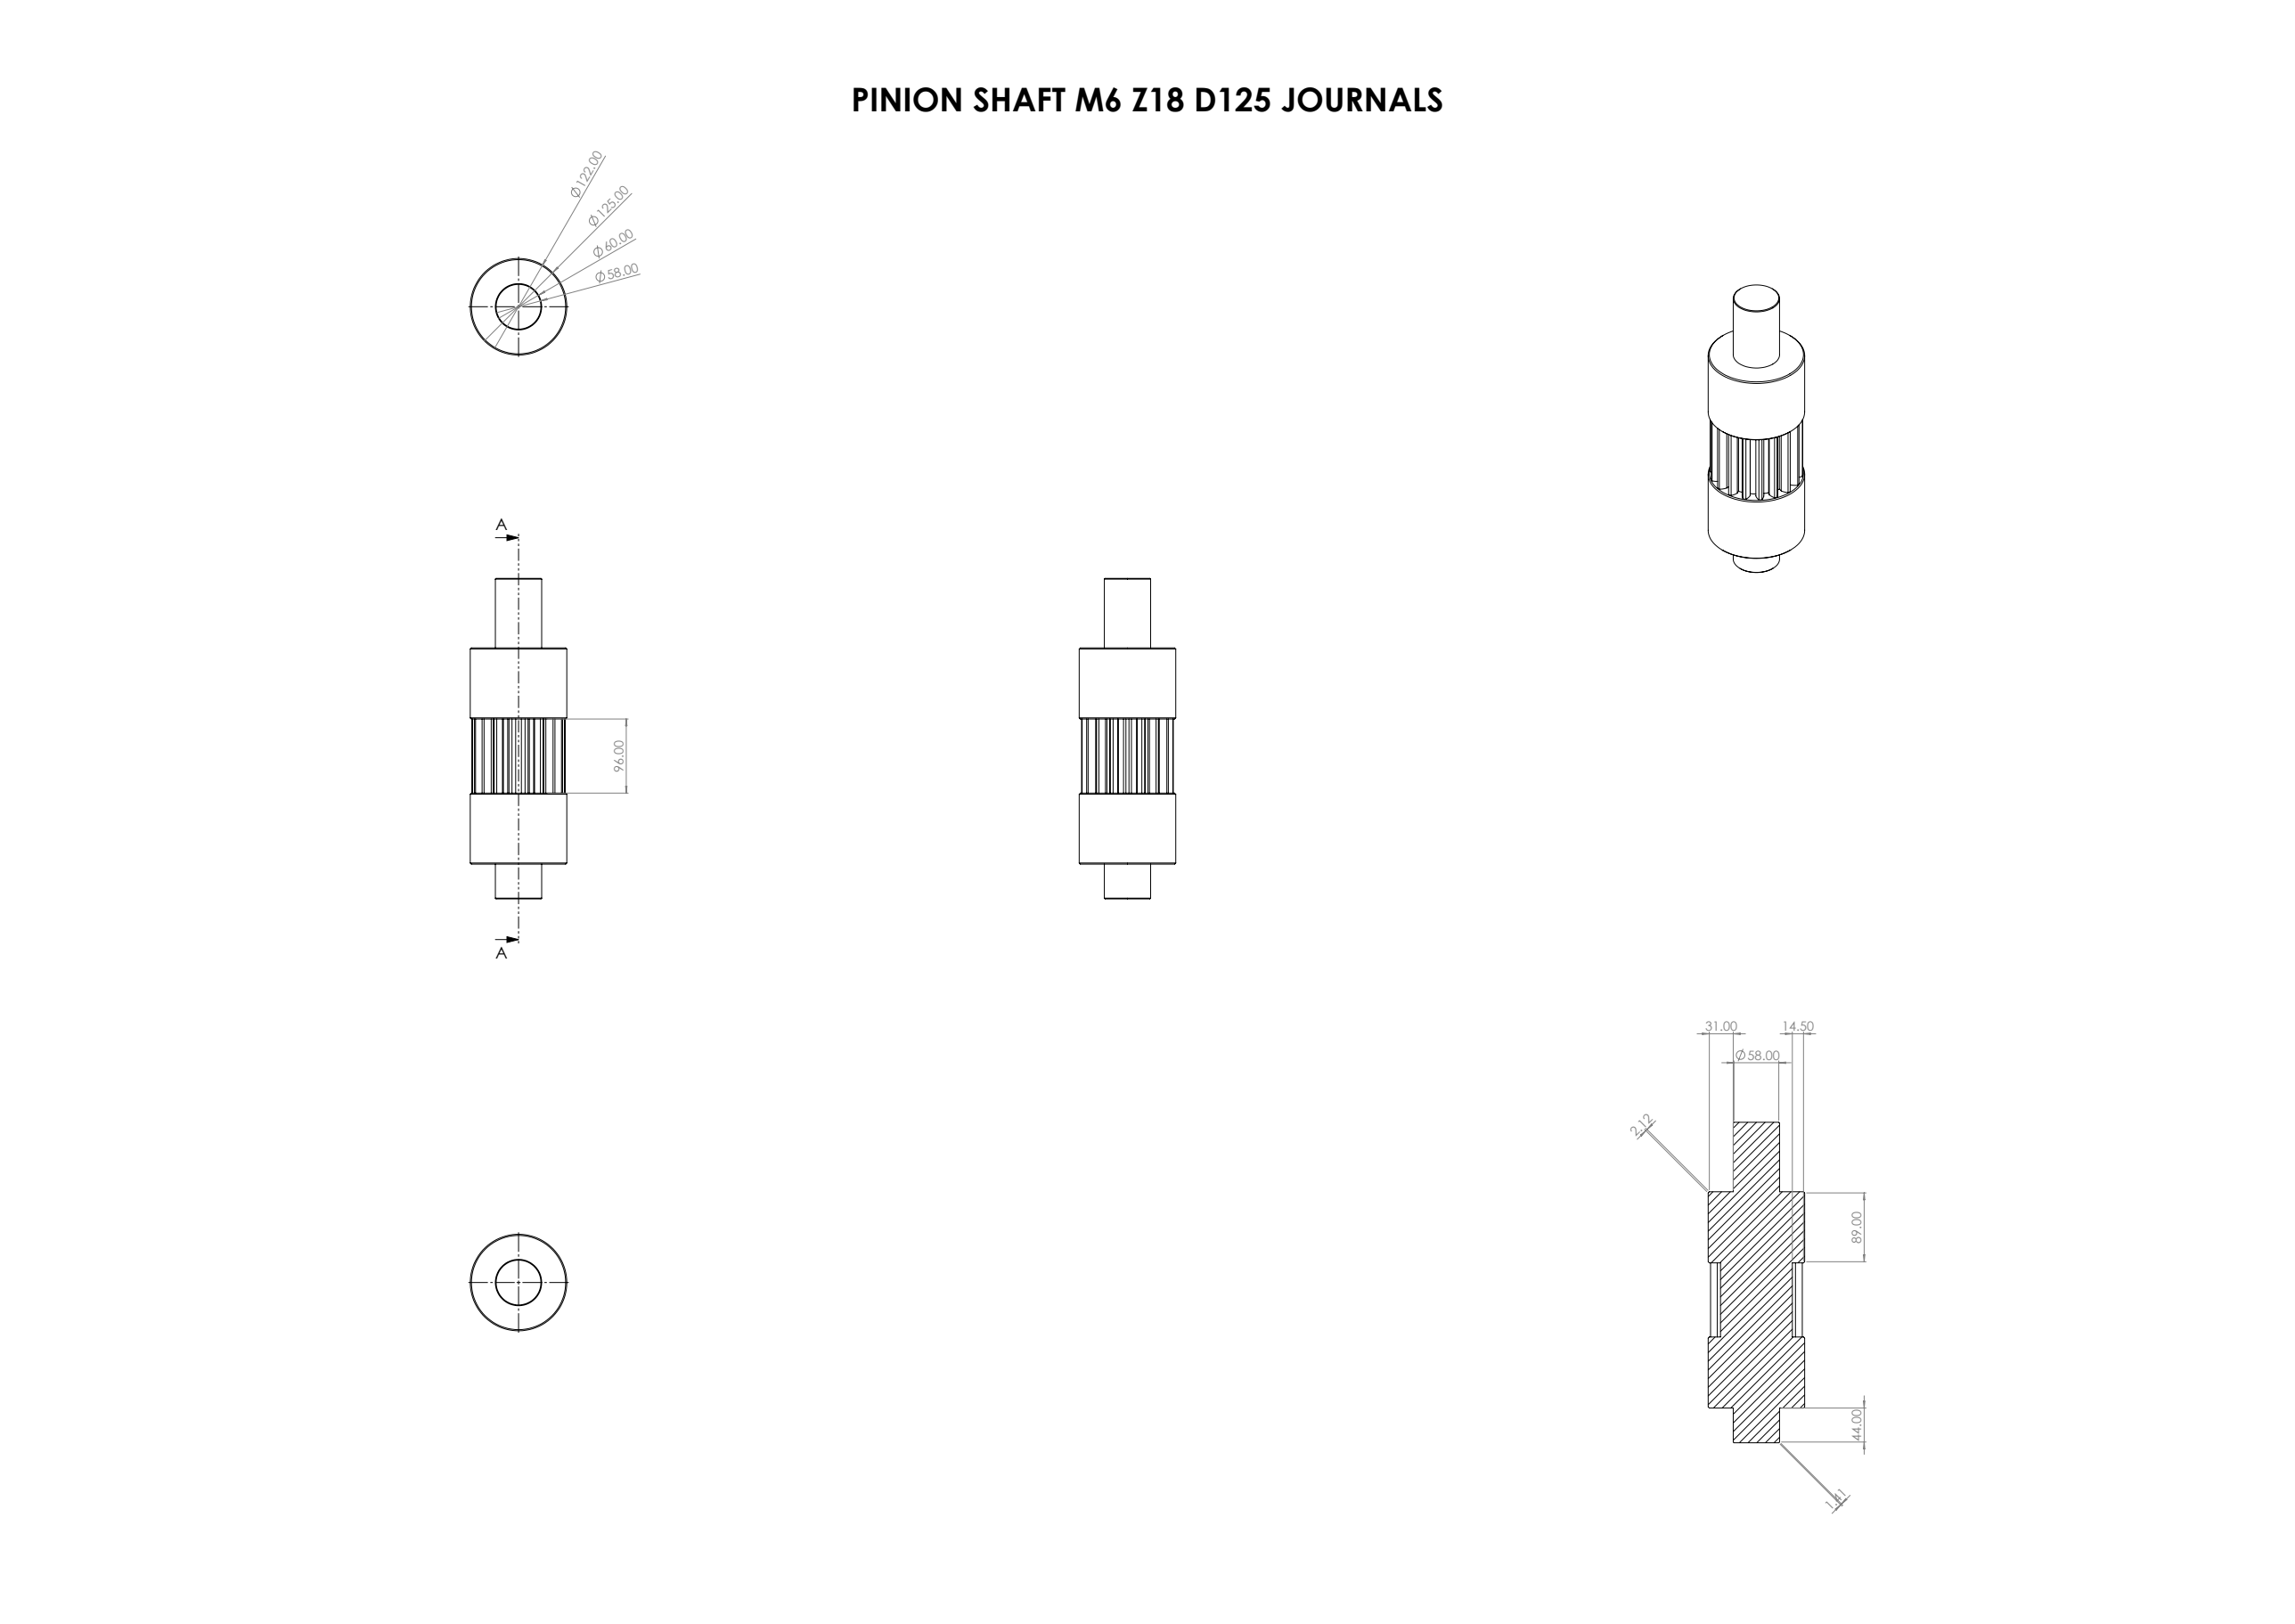
ISO-10303-21;
HEADER;
/* Generated by software containing ST-Developer
 * from STEP Tools, Inc. (www.steptools.com) 
 */

FILE_DESCRIPTION(
/* description */ (''),
/* implementation_level */ '2;1');

FILE_NAME(
/* name */ '03_Pinion_Shaft_m6_z18_D125_Journals.step',
/* time_stamp */ '2026-10-19T23:58:09-07:00',
/* author */ (''),
/* organization */ (''),
/* preprocessor_version */ 'ST-DEVELOPER v20.2',
/* originating_system */ 'Autodesk Translation Framework v15.15.0.0',
/* authorisation */ '');

FILE_SCHEMA (('AP203_CONFIGURATION_CONTROLLED_3D_DESIGN_OF_MECHANICAL_PARTS_AND_ASSEMBLIES_MIM_LF { 1 0 10303 203 3 1 4 }',
'AUTOMOTIVE_DESIGN { 1 0 10303 214 3 1 1 }','INTEGRATED_CNC_SCHEMA','MODEL_BASED_INTEGRATED_MANUFACTURING_SCHEMA',
'PROCESS_PLANNING_SCHEMA','AP242_MANAGED_MODEL_BASED_3D_ENGINEERING_MIM_LF { 1 0 10303 442 3 1 4 }'));
ENDSEC;

DATA;
#10=MECHANICAL_DESIGN_GEOMETRIC_PRESENTATION_REPRESENTATION('',(#407),#70757);
#377=SHAPE_REPRESENTATION_RELATIONSHIP('SRR','None',#70818,#392);
#392=ADVANCED_BREP_SHAPE_REPRESENTATION('',(#467),#70742);
#407=STYLED_ITEM('',(#71047),#467);
#467=MANIFOLD_SOLID_BREP('Pinion shaft',#26872);
#482=(
BOUNDED_SURFACE()
B_SPLINE_SURFACE(5,1,((#37442,#37443),(#37444,#37445),(#37446,#37447),(#37448,
#37449),(#37450,#37451),(#37452,#37453),(#37454,#37455),(#37456,#37457),
(#37458,#37459),(#37460,#37461),(#37462,#37463),(#37464,#37465),(#37466,
#37467),(#37468,#37469),(#37470,#37471),(#37472,#37473),(#37474,#37475),
(#37476,#37477),(#37478,#37479),(#37480,#37481),(#37482,#37483),(#37484,
#37485),(#37486,#37487),(#37488,#37489),(#37490,#37491),(#37492,#37493),
(#37494,#37495),(#37496,#37497),(#37498,#37499),(#37500,#37501),(#37502,
#37503),(#37504,#37505),(#37506,#37507),(#37508,#37509),(#37510,#37511)),
 .UNSPECIFIED.,.F.,.F.,.F.)
B_SPLINE_SURFACE_WITH_KNOTS((6,1,1,1,1,1,1,1,1,1,1,1,1,1,1,1,1,1,1,1,1,
1,1,1,1,1,1,1,1,1,6),(2,2),(-1.,-0.966666666666667,-0.933333333333333,-0.9,
-0.866666666666667,-0.833333333333333,-0.8,-0.766666666666667,-0.733333333333333,
-0.7,-0.666666666666667,-0.633333333333333,-0.6,-0.566666666666667,-0.533333333333333,
-0.5,-0.466666666666667,-0.433333333333333,-0.4,-0.366666666666667,-0.333333333333333,
-0.3,-0.266666666666667,-0.233333333333333,-0.2,-0.166666666666667,-0.133333333333333,
-0.1,-0.0666666666666667,-0.0333333333333333,0.),(-5.,5.),.UNSPECIFIED.)
GEOMETRIC_REPRESENTATION_ITEM()
RATIONAL_B_SPLINE_SURFACE(((1.,1.),(1.,1.),(1.,1.),(1.,1.),(1.,1.),(1.,
1.),(1.,1.),(1.,1.),(1.,1.),(1.,1.),(1.,1.),(1.,1.),(1.,1.),(1.,1.),(1.,
1.),(1.,1.),(1.,1.),(1.,1.),(1.,1.),(1.,1.),(1.,1.),(1.,1.),(1.,1.),(1.,
1.),(1.,1.),(1.,1.),(1.,1.),(1.,1.),(1.,1.),(1.,1.),(1.,1.),(1.,1.),(1.,
1.),(1.,1.),(1.,1.)))
REPRESENTATION_ITEM('')
SURFACE()
);
#483=(
BOUNDED_SURFACE()
B_SPLINE_SURFACE(5,1,((#37523,#37524),(#37525,#37526),(#37527,#37528),(#37529,
#37530),(#37531,#37532),(#37533,#37534),(#37535,#37536),(#37537,#37538),
(#37539,#37540),(#37541,#37542),(#37543,#37544),(#37545,#37546),(#37547,
#37548),(#37549,#37550),(#37551,#37552),(#37553,#37554),(#37555,#37556),
(#37557,#37558),(#37559,#37560),(#37561,#37562),(#37563,#37564),(#37565,
#37566),(#37567,#37568),(#37569,#37570),(#37571,#37572),(#37573,#37574),
(#37575,#37576),(#37577,#37578),(#37579,#37580),(#37581,#37582),(#37583,
#37584),(#37585,#37586),(#37587,#37588),(#37589,#37590),(#37591,#37592)),
 .UNSPECIFIED.,.F.,.F.,.F.)
B_SPLINE_SURFACE_WITH_KNOTS((6,1,1,1,1,1,1,1,1,1,1,1,1,1,1,1,1,1,1,1,1,
1,1,1,1,1,1,1,1,1,6),(2,2),(0.,0.0333333333333333,0.0666666666666667,0.1,
0.133333333333333,0.166666666666667,0.2,0.233333333333333,0.266666666666667,
0.3,0.333333333333333,0.366666666666667,0.4,0.433333333333333,0.466666666666667,
0.5,0.533333333333333,0.566666666666667,0.6,0.633333333333333,0.666666666666667,
0.7,0.733333333333333,0.766666666666667,0.8,0.833333333333333,0.866666666666667,
0.9,0.933333333333333,0.966666666666667,1.),(-5.,5.),.UNSPECIFIED.)
GEOMETRIC_REPRESENTATION_ITEM()
RATIONAL_B_SPLINE_SURFACE(((1.,1.),(1.,1.),(1.,1.),(1.,1.),(1.,1.),(1.,
1.),(1.,1.),(1.,1.),(1.,1.),(1.,1.),(1.,1.),(1.,1.),(1.,1.),(1.,1.),(1.,
1.),(1.,1.),(1.,1.),(1.,1.),(1.,1.),(1.,1.),(1.,1.),(1.,1.),(1.,1.),(1.,
1.),(1.,1.),(1.,1.),(1.,1.),(1.,1.),(1.,1.),(1.,1.),(1.,1.),(1.,1.),(1.,
1.),(1.,1.),(1.,1.)))
REPRESENTATION_ITEM('')
SURFACE()
);
#484=(
BOUNDED_SURFACE()
B_SPLINE_SURFACE(5,1,((#37601,#37602),(#37603,#37604),(#37605,#37606),(#37607,
#37608),(#37609,#37610),(#37611,#37612),(#37613,#37614),(#37615,#37616),
(#37617,#37618),(#37619,#37620),(#37621,#37622),(#37623,#37624),(#37625,
#37626),(#37627,#37628),(#37629,#37630),(#37631,#37632),(#37633,#37634),
(#37635,#37636),(#37637,#37638),(#37639,#37640),(#37641,#37642),(#37643,
#37644),(#37645,#37646),(#37647,#37648),(#37649,#37650),(#37651,#37652),
(#37653,#37654),(#37655,#37656),(#37657,#37658),(#37659,#37660),(#37661,
#37662),(#37663,#37664),(#37665,#37666),(#37667,#37668),(#37669,#37670)),
 .UNSPECIFIED.,.F.,.F.,.F.)
B_SPLINE_SURFACE_WITH_KNOTS((6,1,1,1,1,1,1,1,1,1,1,1,1,1,1,1,1,1,1,1,1,
1,1,1,1,1,1,1,1,1,6),(2,2),(-1.,-0.966666666666667,-0.933333333333333,-0.9,
-0.866666666666667,-0.833333333333333,-0.8,-0.766666666666667,-0.733333333333333,
-0.7,-0.666666666666667,-0.633333333333333,-0.6,-0.566666666666667,-0.533333333333333,
-0.5,-0.466666666666667,-0.433333333333333,-0.4,-0.366666666666667,-0.333333333333333,
-0.3,-0.266666666666667,-0.233333333333333,-0.2,-0.166666666666667,-0.133333333333333,
-0.1,-0.0666666666666667,-0.0333333333333333,0.),(-5.,5.),.UNSPECIFIED.)
GEOMETRIC_REPRESENTATION_ITEM()
RATIONAL_B_SPLINE_SURFACE(((1.,1.),(1.,1.),(1.,1.),(1.,1.),(1.,1.),(1.,
1.),(1.,1.),(1.,1.),(1.,1.),(1.,1.),(1.,1.),(1.,1.),(1.,1.),(1.,1.),(1.,
1.),(1.,1.),(1.,1.),(1.,1.),(1.,1.),(1.,1.),(1.,1.),(1.,1.),(1.,1.),(1.,
1.),(1.,1.),(1.,1.),(1.,1.),(1.,1.),(1.,1.),(1.,1.),(1.,1.),(1.,1.),(1.,
1.),(1.,1.),(1.,1.)))
REPRESENTATION_ITEM('')
SURFACE()
);
#485=(
BOUNDED_SURFACE()
B_SPLINE_SURFACE(5,1,((#37682,#37683),(#37684,#37685),(#37686,#37687),(#37688,
#37689),(#37690,#37691),(#37692,#37693),(#37694,#37695),(#37696,#37697),
(#37698,#37699),(#37700,#37701),(#37702,#37703),(#37704,#37705),(#37706,
#37707),(#37708,#37709),(#37710,#37711),(#37712,#37713),(#37714,#37715),
(#37716,#37717),(#37718,#37719),(#37720,#37721),(#37722,#37723),(#37724,
#37725),(#37726,#37727),(#37728,#37729),(#37730,#37731),(#37732,#37733),
(#37734,#37735),(#37736,#37737),(#37738,#37739),(#37740,#37741),(#37742,
#37743),(#37744,#37745),(#37746,#37747),(#37748,#37749),(#37750,#37751)),
 .UNSPECIFIED.,.F.,.F.,.F.)
B_SPLINE_SURFACE_WITH_KNOTS((6,1,1,1,1,1,1,1,1,1,1,1,1,1,1,1,1,1,1,1,1,
1,1,1,1,1,1,1,1,1,6),(2,2),(0.,0.0333333333333333,0.0666666666666667,0.1,
0.133333333333333,0.166666666666667,0.2,0.233333333333333,0.266666666666667,
0.3,0.333333333333333,0.366666666666667,0.4,0.433333333333333,0.466666666666667,
0.5,0.533333333333333,0.566666666666667,0.6,0.633333333333333,0.666666666666667,
0.7,0.733333333333333,0.766666666666667,0.8,0.833333333333333,0.866666666666667,
0.9,0.933333333333333,0.966666666666667,1.),(-5.,5.),.UNSPECIFIED.)
GEOMETRIC_REPRESENTATION_ITEM()
RATIONAL_B_SPLINE_SURFACE(((1.,1.),(1.,1.),(1.,1.),(1.,1.),(1.,1.),(1.,
1.),(1.,1.),(1.,1.),(1.,1.),(1.,1.),(1.,1.),(1.,1.),(1.,1.),(1.,1.),(1.,
1.),(1.,1.),(1.,1.),(1.,1.),(1.,1.),(1.,1.),(1.,1.),(1.,1.),(1.,1.),(1.,
1.),(1.,1.),(1.,1.),(1.,1.),(1.,1.),(1.,1.),(1.,1.),(1.,1.),(1.,1.),(1.,
1.),(1.,1.),(1.,1.)))
REPRESENTATION_ITEM('')
SURFACE()
);
#486=(
BOUNDED_SURFACE()
B_SPLINE_SURFACE(5,1,((#37760,#37761),(#37762,#37763),(#37764,#37765),(#37766,
#37767),(#37768,#37769),(#37770,#37771),(#37772,#37773),(#37774,#37775),
(#37776,#37777),(#37778,#37779),(#37780,#37781),(#37782,#37783),(#37784,
#37785),(#37786,#37787),(#37788,#37789),(#37790,#37791),(#37792,#37793),
(#37794,#37795),(#37796,#37797),(#37798,#37799),(#37800,#37801),(#37802,
#37803),(#37804,#37805),(#37806,#37807),(#37808,#37809),(#37810,#37811),
(#37812,#37813),(#37814,#37815),(#37816,#37817),(#37818,#37819),(#37820,
#37821),(#37822,#37823),(#37824,#37825),(#37826,#37827),(#37828,#37829)),
 .UNSPECIFIED.,.F.,.F.,.F.)
B_SPLINE_SURFACE_WITH_KNOTS((6,1,1,1,1,1,1,1,1,1,1,1,1,1,1,1,1,1,1,1,1,
1,1,1,1,1,1,1,1,1,6),(2,2),(-1.,-0.966666666666667,-0.933333333333333,-0.9,
-0.866666666666667,-0.833333333333333,-0.8,-0.766666666666667,-0.733333333333333,
-0.7,-0.666666666666667,-0.633333333333333,-0.6,-0.566666666666667,-0.533333333333333,
-0.5,-0.466666666666667,-0.433333333333333,-0.4,-0.366666666666667,-0.333333333333333,
-0.3,-0.266666666666667,-0.233333333333333,-0.2,-0.166666666666667,-0.133333333333333,
-0.1,-0.0666666666666667,-0.0333333333333333,0.),(-5.,5.),.UNSPECIFIED.)
GEOMETRIC_REPRESENTATION_ITEM()
RATIONAL_B_SPLINE_SURFACE(((1.,1.),(1.,1.),(1.,1.),(1.,1.),(1.,1.),(1.,
1.),(1.,1.),(1.,1.),(1.,1.),(1.,1.),(1.,1.),(1.,1.),(1.,1.),(1.,1.),(1.,
1.),(1.,1.),(1.,1.),(1.,1.),(1.,1.),(1.,1.),(1.,1.),(1.,1.),(1.,1.),(1.,
1.),(1.,1.),(1.,1.),(1.,1.),(1.,1.),(1.,1.),(1.,1.),(1.,1.),(1.,1.),(1.,
1.),(1.,1.),(1.,1.)))
REPRESENTATION_ITEM('')
SURFACE()
);
#487=(
BOUNDED_SURFACE()
B_SPLINE_SURFACE(5,1,((#37841,#37842),(#37843,#37844),(#37845,#37846),(#37847,
#37848),(#37849,#37850),(#37851,#37852),(#37853,#37854),(#37855,#37856),
(#37857,#37858),(#37859,#37860),(#37861,#37862),(#37863,#37864),(#37865,
#37866),(#37867,#37868),(#37869,#37870),(#37871,#37872),(#37873,#37874),
(#37875,#37876),(#37877,#37878),(#37879,#37880),(#37881,#37882),(#37883,
#37884),(#37885,#37886),(#37887,#37888),(#37889,#37890),(#37891,#37892),
(#37893,#37894),(#37895,#37896),(#37897,#37898),(#37899,#37900),(#37901,
#37902),(#37903,#37904),(#37905,#37906),(#37907,#37908),(#37909,#37910)),
 .UNSPECIFIED.,.F.,.F.,.F.)
B_SPLINE_SURFACE_WITH_KNOTS((6,1,1,1,1,1,1,1,1,1,1,1,1,1,1,1,1,1,1,1,1,
1,1,1,1,1,1,1,1,1,6),(2,2),(0.,0.0333333333333333,0.0666666666666667,0.1,
0.133333333333333,0.166666666666667,0.2,0.233333333333333,0.266666666666667,
0.3,0.333333333333333,0.366666666666667,0.4,0.433333333333333,0.466666666666667,
0.5,0.533333333333333,0.566666666666667,0.6,0.633333333333333,0.666666666666667,
0.7,0.733333333333333,0.766666666666667,0.8,0.833333333333333,0.866666666666667,
0.9,0.933333333333333,0.966666666666667,1.),(-5.,5.),.UNSPECIFIED.)
GEOMETRIC_REPRESENTATION_ITEM()
RATIONAL_B_SPLINE_SURFACE(((1.,1.),(1.,1.),(1.,1.),(1.,1.),(1.,1.),(1.,
1.),(1.,1.),(1.,1.),(1.,1.),(1.,1.),(1.,1.),(1.,1.),(1.,1.),(1.,1.),(1.,
1.),(1.,1.),(1.,1.),(1.,1.),(1.,1.),(1.,1.),(1.,1.),(1.,1.),(1.,1.),(1.,
1.),(1.,1.),(1.,1.),(1.,1.),(1.,1.),(1.,1.),(1.,1.),(1.,1.),(1.,1.),(1.,
1.),(1.,1.),(1.,1.)))
REPRESENTATION_ITEM('')
SURFACE()
);
#488=(
BOUNDED_SURFACE()
B_SPLINE_SURFACE(5,1,((#37919,#37920),(#37921,#37922),(#37923,#37924),(#37925,
#37926),(#37927,#37928),(#37929,#37930),(#37931,#37932),(#37933,#37934),
(#37935,#37936),(#37937,#37938),(#37939,#37940),(#37941,#37942),(#37943,
#37944),(#37945,#37946),(#37947,#37948),(#37949,#37950),(#37951,#37952),
(#37953,#37954),(#37955,#37956),(#37957,#37958),(#37959,#37960),(#37961,
#37962),(#37963,#37964),(#37965,#37966),(#37967,#37968),(#37969,#37970),
(#37971,#37972),(#37973,#37974),(#37975,#37976),(#37977,#37978),(#37979,
#37980),(#37981,#37982),(#37983,#37984),(#37985,#37986),(#37987,#37988)),
 .UNSPECIFIED.,.F.,.F.,.F.)
B_SPLINE_SURFACE_WITH_KNOTS((6,1,1,1,1,1,1,1,1,1,1,1,1,1,1,1,1,1,1,1,1,
1,1,1,1,1,1,1,1,1,6),(2,2),(-1.,-0.966666666666667,-0.933333333333333,-0.9,
-0.866666666666667,-0.833333333333333,-0.8,-0.766666666666667,-0.733333333333333,
-0.7,-0.666666666666667,-0.633333333333333,-0.6,-0.566666666666667,-0.533333333333333,
-0.5,-0.466666666666667,-0.433333333333333,-0.4,-0.366666666666667,-0.333333333333333,
-0.3,-0.266666666666667,-0.233333333333333,-0.2,-0.166666666666667,-0.133333333333333,
-0.1,-0.0666666666666667,-0.0333333333333333,0.),(-5.,5.),.UNSPECIFIED.)
GEOMETRIC_REPRESENTATION_ITEM()
RATIONAL_B_SPLINE_SURFACE(((1.,1.),(1.,1.),(1.,1.),(1.,1.),(1.,1.),(1.,
1.),(1.,1.),(1.,1.),(1.,1.),(1.,1.),(1.,1.),(1.,1.),(1.,1.),(1.,1.),(1.,
1.),(1.,1.),(1.,1.),(1.,1.),(1.,1.),(1.,1.),(1.,1.),(1.,1.),(1.,1.),(1.,
1.),(1.,1.),(1.,1.),(1.,1.),(1.,1.),(1.,1.),(1.,1.),(1.,1.),(1.,1.),(1.,
1.),(1.,1.),(1.,1.)))
REPRESENTATION_ITEM('')
SURFACE()
);
#489=(
BOUNDED_SURFACE()
B_SPLINE_SURFACE(5,1,((#38000,#38001),(#38002,#38003),(#38004,#38005),(#38006,
#38007),(#38008,#38009),(#38010,#38011),(#38012,#38013),(#38014,#38015),
(#38016,#38017),(#38018,#38019),(#38020,#38021),(#38022,#38023),(#38024,
#38025),(#38026,#38027),(#38028,#38029),(#38030,#38031),(#38032,#38033),
(#38034,#38035),(#38036,#38037),(#38038,#38039),(#38040,#38041),(#38042,
#38043),(#38044,#38045),(#38046,#38047),(#38048,#38049),(#38050,#38051),
(#38052,#38053),(#38054,#38055),(#38056,#38057),(#38058,#38059),(#38060,
#38061),(#38062,#38063),(#38064,#38065),(#38066,#38067),(#38068,#38069)),
 .UNSPECIFIED.,.F.,.F.,.F.)
B_SPLINE_SURFACE_WITH_KNOTS((6,1,1,1,1,1,1,1,1,1,1,1,1,1,1,1,1,1,1,1,1,
1,1,1,1,1,1,1,1,1,6),(2,2),(0.,0.0333333333333333,0.0666666666666667,0.1,
0.133333333333333,0.166666666666667,0.2,0.233333333333333,0.266666666666667,
0.3,0.333333333333333,0.366666666666667,0.4,0.433333333333333,0.466666666666667,
0.5,0.533333333333333,0.566666666666667,0.6,0.633333333333333,0.666666666666667,
0.7,0.733333333333333,0.766666666666667,0.8,0.833333333333333,0.866666666666667,
0.9,0.933333333333333,0.966666666666667,1.),(-5.,5.),.UNSPECIFIED.)
GEOMETRIC_REPRESENTATION_ITEM()
RATIONAL_B_SPLINE_SURFACE(((1.,1.),(1.,1.),(1.,1.),(1.,1.),(1.,1.),(1.,
1.),(1.,1.),(1.,1.),(1.,1.),(1.,1.),(1.,1.),(1.,1.),(1.,1.),(1.,1.),(1.,
1.),(1.,1.),(1.,1.),(1.,1.),(1.,1.),(1.,1.),(1.,1.),(1.,1.),(1.,1.),(1.,
1.),(1.,1.),(1.,1.),(1.,1.),(1.,1.),(1.,1.),(1.,1.),(1.,1.),(1.,1.),(1.,
1.),(1.,1.),(1.,1.)))
REPRESENTATION_ITEM('')
SURFACE()
);
#490=(
BOUNDED_SURFACE()
B_SPLINE_SURFACE(5,1,((#38078,#38079),(#38080,#38081),(#38082,#38083),(#38084,
#38085),(#38086,#38087),(#38088,#38089),(#38090,#38091),(#38092,#38093),
(#38094,#38095),(#38096,#38097),(#38098,#38099),(#38100,#38101),(#38102,
#38103),(#38104,#38105),(#38106,#38107),(#38108,#38109),(#38110,#38111),
(#38112,#38113),(#38114,#38115),(#38116,#38117),(#38118,#38119),(#38120,
#38121),(#38122,#38123),(#38124,#38125),(#38126,#38127),(#38128,#38129),
(#38130,#38131),(#38132,#38133),(#38134,#38135),(#38136,#38137),(#38138,
#38139),(#38140,#38141),(#38142,#38143),(#38144,#38145),(#38146,#38147)),
 .UNSPECIFIED.,.F.,.F.,.F.)
B_SPLINE_SURFACE_WITH_KNOTS((6,1,1,1,1,1,1,1,1,1,1,1,1,1,1,1,1,1,1,1,1,
1,1,1,1,1,1,1,1,1,6),(2,2),(-1.,-0.966666666666667,-0.933333333333333,-0.9,
-0.866666666666667,-0.833333333333333,-0.8,-0.766666666666667,-0.733333333333333,
-0.7,-0.666666666666667,-0.633333333333333,-0.6,-0.566666666666667,-0.533333333333333,
-0.5,-0.466666666666667,-0.433333333333333,-0.4,-0.366666666666667,-0.333333333333333,
-0.3,-0.266666666666667,-0.233333333333333,-0.2,-0.166666666666667,-0.133333333333333,
-0.1,-0.0666666666666667,-0.0333333333333333,0.),(-5.,5.),.UNSPECIFIED.)
GEOMETRIC_REPRESENTATION_ITEM()
RATIONAL_B_SPLINE_SURFACE(((1.,1.),(1.,1.),(1.,1.),(1.,1.),(1.,1.),(1.,
1.),(1.,1.),(1.,1.),(1.,1.),(1.,1.),(1.,1.),(1.,1.),(1.,1.),(1.,1.),(1.,
1.),(1.,1.),(1.,1.),(1.,1.),(1.,1.),(1.,1.),(1.,1.),(1.,1.),(1.,1.),(1.,
1.),(1.,1.),(1.,1.),(1.,1.),(1.,1.),(1.,1.),(1.,1.),(1.,1.),(1.,1.),(1.,
1.),(1.,1.),(1.,1.)))
REPRESENTATION_ITEM('')
SURFACE()
);
#491=(
BOUNDED_SURFACE()
B_SPLINE_SURFACE(5,1,((#38159,#38160),(#38161,#38162),(#38163,#38164),(#38165,
#38166),(#38167,#38168),(#38169,#38170),(#38171,#38172),(#38173,#38174),
(#38175,#38176),(#38177,#38178),(#38179,#38180),(#38181,#38182),(#38183,
#38184),(#38185,#38186),(#38187,#38188),(#38189,#38190),(#38191,#38192),
(#38193,#38194),(#38195,#38196),(#38197,#38198),(#38199,#38200),(#38201,
#38202),(#38203,#38204),(#38205,#38206),(#38207,#38208),(#38209,#38210),
(#38211,#38212),(#38213,#38214),(#38215,#38216),(#38217,#38218),(#38219,
#38220),(#38221,#38222),(#38223,#38224),(#38225,#38226),(#38227,#38228)),
 .UNSPECIFIED.,.F.,.F.,.F.)
B_SPLINE_SURFACE_WITH_KNOTS((6,1,1,1,1,1,1,1,1,1,1,1,1,1,1,1,1,1,1,1,1,
1,1,1,1,1,1,1,1,1,6),(2,2),(0.,0.0333333333333333,0.0666666666666667,0.1,
0.133333333333333,0.166666666666667,0.2,0.233333333333333,0.266666666666667,
0.3,0.333333333333333,0.366666666666667,0.4,0.433333333333333,0.466666666666667,
0.5,0.533333333333333,0.566666666666667,0.6,0.633333333333333,0.666666666666667,
0.7,0.733333333333333,0.766666666666667,0.8,0.833333333333333,0.866666666666667,
0.9,0.933333333333333,0.966666666666667,1.),(-5.,5.),.UNSPECIFIED.)
GEOMETRIC_REPRESENTATION_ITEM()
RATIONAL_B_SPLINE_SURFACE(((1.,1.),(1.,1.),(1.,1.),(1.,1.),(1.,1.),(1.,
1.),(1.,1.),(1.,1.),(1.,1.),(1.,1.),(1.,1.),(1.,1.),(1.,1.),(1.,1.),(1.,
1.),(1.,1.),(1.,1.),(1.,1.),(1.,1.),(1.,1.),(1.,1.),(1.,1.),(1.,1.),(1.,
1.),(1.,1.),(1.,1.),(1.,1.),(1.,1.),(1.,1.),(1.,1.),(1.,1.),(1.,1.),(1.,
1.),(1.,1.),(1.,1.)))
REPRESENTATION_ITEM('')
SURFACE()
);
#492=(
BOUNDED_SURFACE()
B_SPLINE_SURFACE(5,1,((#38237,#38238),(#38239,#38240),(#38241,#38242),(#38243,
#38244),(#38245,#38246),(#38247,#38248),(#38249,#38250),(#38251,#38252),
(#38253,#38254),(#38255,#38256),(#38257,#38258),(#38259,#38260),(#38261,
#38262),(#38263,#38264),(#38265,#38266),(#38267,#38268),(#38269,#38270),
(#38271,#38272),(#38273,#38274),(#38275,#38276),(#38277,#38278),(#38279,
#38280),(#38281,#38282),(#38283,#38284),(#38285,#38286),(#38287,#38288),
(#38289,#38290),(#38291,#38292),(#38293,#38294),(#38295,#38296),(#38297,
#38298),(#38299,#38300),(#38301,#38302),(#38303,#38304),(#38305,#38306)),
 .UNSPECIFIED.,.F.,.F.,.F.)
B_SPLINE_SURFACE_WITH_KNOTS((6,1,1,1,1,1,1,1,1,1,1,1,1,1,1,1,1,1,1,1,1,
1,1,1,1,1,1,1,1,1,6),(2,2),(-1.,-0.966666666666667,-0.933333333333333,-0.9,
-0.866666666666667,-0.833333333333333,-0.8,-0.766666666666667,-0.733333333333333,
-0.7,-0.666666666666667,-0.633333333333333,-0.6,-0.566666666666667,-0.533333333333333,
-0.5,-0.466666666666667,-0.433333333333333,-0.4,-0.366666666666667,-0.333333333333333,
-0.3,-0.266666666666667,-0.233333333333333,-0.2,-0.166666666666667,-0.133333333333333,
-0.1,-0.0666666666666667,-0.0333333333333333,0.),(-5.,5.),.UNSPECIFIED.)
GEOMETRIC_REPRESENTATION_ITEM()
RATIONAL_B_SPLINE_SURFACE(((1.,1.),(1.,1.),(1.,1.),(1.,1.),(1.,1.),(1.,
1.),(1.,1.),(1.,1.),(1.,1.),(1.,1.),(1.,1.),(1.,1.),(1.,1.),(1.,1.),(1.,
1.),(1.,1.),(1.,1.),(1.,1.),(1.,1.),(1.,1.),(1.,1.),(1.,1.),(1.,1.),(1.,
1.),(1.,1.),(1.,1.),(1.,1.),(1.,1.),(1.,1.),(1.,1.),(1.,1.),(1.,1.),(1.,
1.),(1.,1.),(1.,1.)))
REPRESENTATION_ITEM('')
SURFACE()
);
#493=(
BOUNDED_SURFACE()
B_SPLINE_SURFACE(5,1,((#38318,#38319),(#38320,#38321),(#38322,#38323),(#38324,
#38325),(#38326,#38327),(#38328,#38329),(#38330,#38331),(#38332,#38333),
(#38334,#38335),(#38336,#38337),(#38338,#38339),(#38340,#38341),(#38342,
#38343),(#38344,#38345),(#38346,#38347),(#38348,#38349),(#38350,#38351),
(#38352,#38353),(#38354,#38355),(#38356,#38357),(#38358,#38359),(#38360,
#38361),(#38362,#38363),(#38364,#38365),(#38366,#38367),(#38368,#38369),
(#38370,#38371),(#38372,#38373),(#38374,#38375),(#38376,#38377),(#38378,
#38379),(#38380,#38381),(#38382,#38383),(#38384,#38385),(#38386,#38387)),
 .UNSPECIFIED.,.F.,.F.,.F.)
B_SPLINE_SURFACE_WITH_KNOTS((6,1,1,1,1,1,1,1,1,1,1,1,1,1,1,1,1,1,1,1,1,
1,1,1,1,1,1,1,1,1,6),(2,2),(0.,0.0333333333333333,0.0666666666666667,0.1,
0.133333333333333,0.166666666666667,0.2,0.233333333333333,0.266666666666667,
0.3,0.333333333333333,0.366666666666667,0.4,0.433333333333333,0.466666666666667,
0.5,0.533333333333333,0.566666666666667,0.6,0.633333333333333,0.666666666666667,
0.7,0.733333333333333,0.766666666666667,0.8,0.833333333333333,0.866666666666667,
0.9,0.933333333333333,0.966666666666667,1.),(-5.,5.),.UNSPECIFIED.)
GEOMETRIC_REPRESENTATION_ITEM()
RATIONAL_B_SPLINE_SURFACE(((1.,1.),(1.,1.),(1.,1.),(1.,1.),(1.,1.),(1.,
1.),(1.,1.),(1.,1.),(1.,1.),(1.,1.),(1.,1.),(1.,1.),(1.,1.),(1.,1.),(1.,
1.),(1.,1.),(1.,1.),(1.,1.),(1.,1.),(1.,1.),(1.,1.),(1.,1.),(1.,1.),(1.,
1.),(1.,1.),(1.,1.),(1.,1.),(1.,1.),(1.,1.),(1.,1.),(1.,1.),(1.,1.),(1.,
1.),(1.,1.),(1.,1.)))
REPRESENTATION_ITEM('')
SURFACE()
);
#494=(
BOUNDED_SURFACE()
B_SPLINE_SURFACE(5,1,((#38396,#38397),(#38398,#38399),(#38400,#38401),(#38402,
#38403),(#38404,#38405),(#38406,#38407),(#38408,#38409),(#38410,#38411),
(#38412,#38413),(#38414,#38415),(#38416,#38417),(#38418,#38419),(#38420,
#38421),(#38422,#38423),(#38424,#38425),(#38426,#38427),(#38428,#38429),
(#38430,#38431),(#38432,#38433),(#38434,#38435),(#38436,#38437),(#38438,
#38439),(#38440,#38441),(#38442,#38443),(#38444,#38445),(#38446,#38447),
(#38448,#38449),(#38450,#38451),(#38452,#38453),(#38454,#38455),(#38456,
#38457),(#38458,#38459),(#38460,#38461),(#38462,#38463),(#38464,#38465)),
 .UNSPECIFIED.,.F.,.F.,.F.)
B_SPLINE_SURFACE_WITH_KNOTS((6,1,1,1,1,1,1,1,1,1,1,1,1,1,1,1,1,1,1,1,1,
1,1,1,1,1,1,1,1,1,6),(2,2),(-1.,-0.966666666666667,-0.933333333333333,-0.9,
-0.866666666666667,-0.833333333333333,-0.8,-0.766666666666667,-0.733333333333333,
-0.7,-0.666666666666667,-0.633333333333333,-0.6,-0.566666666666667,-0.533333333333333,
-0.5,-0.466666666666667,-0.433333333333333,-0.4,-0.366666666666667,-0.333333333333333,
-0.3,-0.266666666666667,-0.233333333333333,-0.2,-0.166666666666667,-0.133333333333333,
-0.1,-0.0666666666666667,-0.0333333333333333,0.),(-5.,5.),.UNSPECIFIED.)
GEOMETRIC_REPRESENTATION_ITEM()
RATIONAL_B_SPLINE_SURFACE(((1.,1.),(1.,1.),(1.,1.),(1.,1.),(1.,1.),(1.,
1.),(1.,1.),(1.,1.),(1.,1.),(1.,1.),(1.,1.),(1.,1.),(1.,1.),(1.,1.),(1.,
1.),(1.,1.),(1.,1.),(1.,1.),(1.,1.),(1.,1.),(1.,1.),(1.,1.),(1.,1.),(1.,
1.),(1.,1.),(1.,1.),(1.,1.),(1.,1.),(1.,1.),(1.,1.),(1.,1.),(1.,1.),(1.,
1.),(1.,1.),(1.,1.)))
REPRESENTATION_ITEM('')
SURFACE()
);
#495=(
BOUNDED_SURFACE()
B_SPLINE_SURFACE(5,1,((#38477,#38478),(#38479,#38480),(#38481,#38482),(#38483,
#38484),(#38485,#38486),(#38487,#38488),(#38489,#38490),(#38491,#38492),
(#38493,#38494),(#38495,#38496),(#38497,#38498),(#38499,#38500),(#38501,
#38502),(#38503,#38504),(#38505,#38506),(#38507,#38508),(#38509,#38510),
(#38511,#38512),(#38513,#38514),(#38515,#38516),(#38517,#38518),(#38519,
#38520),(#38521,#38522),(#38523,#38524),(#38525,#38526),(#38527,#38528),
(#38529,#38530),(#38531,#38532),(#38533,#38534),(#38535,#38536),(#38537,
#38538),(#38539,#38540),(#38541,#38542),(#38543,#38544),(#38545,#38546)),
 .UNSPECIFIED.,.F.,.F.,.F.)
B_SPLINE_SURFACE_WITH_KNOTS((6,1,1,1,1,1,1,1,1,1,1,1,1,1,1,1,1,1,1,1,1,
1,1,1,1,1,1,1,1,1,6),(2,2),(0.,0.0333333333333333,0.0666666666666667,0.1,
0.133333333333333,0.166666666666667,0.2,0.233333333333333,0.266666666666667,
0.3,0.333333333333333,0.366666666666667,0.4,0.433333333333333,0.466666666666667,
0.5,0.533333333333333,0.566666666666667,0.6,0.633333333333333,0.666666666666667,
0.7,0.733333333333333,0.766666666666667,0.8,0.833333333333333,0.866666666666667,
0.9,0.933333333333333,0.966666666666667,1.),(-5.,5.),.UNSPECIFIED.)
GEOMETRIC_REPRESENTATION_ITEM()
RATIONAL_B_SPLINE_SURFACE(((1.,1.),(1.,1.),(1.,1.),(1.,1.),(1.,1.),(1.,
1.),(1.,1.),(1.,1.),(1.,1.),(1.,1.),(1.,1.),(1.,1.),(1.,1.),(1.,1.),(1.,
1.),(1.,1.),(1.,1.),(1.,1.),(1.,1.),(1.,1.),(1.,1.),(1.,1.),(1.,1.),(1.,
1.),(1.,1.),(1.,1.),(1.,1.),(1.,1.),(1.,1.),(1.,1.),(1.,1.),(1.,1.),(1.,
1.),(1.,1.),(1.,1.)))
REPRESENTATION_ITEM('')
SURFACE()
);
#496=(
BOUNDED_SURFACE()
B_SPLINE_SURFACE(5,1,((#38555,#38556),(#38557,#38558),(#38559,#38560),(#38561,
#38562),(#38563,#38564),(#38565,#38566),(#38567,#38568),(#38569,#38570),
(#38571,#38572),(#38573,#38574),(#38575,#38576),(#38577,#38578),(#38579,
#38580),(#38581,#38582),(#38583,#38584),(#38585,#38586),(#38587,#38588),
(#38589,#38590),(#38591,#38592),(#38593,#38594),(#38595,#38596),(#38597,
#38598),(#38599,#38600),(#38601,#38602),(#38603,#38604),(#38605,#38606),
(#38607,#38608),(#38609,#38610),(#38611,#38612),(#38613,#38614),(#38615,
#38616),(#38617,#38618),(#38619,#38620),(#38621,#38622),(#38623,#38624)),
 .UNSPECIFIED.,.F.,.F.,.F.)
B_SPLINE_SURFACE_WITH_KNOTS((6,1,1,1,1,1,1,1,1,1,1,1,1,1,1,1,1,1,1,1,1,
1,1,1,1,1,1,1,1,1,6),(2,2),(-1.,-0.966666666666667,-0.933333333333333,-0.9,
-0.866666666666667,-0.833333333333333,-0.8,-0.766666666666667,-0.733333333333333,
-0.7,-0.666666666666667,-0.633333333333333,-0.6,-0.566666666666667,-0.533333333333333,
-0.5,-0.466666666666667,-0.433333333333333,-0.4,-0.366666666666667,-0.333333333333333,
-0.3,-0.266666666666667,-0.233333333333333,-0.2,-0.166666666666667,-0.133333333333333,
-0.1,-0.0666666666666667,-0.0333333333333333,0.),(-5.,5.),.UNSPECIFIED.)
GEOMETRIC_REPRESENTATION_ITEM()
RATIONAL_B_SPLINE_SURFACE(((1.,1.),(1.,1.),(1.,1.),(1.,1.),(1.,1.),(1.,
1.),(1.,1.),(1.,1.),(1.,1.),(1.,1.),(1.,1.),(1.,1.),(1.,1.),(1.,1.),(1.,
1.),(1.,1.),(1.,1.),(1.,1.),(1.,1.),(1.,1.),(1.,1.),(1.,1.),(1.,1.),(1.,
1.),(1.,1.),(1.,1.),(1.,1.),(1.,1.),(1.,1.),(1.,1.),(1.,1.),(1.,1.),(1.,
1.),(1.,1.),(1.,1.)))
REPRESENTATION_ITEM('')
SURFACE()
);
#497=(
BOUNDED_SURFACE()
B_SPLINE_SURFACE(5,1,((#38636,#38637),(#38638,#38639),(#38640,#38641),(#38642,
#38643),(#38644,#38645),(#38646,#38647),(#38648,#38649),(#38650,#38651),
(#38652,#38653),(#38654,#38655),(#38656,#38657),(#38658,#38659),(#38660,
#38661),(#38662,#38663),(#38664,#38665),(#38666,#38667),(#38668,#38669),
(#38670,#38671),(#38672,#38673),(#38674,#38675),(#38676,#38677),(#38678,
#38679),(#38680,#38681),(#38682,#38683),(#38684,#38685),(#38686,#38687),
(#38688,#38689),(#38690,#38691),(#38692,#38693),(#38694,#38695),(#38696,
#38697),(#38698,#38699),(#38700,#38701),(#38702,#38703),(#38704,#38705)),
 .UNSPECIFIED.,.F.,.F.,.F.)
B_SPLINE_SURFACE_WITH_KNOTS((6,1,1,1,1,1,1,1,1,1,1,1,1,1,1,1,1,1,1,1,1,
1,1,1,1,1,1,1,1,1,6),(2,2),(0.,0.0333333333333333,0.0666666666666667,0.1,
0.133333333333333,0.166666666666667,0.2,0.233333333333333,0.266666666666667,
0.3,0.333333333333333,0.366666666666667,0.4,0.433333333333333,0.466666666666667,
0.5,0.533333333333333,0.566666666666667,0.6,0.633333333333333,0.666666666666667,
0.7,0.733333333333333,0.766666666666667,0.8,0.833333333333333,0.866666666666667,
0.9,0.933333333333333,0.966666666666667,1.),(-5.,5.),.UNSPECIFIED.)
GEOMETRIC_REPRESENTATION_ITEM()
RATIONAL_B_SPLINE_SURFACE(((1.,1.),(1.,1.),(1.,1.),(1.,1.),(1.,1.),(1.,
1.),(1.,1.),(1.,1.),(1.,1.),(1.,1.),(1.,1.),(1.,1.),(1.,1.),(1.,1.),(1.,
1.),(1.,1.),(1.,1.),(1.,1.),(1.,1.),(1.,1.),(1.,1.),(1.,1.),(1.,1.),(1.,
1.),(1.,1.),(1.,1.),(1.,1.),(1.,1.),(1.,1.),(1.,1.),(1.,1.),(1.,1.),(1.,
1.),(1.,1.),(1.,1.)))
REPRESENTATION_ITEM('')
SURFACE()
);
#498=(
BOUNDED_SURFACE()
B_SPLINE_SURFACE(5,1,((#38714,#38715),(#38716,#38717),(#38718,#38719),(#38720,
#38721),(#38722,#38723),(#38724,#38725),(#38726,#38727),(#38728,#38729),
(#38730,#38731),(#38732,#38733),(#38734,#38735),(#38736,#38737),(#38738,
#38739),(#38740,#38741),(#38742,#38743),(#38744,#38745),(#38746,#38747),
(#38748,#38749),(#38750,#38751),(#38752,#38753),(#38754,#38755),(#38756,
#38757),(#38758,#38759),(#38760,#38761),(#38762,#38763),(#38764,#38765),
(#38766,#38767),(#38768,#38769),(#38770,#38771),(#38772,#38773),(#38774,
#38775),(#38776,#38777),(#38778,#38779),(#38780,#38781),(#38782,#38783)),
 .UNSPECIFIED.,.F.,.F.,.F.)
B_SPLINE_SURFACE_WITH_KNOTS((6,1,1,1,1,1,1,1,1,1,1,1,1,1,1,1,1,1,1,1,1,
1,1,1,1,1,1,1,1,1,6),(2,2),(-1.,-0.966666666666667,-0.933333333333333,-0.9,
-0.866666666666667,-0.833333333333333,-0.8,-0.766666666666667,-0.733333333333333,
-0.7,-0.666666666666667,-0.633333333333333,-0.6,-0.566666666666667,-0.533333333333333,
-0.5,-0.466666666666667,-0.433333333333333,-0.4,-0.366666666666667,-0.333333333333333,
-0.3,-0.266666666666667,-0.233333333333333,-0.2,-0.166666666666667,-0.133333333333333,
-0.1,-0.0666666666666667,-0.0333333333333333,0.),(-5.,5.),.UNSPECIFIED.)
GEOMETRIC_REPRESENTATION_ITEM()
RATIONAL_B_SPLINE_SURFACE(((1.,1.),(1.,1.),(1.,1.),(1.,1.),(1.,1.),(1.,
1.),(1.,1.),(1.,1.),(1.,1.),(1.,1.),(1.,1.),(1.,1.),(1.,1.),(1.,1.),(1.,
1.),(1.,1.),(1.,1.),(1.,1.),(1.,1.),(1.,1.),(1.,1.),(1.,1.),(1.,1.),(1.,
1.),(1.,1.),(1.,1.),(1.,1.),(1.,1.),(1.,1.),(1.,1.),(1.,1.),(1.,1.),(1.,
1.),(1.,1.),(1.,1.)))
REPRESENTATION_ITEM('')
SURFACE()
);
#499=(
BOUNDED_SURFACE()
B_SPLINE_SURFACE(5,1,((#38795,#38796),(#38797,#38798),(#38799,#38800),(#38801,
#38802),(#38803,#38804),(#38805,#38806),(#38807,#38808),(#38809,#38810),
(#38811,#38812),(#38813,#38814),(#38815,#38816),(#38817,#38818),(#38819,
#38820),(#38821,#38822),(#38823,#38824),(#38825,#38826),(#38827,#38828),
(#38829,#38830),(#38831,#38832),(#38833,#38834),(#38835,#38836),(#38837,
#38838),(#38839,#38840),(#38841,#38842),(#38843,#38844),(#38845,#38846),
(#38847,#38848),(#38849,#38850),(#38851,#38852),(#38853,#38854),(#38855,
#38856),(#38857,#38858),(#38859,#38860),(#38861,#38862),(#38863,#38864)),
 .UNSPECIFIED.,.F.,.F.,.F.)
B_SPLINE_SURFACE_WITH_KNOTS((6,1,1,1,1,1,1,1,1,1,1,1,1,1,1,1,1,1,1,1,1,
1,1,1,1,1,1,1,1,1,6),(2,2),(0.,0.0333333333333333,0.0666666666666667,0.1,
0.133333333333333,0.166666666666667,0.2,0.233333333333333,0.266666666666667,
0.3,0.333333333333333,0.366666666666667,0.4,0.433333333333333,0.466666666666667,
0.5,0.533333333333333,0.566666666666667,0.6,0.633333333333333,0.666666666666667,
0.7,0.733333333333333,0.766666666666667,0.8,0.833333333333333,0.866666666666667,
0.9,0.933333333333333,0.966666666666667,1.),(-5.,5.),.UNSPECIFIED.)
GEOMETRIC_REPRESENTATION_ITEM()
RATIONAL_B_SPLINE_SURFACE(((1.,1.),(1.,1.),(1.,1.),(1.,1.),(1.,1.),(1.,
1.),(1.,1.),(1.,1.),(1.,1.),(1.,1.),(1.,1.),(1.,1.),(1.,1.),(1.,1.),(1.,
1.),(1.,1.),(1.,1.),(1.,1.),(1.,1.),(1.,1.),(1.,1.),(1.,1.),(1.,1.),(1.,
1.),(1.,1.),(1.,1.),(1.,1.),(1.,1.),(1.,1.),(1.,1.),(1.,1.),(1.,1.),(1.,
1.),(1.,1.),(1.,1.)))
REPRESENTATION_ITEM('')
SURFACE()
);
#500=(
BOUNDED_SURFACE()
B_SPLINE_SURFACE(5,1,((#38873,#38874),(#38875,#38876),(#38877,#38878),(#38879,
#38880),(#38881,#38882),(#38883,#38884),(#38885,#38886),(#38887,#38888),
(#38889,#38890),(#38891,#38892),(#38893,#38894),(#38895,#38896),(#38897,
#38898),(#38899,#38900),(#38901,#38902),(#38903,#38904),(#38905,#38906),
(#38907,#38908),(#38909,#38910),(#38911,#38912),(#38913,#38914),(#38915,
#38916),(#38917,#38918),(#38919,#38920),(#38921,#38922),(#38923,#38924),
(#38925,#38926),(#38927,#38928),(#38929,#38930),(#38931,#38932),(#38933,
#38934),(#38935,#38936),(#38937,#38938),(#38939,#38940),(#38941,#38942)),
 .UNSPECIFIED.,.F.,.F.,.F.)
B_SPLINE_SURFACE_WITH_KNOTS((6,1,1,1,1,1,1,1,1,1,1,1,1,1,1,1,1,1,1,1,1,
1,1,1,1,1,1,1,1,1,6),(2,2),(-1.,-0.966666666666667,-0.933333333333333,-0.9,
-0.866666666666667,-0.833333333333333,-0.8,-0.766666666666667,-0.733333333333333,
-0.7,-0.666666666666667,-0.633333333333333,-0.6,-0.566666666666667,-0.533333333333333,
-0.5,-0.466666666666667,-0.433333333333333,-0.4,-0.366666666666667,-0.333333333333333,
-0.3,-0.266666666666667,-0.233333333333333,-0.2,-0.166666666666667,-0.133333333333333,
-0.1,-0.0666666666666667,-0.0333333333333333,0.),(-5.,5.),.UNSPECIFIED.)
GEOMETRIC_REPRESENTATION_ITEM()
RATIONAL_B_SPLINE_SURFACE(((1.,1.),(1.,1.),(1.,1.),(1.,1.),(1.,1.),(1.,
1.),(1.,1.),(1.,1.),(1.,1.),(1.,1.),(1.,1.),(1.,1.),(1.,1.),(1.,1.),(1.,
1.),(1.,1.),(1.,1.),(1.,1.),(1.,1.),(1.,1.),(1.,1.),(1.,1.),(1.,1.),(1.,
1.),(1.,1.),(1.,1.),(1.,1.),(1.,1.),(1.,1.),(1.,1.),(1.,1.),(1.,1.),(1.,
1.),(1.,1.),(1.,1.)))
REPRESENTATION_ITEM('')
SURFACE()
);
#501=(
BOUNDED_SURFACE()
B_SPLINE_SURFACE(5,1,((#38954,#38955),(#38956,#38957),(#38958,#38959),(#38960,
#38961),(#38962,#38963),(#38964,#38965),(#38966,#38967),(#38968,#38969),
(#38970,#38971),(#38972,#38973),(#38974,#38975),(#38976,#38977),(#38978,
#38979),(#38980,#38981),(#38982,#38983),(#38984,#38985),(#38986,#38987),
(#38988,#38989),(#38990,#38991),(#38992,#38993),(#38994,#38995),(#38996,
#38997),(#38998,#38999),(#39000,#39001),(#39002,#39003),(#39004,#39005),
(#39006,#39007),(#39008,#39009),(#39010,#39011),(#39012,#39013),(#39014,
#39015),(#39016,#39017),(#39018,#39019),(#39020,#39021),(#39022,#39023)),
 .UNSPECIFIED.,.F.,.F.,.F.)
B_SPLINE_SURFACE_WITH_KNOTS((6,1,1,1,1,1,1,1,1,1,1,1,1,1,1,1,1,1,1,1,1,
1,1,1,1,1,1,1,1,1,6),(2,2),(0.,0.0333333333333333,0.0666666666666667,0.1,
0.133333333333333,0.166666666666667,0.2,0.233333333333333,0.266666666666667,
0.3,0.333333333333333,0.366666666666667,0.4,0.433333333333333,0.466666666666667,
0.5,0.533333333333333,0.566666666666667,0.6,0.633333333333333,0.666666666666667,
0.7,0.733333333333333,0.766666666666667,0.8,0.833333333333333,0.866666666666667,
0.9,0.933333333333333,0.966666666666667,1.),(-5.,5.),.UNSPECIFIED.)
GEOMETRIC_REPRESENTATION_ITEM()
RATIONAL_B_SPLINE_SURFACE(((1.,1.),(1.,1.),(1.,1.),(1.,1.),(1.,1.),(1.,
1.),(1.,1.),(1.,1.),(1.,1.),(1.,1.),(1.,1.),(1.,1.),(1.,1.),(1.,1.),(1.,
1.),(1.,1.),(1.,1.),(1.,1.),(1.,1.),(1.,1.),(1.,1.),(1.,1.),(1.,1.),(1.,
1.),(1.,1.),(1.,1.),(1.,1.),(1.,1.),(1.,1.),(1.,1.),(1.,1.),(1.,1.),(1.,
1.),(1.,1.),(1.,1.)))
REPRESENTATION_ITEM('')
SURFACE()
);
#502=(
BOUNDED_SURFACE()
B_SPLINE_SURFACE(5,1,((#39032,#39033),(#39034,#39035),(#39036,#39037),(#39038,
#39039),(#39040,#39041),(#39042,#39043),(#39044,#39045),(#39046,#39047),
(#39048,#39049),(#39050,#39051),(#39052,#39053),(#39054,#39055),(#39056,
#39057),(#39058,#39059),(#39060,#39061),(#39062,#39063),(#39064,#39065),
(#39066,#39067),(#39068,#39069),(#39070,#39071),(#39072,#39073),(#39074,
#39075),(#39076,#39077),(#39078,#39079),(#39080,#39081),(#39082,#39083),
(#39084,#39085),(#39086,#39087),(#39088,#39089),(#39090,#39091),(#39092,
#39093),(#39094,#39095),(#39096,#39097),(#39098,#39099),(#39100,#39101)),
 .UNSPECIFIED.,.F.,.F.,.F.)
B_SPLINE_SURFACE_WITH_KNOTS((6,1,1,1,1,1,1,1,1,1,1,1,1,1,1,1,1,1,1,1,1,
1,1,1,1,1,1,1,1,1,6),(2,2),(-1.,-0.966666666666667,-0.933333333333333,-0.9,
-0.866666666666667,-0.833333333333333,-0.8,-0.766666666666667,-0.733333333333333,
-0.7,-0.666666666666667,-0.633333333333333,-0.6,-0.566666666666667,-0.533333333333333,
-0.5,-0.466666666666667,-0.433333333333333,-0.4,-0.366666666666667,-0.333333333333333,
-0.3,-0.266666666666667,-0.233333333333333,-0.2,-0.166666666666667,-0.133333333333333,
-0.1,-0.0666666666666667,-0.0333333333333333,0.),(-5.,5.),.UNSPECIFIED.)
GEOMETRIC_REPRESENTATION_ITEM()
RATIONAL_B_SPLINE_SURFACE(((1.,1.),(1.,1.),(1.,1.),(1.,1.),(1.,1.),(1.,
1.),(1.,1.),(1.,1.),(1.,1.),(1.,1.),(1.,1.),(1.,1.),(1.,1.),(1.,1.),(1.,
1.),(1.,1.),(1.,1.),(1.,1.),(1.,1.),(1.,1.),(1.,1.),(1.,1.),(1.,1.),(1.,
1.),(1.,1.),(1.,1.),(1.,1.),(1.,1.),(1.,1.),(1.,1.),(1.,1.),(1.,1.),(1.,
1.),(1.,1.),(1.,1.)))
REPRESENTATION_ITEM('')
SURFACE()
);
#503=(
BOUNDED_SURFACE()
B_SPLINE_SURFACE(5,1,((#39113,#39114),(#39115,#39116),(#39117,#39118),(#39119,
#39120),(#39121,#39122),(#39123,#39124),(#39125,#39126),(#39127,#39128),
(#39129,#39130),(#39131,#39132),(#39133,#39134),(#39135,#39136),(#39137,
#39138),(#39139,#39140),(#39141,#39142),(#39143,#39144),(#39145,#39146),
(#39147,#39148),(#39149,#39150),(#39151,#39152),(#39153,#39154),(#39155,
#39156),(#39157,#39158),(#39159,#39160),(#39161,#39162),(#39163,#39164),
(#39165,#39166),(#39167,#39168),(#39169,#39170),(#39171,#39172),(#39173,
#39174),(#39175,#39176),(#39177,#39178),(#39179,#39180),(#39181,#39182)),
 .UNSPECIFIED.,.F.,.F.,.F.)
B_SPLINE_SURFACE_WITH_KNOTS((6,1,1,1,1,1,1,1,1,1,1,1,1,1,1,1,1,1,1,1,1,
1,1,1,1,1,1,1,1,1,6),(2,2),(0.,0.0333333333333333,0.0666666666666667,0.1,
0.133333333333333,0.166666666666667,0.2,0.233333333333333,0.266666666666667,
0.3,0.333333333333333,0.366666666666667,0.4,0.433333333333333,0.466666666666667,
0.5,0.533333333333333,0.566666666666667,0.6,0.633333333333333,0.666666666666667,
0.7,0.733333333333333,0.766666666666667,0.8,0.833333333333333,0.866666666666667,
0.9,0.933333333333333,0.966666666666667,1.),(-5.,5.),.UNSPECIFIED.)
GEOMETRIC_REPRESENTATION_ITEM()
RATIONAL_B_SPLINE_SURFACE(((1.,1.),(1.,1.),(1.,1.),(1.,1.),(1.,1.),(1.,
1.),(1.,1.),(1.,1.),(1.,1.),(1.,1.),(1.,1.),(1.,1.),(1.,1.),(1.,1.),(1.,
1.),(1.,1.),(1.,1.),(1.,1.),(1.,1.),(1.,1.),(1.,1.),(1.,1.),(1.,1.),(1.,
1.),(1.,1.),(1.,1.),(1.,1.),(1.,1.),(1.,1.),(1.,1.),(1.,1.),(1.,1.),(1.,
1.),(1.,1.),(1.,1.)))
REPRESENTATION_ITEM('')
SURFACE()
);
#504=(
BOUNDED_SURFACE()
B_SPLINE_SURFACE(5,1,((#39191,#39192),(#39193,#39194),(#39195,#39196),(#39197,
#39198),(#39199,#39200),(#39201,#39202),(#39203,#39204),(#39205,#39206),
(#39207,#39208),(#39209,#39210),(#39211,#39212),(#39213,#39214),(#39215,
#39216),(#39217,#39218),(#39219,#39220),(#39221,#39222),(#39223,#39224),
(#39225,#39226),(#39227,#39228),(#39229,#39230),(#39231,#39232),(#39233,
#39234),(#39235,#39236),(#39237,#39238),(#39239,#39240),(#39241,#39242),
(#39243,#39244),(#39245,#39246),(#39247,#39248),(#39249,#39250),(#39251,
#39252),(#39253,#39254),(#39255,#39256),(#39257,#39258),(#39259,#39260)),
 .UNSPECIFIED.,.F.,.F.,.F.)
B_SPLINE_SURFACE_WITH_KNOTS((6,1,1,1,1,1,1,1,1,1,1,1,1,1,1,1,1,1,1,1,1,
1,1,1,1,1,1,1,1,1,6),(2,2),(-1.,-0.966666666666667,-0.933333333333333,-0.9,
-0.866666666666667,-0.833333333333333,-0.8,-0.766666666666667,-0.733333333333333,
-0.7,-0.666666666666667,-0.633333333333333,-0.6,-0.566666666666667,-0.533333333333333,
-0.5,-0.466666666666667,-0.433333333333333,-0.4,-0.366666666666667,-0.333333333333333,
-0.3,-0.266666666666667,-0.233333333333333,-0.2,-0.166666666666667,-0.133333333333333,
-0.1,-0.0666666666666667,-0.0333333333333333,0.),(-5.,5.),.UNSPECIFIED.)
GEOMETRIC_REPRESENTATION_ITEM()
RATIONAL_B_SPLINE_SURFACE(((1.,1.),(1.,1.),(1.,1.),(1.,1.),(1.,1.),(1.,
1.),(1.,1.),(1.,1.),(1.,1.),(1.,1.),(1.,1.),(1.,1.),(1.,1.),(1.,1.),(1.,
1.),(1.,1.),(1.,1.),(1.,1.),(1.,1.),(1.,1.),(1.,1.),(1.,1.),(1.,1.),(1.,
1.),(1.,1.),(1.,1.),(1.,1.),(1.,1.),(1.,1.),(1.,1.),(1.,1.),(1.,1.),(1.,
1.),(1.,1.),(1.,1.)))
REPRESENTATION_ITEM('')
SURFACE()
);
#505=(
BOUNDED_SURFACE()
B_SPLINE_SURFACE(5,1,((#39272,#39273),(#39274,#39275),(#39276,#39277),(#39278,
#39279),(#39280,#39281),(#39282,#39283),(#39284,#39285),(#39286,#39287),
(#39288,#39289),(#39290,#39291),(#39292,#39293),(#39294,#39295),(#39296,
#39297),(#39298,#39299),(#39300,#39301),(#39302,#39303),(#39304,#39305),
(#39306,#39307),(#39308,#39309),(#39310,#39311),(#39312,#39313),(#39314,
#39315),(#39316,#39317),(#39318,#39319),(#39320,#39321),(#39322,#39323),
(#39324,#39325),(#39326,#39327),(#39328,#39329),(#39330,#39331),(#39332,
#39333),(#39334,#39335),(#39336,#39337),(#39338,#39339),(#39340,#39341)),
 .UNSPECIFIED.,.F.,.F.,.F.)
B_SPLINE_SURFACE_WITH_KNOTS((6,1,1,1,1,1,1,1,1,1,1,1,1,1,1,1,1,1,1,1,1,
1,1,1,1,1,1,1,1,1,6),(2,2),(0.,0.0333333333333333,0.0666666666666667,0.1,
0.133333333333333,0.166666666666667,0.2,0.233333333333333,0.266666666666667,
0.3,0.333333333333333,0.366666666666667,0.4,0.433333333333333,0.466666666666667,
0.5,0.533333333333333,0.566666666666667,0.6,0.633333333333333,0.666666666666667,
0.7,0.733333333333333,0.766666666666667,0.8,0.833333333333333,0.866666666666667,
0.9,0.933333333333333,0.966666666666667,1.),(-5.,5.),.UNSPECIFIED.)
GEOMETRIC_REPRESENTATION_ITEM()
RATIONAL_B_SPLINE_SURFACE(((1.,1.),(1.,1.),(1.,1.),(1.,1.),(1.,1.),(1.,
1.),(1.,1.),(1.,1.),(1.,1.),(1.,1.),(1.,1.),(1.,1.),(1.,1.),(1.,1.),(1.,
1.),(1.,1.),(1.,1.),(1.,1.),(1.,1.),(1.,1.),(1.,1.),(1.,1.),(1.,1.),(1.,
1.),(1.,1.),(1.,1.),(1.,1.),(1.,1.),(1.,1.),(1.,1.),(1.,1.),(1.,1.),(1.,
1.),(1.,1.),(1.,1.)))
REPRESENTATION_ITEM('')
SURFACE()
);
#506=(
BOUNDED_SURFACE()
B_SPLINE_SURFACE(5,1,((#39350,#39351),(#39352,#39353),(#39354,#39355),(#39356,
#39357),(#39358,#39359),(#39360,#39361),(#39362,#39363),(#39364,#39365),
(#39366,#39367),(#39368,#39369),(#39370,#39371),(#39372,#39373),(#39374,
#39375),(#39376,#39377),(#39378,#39379),(#39380,#39381),(#39382,#39383),
(#39384,#39385),(#39386,#39387),(#39388,#39389),(#39390,#39391),(#39392,
#39393),(#39394,#39395),(#39396,#39397),(#39398,#39399),(#39400,#39401),
(#39402,#39403),(#39404,#39405),(#39406,#39407),(#39408,#39409),(#39410,
#39411),(#39412,#39413),(#39414,#39415),(#39416,#39417),(#39418,#39419)),
 .UNSPECIFIED.,.F.,.F.,.F.)
B_SPLINE_SURFACE_WITH_KNOTS((6,1,1,1,1,1,1,1,1,1,1,1,1,1,1,1,1,1,1,1,1,
1,1,1,1,1,1,1,1,1,6),(2,2),(-1.,-0.966666666666667,-0.933333333333333,-0.9,
-0.866666666666667,-0.833333333333333,-0.8,-0.766666666666667,-0.733333333333333,
-0.7,-0.666666666666667,-0.633333333333333,-0.6,-0.566666666666667,-0.533333333333333,
-0.5,-0.466666666666667,-0.433333333333333,-0.4,-0.366666666666667,-0.333333333333333,
-0.3,-0.266666666666667,-0.233333333333333,-0.2,-0.166666666666667,-0.133333333333333,
-0.1,-0.0666666666666667,-0.0333333333333333,0.),(-5.,5.),.UNSPECIFIED.)
GEOMETRIC_REPRESENTATION_ITEM()
RATIONAL_B_SPLINE_SURFACE(((1.,1.),(1.,1.),(1.,1.),(1.,1.),(1.,1.),(1.,
1.),(1.,1.),(1.,1.),(1.,1.),(1.,1.),(1.,1.),(1.,1.),(1.,1.),(1.,1.),(1.,
1.),(1.,1.),(1.,1.),(1.,1.),(1.,1.),(1.,1.),(1.,1.),(1.,1.),(1.,1.),(1.,
1.),(1.,1.),(1.,1.),(1.,1.),(1.,1.),(1.,1.),(1.,1.),(1.,1.),(1.,1.),(1.,
1.),(1.,1.),(1.,1.)))
REPRESENTATION_ITEM('')
SURFACE()
);
#507=(
BOUNDED_SURFACE()
B_SPLINE_SURFACE(5,1,((#39431,#39432),(#39433,#39434),(#39435,#39436),(#39437,
#39438),(#39439,#39440),(#39441,#39442),(#39443,#39444),(#39445,#39446),
(#39447,#39448),(#39449,#39450),(#39451,#39452),(#39453,#39454),(#39455,
#39456),(#39457,#39458),(#39459,#39460),(#39461,#39462),(#39463,#39464),
(#39465,#39466),(#39467,#39468),(#39469,#39470),(#39471,#39472),(#39473,
#39474),(#39475,#39476),(#39477,#39478),(#39479,#39480),(#39481,#39482),
(#39483,#39484),(#39485,#39486),(#39487,#39488),(#39489,#39490),(#39491,
#39492),(#39493,#39494),(#39495,#39496),(#39497,#39498),(#39499,#39500)),
 .UNSPECIFIED.,.F.,.F.,.F.)
B_SPLINE_SURFACE_WITH_KNOTS((6,1,1,1,1,1,1,1,1,1,1,1,1,1,1,1,1,1,1,1,1,
1,1,1,1,1,1,1,1,1,6),(2,2),(0.,0.0333333333333333,0.0666666666666667,0.1,
0.133333333333333,0.166666666666667,0.2,0.233333333333333,0.266666666666667,
0.3,0.333333333333333,0.366666666666667,0.4,0.433333333333333,0.466666666666667,
0.5,0.533333333333333,0.566666666666667,0.6,0.633333333333333,0.666666666666667,
0.7,0.733333333333333,0.766666666666667,0.8,0.833333333333333,0.866666666666667,
0.9,0.933333333333333,0.966666666666667,1.),(-5.,5.),.UNSPECIFIED.)
GEOMETRIC_REPRESENTATION_ITEM()
RATIONAL_B_SPLINE_SURFACE(((1.,1.),(1.,1.),(1.,1.),(1.,1.),(1.,1.),(1.,
1.),(1.,1.),(1.,1.),(1.,1.),(1.,1.),(1.,1.),(1.,1.),(1.,1.),(1.,1.),(1.,
1.),(1.,1.),(1.,1.),(1.,1.),(1.,1.),(1.,1.),(1.,1.),(1.,1.),(1.,1.),(1.,
1.),(1.,1.),(1.,1.),(1.,1.),(1.,1.),(1.,1.),(1.,1.),(1.,1.),(1.,1.),(1.,
1.),(1.,1.),(1.,1.)))
REPRESENTATION_ITEM('')
SURFACE()
);
#508=(
BOUNDED_SURFACE()
B_SPLINE_SURFACE(5,1,((#39509,#39510),(#39511,#39512),(#39513,#39514),(#39515,
#39516),(#39517,#39518),(#39519,#39520),(#39521,#39522),(#39523,#39524),
(#39525,#39526),(#39527,#39528),(#39529,#39530),(#39531,#39532),(#39533,
#39534),(#39535,#39536),(#39537,#39538),(#39539,#39540),(#39541,#39542),
(#39543,#39544),(#39545,#39546),(#39547,#39548),(#39549,#39550),(#39551,
#39552),(#39553,#39554),(#39555,#39556),(#39557,#39558),(#39559,#39560),
(#39561,#39562),(#39563,#39564),(#39565,#39566),(#39567,#39568),(#39569,
#39570),(#39571,#39572),(#39573,#39574),(#39575,#39576),(#39577,#39578)),
 .UNSPECIFIED.,.F.,.F.,.F.)
B_SPLINE_SURFACE_WITH_KNOTS((6,1,1,1,1,1,1,1,1,1,1,1,1,1,1,1,1,1,1,1,1,
1,1,1,1,1,1,1,1,1,6),(2,2),(-1.,-0.966666666666667,-0.933333333333333,-0.9,
-0.866666666666667,-0.833333333333333,-0.8,-0.766666666666667,-0.733333333333333,
-0.7,-0.666666666666667,-0.633333333333333,-0.6,-0.566666666666667,-0.533333333333333,
-0.5,-0.466666666666667,-0.433333333333333,-0.4,-0.366666666666667,-0.333333333333333,
-0.3,-0.266666666666667,-0.233333333333333,-0.2,-0.166666666666667,-0.133333333333333,
-0.1,-0.0666666666666667,-0.0333333333333333,0.),(-5.,5.),.UNSPECIFIED.)
GEOMETRIC_REPRESENTATION_ITEM()
RATIONAL_B_SPLINE_SURFACE(((1.,1.),(1.,1.),(1.,1.),(1.,1.),(1.,1.),(1.,
1.),(1.,1.),(1.,1.),(1.,1.),(1.,1.),(1.,1.),(1.,1.),(1.,1.),(1.,1.),(1.,
1.),(1.,1.),(1.,1.),(1.,1.),(1.,1.),(1.,1.),(1.,1.),(1.,1.),(1.,1.),(1.,
1.),(1.,1.),(1.,1.),(1.,1.),(1.,1.),(1.,1.),(1.,1.),(1.,1.),(1.,1.),(1.,
1.),(1.,1.),(1.,1.)))
REPRESENTATION_ITEM('')
SURFACE()
);
#509=(
BOUNDED_SURFACE()
B_SPLINE_SURFACE(5,1,((#39590,#39591),(#39592,#39593),(#39594,#39595),(#39596,
#39597),(#39598,#39599),(#39600,#39601),(#39602,#39603),(#39604,#39605),
(#39606,#39607),(#39608,#39609),(#39610,#39611),(#39612,#39613),(#39614,
#39615),(#39616,#39617),(#39618,#39619),(#39620,#39621),(#39622,#39623),
(#39624,#39625),(#39626,#39627),(#39628,#39629),(#39630,#39631),(#39632,
#39633),(#39634,#39635),(#39636,#39637),(#39638,#39639),(#39640,#39641),
(#39642,#39643),(#39644,#39645),(#39646,#39647),(#39648,#39649),(#39650,
#39651),(#39652,#39653),(#39654,#39655),(#39656,#39657),(#39658,#39659)),
 .UNSPECIFIED.,.F.,.F.,.F.)
B_SPLINE_SURFACE_WITH_KNOTS((6,1,1,1,1,1,1,1,1,1,1,1,1,1,1,1,1,1,1,1,1,
1,1,1,1,1,1,1,1,1,6),(2,2),(0.,0.0333333333333333,0.0666666666666667,0.1,
0.133333333333333,0.166666666666667,0.2,0.233333333333333,0.266666666666667,
0.3,0.333333333333333,0.366666666666667,0.4,0.433333333333333,0.466666666666667,
0.5,0.533333333333333,0.566666666666667,0.6,0.633333333333333,0.666666666666667,
0.7,0.733333333333333,0.766666666666667,0.8,0.833333333333333,0.866666666666667,
0.9,0.933333333333333,0.966666666666667,1.),(-5.,5.),.UNSPECIFIED.)
GEOMETRIC_REPRESENTATION_ITEM()
RATIONAL_B_SPLINE_SURFACE(((1.,1.),(1.,1.),(1.,1.),(1.,1.),(1.,1.),(1.,
1.),(1.,1.),(1.,1.),(1.,1.),(1.,1.),(1.,1.),(1.,1.),(1.,1.),(1.,1.),(1.,
1.),(1.,1.),(1.,1.),(1.,1.),(1.,1.),(1.,1.),(1.,1.),(1.,1.),(1.,1.),(1.,
1.),(1.,1.),(1.,1.),(1.,1.),(1.,1.),(1.,1.),(1.,1.),(1.,1.),(1.,1.),(1.,
1.),(1.,1.),(1.,1.)))
REPRESENTATION_ITEM('')
SURFACE()
);
#510=(
BOUNDED_SURFACE()
B_SPLINE_SURFACE(5,1,((#39668,#39669),(#39670,#39671),(#39672,#39673),(#39674,
#39675),(#39676,#39677),(#39678,#39679),(#39680,#39681),(#39682,#39683),
(#39684,#39685),(#39686,#39687),(#39688,#39689),(#39690,#39691),(#39692,
#39693),(#39694,#39695),(#39696,#39697),(#39698,#39699),(#39700,#39701),
(#39702,#39703),(#39704,#39705),(#39706,#39707),(#39708,#39709),(#39710,
#39711),(#39712,#39713),(#39714,#39715),(#39716,#39717),(#39718,#39719),
(#39720,#39721),(#39722,#39723),(#39724,#39725),(#39726,#39727),(#39728,
#39729),(#39730,#39731),(#39732,#39733),(#39734,#39735),(#39736,#39737)),
 .UNSPECIFIED.,.F.,.F.,.F.)
B_SPLINE_SURFACE_WITH_KNOTS((6,1,1,1,1,1,1,1,1,1,1,1,1,1,1,1,1,1,1,1,1,
1,1,1,1,1,1,1,1,1,6),(2,2),(-1.,-0.966666666666667,-0.933333333333333,-0.9,
-0.866666666666667,-0.833333333333333,-0.8,-0.766666666666667,-0.733333333333333,
-0.7,-0.666666666666667,-0.633333333333333,-0.6,-0.566666666666667,-0.533333333333333,
-0.5,-0.466666666666667,-0.433333333333333,-0.4,-0.366666666666667,-0.333333333333333,
-0.3,-0.266666666666667,-0.233333333333333,-0.2,-0.166666666666667,-0.133333333333333,
-0.1,-0.0666666666666667,-0.0333333333333333,0.),(-5.,5.),.UNSPECIFIED.)
GEOMETRIC_REPRESENTATION_ITEM()
RATIONAL_B_SPLINE_SURFACE(((1.,1.),(1.,1.),(1.,1.),(1.,1.),(1.,1.),(1.,
1.),(1.,1.),(1.,1.),(1.,1.),(1.,1.),(1.,1.),(1.,1.),(1.,1.),(1.,1.),(1.,
1.),(1.,1.),(1.,1.),(1.,1.),(1.,1.),(1.,1.),(1.,1.),(1.,1.),(1.,1.),(1.,
1.),(1.,1.),(1.,1.),(1.,1.),(1.,1.),(1.,1.),(1.,1.),(1.,1.),(1.,1.),(1.,
1.),(1.,1.),(1.,1.)))
REPRESENTATION_ITEM('')
SURFACE()
);
#511=(
BOUNDED_SURFACE()
B_SPLINE_SURFACE(5,1,((#39749,#39750),(#39751,#39752),(#39753,#39754),(#39755,
#39756),(#39757,#39758),(#39759,#39760),(#39761,#39762),(#39763,#39764),
(#39765,#39766),(#39767,#39768),(#39769,#39770),(#39771,#39772),(#39773,
#39774),(#39775,#39776),(#39777,#39778),(#39779,#39780),(#39781,#39782),
(#39783,#39784),(#39785,#39786),(#39787,#39788),(#39789,#39790),(#39791,
#39792),(#39793,#39794),(#39795,#39796),(#39797,#39798),(#39799,#39800),
(#39801,#39802),(#39803,#39804),(#39805,#39806),(#39807,#39808),(#39809,
#39810),(#39811,#39812),(#39813,#39814),(#39815,#39816),(#39817,#39818)),
 .UNSPECIFIED.,.F.,.F.,.F.)
B_SPLINE_SURFACE_WITH_KNOTS((6,1,1,1,1,1,1,1,1,1,1,1,1,1,1,1,1,1,1,1,1,
1,1,1,1,1,1,1,1,1,6),(2,2),(0.,0.0333333333333333,0.0666666666666667,0.1,
0.133333333333333,0.166666666666667,0.2,0.233333333333333,0.266666666666667,
0.3,0.333333333333333,0.366666666666667,0.4,0.433333333333333,0.466666666666667,
0.5,0.533333333333333,0.566666666666667,0.6,0.633333333333333,0.666666666666667,
0.7,0.733333333333333,0.766666666666667,0.8,0.833333333333333,0.866666666666667,
0.9,0.933333333333333,0.966666666666667,1.),(-5.,5.),.UNSPECIFIED.)
GEOMETRIC_REPRESENTATION_ITEM()
RATIONAL_B_SPLINE_SURFACE(((1.,1.),(1.,1.),(1.,1.),(1.,1.),(1.,1.),(1.,
1.),(1.,1.),(1.,1.),(1.,1.),(1.,1.),(1.,1.),(1.,1.),(1.,1.),(1.,1.),(1.,
1.),(1.,1.),(1.,1.),(1.,1.),(1.,1.),(1.,1.),(1.,1.),(1.,1.),(1.,1.),(1.,
1.),(1.,1.),(1.,1.),(1.,1.),(1.,1.),(1.,1.),(1.,1.),(1.,1.),(1.,1.),(1.,
1.),(1.,1.),(1.,1.)))
REPRESENTATION_ITEM('')
SURFACE()
);
#512=(
BOUNDED_SURFACE()
B_SPLINE_SURFACE(5,1,((#39827,#39828),(#39829,#39830),(#39831,#39832),(#39833,
#39834),(#39835,#39836),(#39837,#39838),(#39839,#39840),(#39841,#39842),
(#39843,#39844),(#39845,#39846),(#39847,#39848),(#39849,#39850),(#39851,
#39852),(#39853,#39854),(#39855,#39856),(#39857,#39858),(#39859,#39860),
(#39861,#39862),(#39863,#39864),(#39865,#39866),(#39867,#39868),(#39869,
#39870),(#39871,#39872),(#39873,#39874),(#39875,#39876),(#39877,#39878),
(#39879,#39880),(#39881,#39882),(#39883,#39884),(#39885,#39886),(#39887,
#39888),(#39889,#39890),(#39891,#39892),(#39893,#39894),(#39895,#39896)),
 .UNSPECIFIED.,.F.,.F.,.F.)
B_SPLINE_SURFACE_WITH_KNOTS((6,1,1,1,1,1,1,1,1,1,1,1,1,1,1,1,1,1,1,1,1,
1,1,1,1,1,1,1,1,1,6),(2,2),(-1.,-0.966666666666667,-0.933333333333333,-0.9,
-0.866666666666667,-0.833333333333333,-0.8,-0.766666666666667,-0.733333333333333,
-0.7,-0.666666666666667,-0.633333333333333,-0.6,-0.566666666666667,-0.533333333333333,
-0.5,-0.466666666666667,-0.433333333333333,-0.4,-0.366666666666667,-0.333333333333333,
-0.3,-0.266666666666667,-0.233333333333333,-0.2,-0.166666666666667,-0.133333333333333,
-0.1,-0.0666666666666667,-0.0333333333333333,0.),(-5.,5.),.UNSPECIFIED.)
GEOMETRIC_REPRESENTATION_ITEM()
RATIONAL_B_SPLINE_SURFACE(((1.,1.),(1.,1.),(1.,1.),(1.,1.),(1.,1.),(1.,
1.),(1.,1.),(1.,1.),(1.,1.),(1.,1.),(1.,1.),(1.,1.),(1.,1.),(1.,1.),(1.,
1.),(1.,1.),(1.,1.),(1.,1.),(1.,1.),(1.,1.),(1.,1.),(1.,1.),(1.,1.),(1.,
1.),(1.,1.),(1.,1.),(1.,1.),(1.,1.),(1.,1.),(1.,1.),(1.,1.),(1.,1.),(1.,
1.),(1.,1.),(1.,1.)))
REPRESENTATION_ITEM('')
SURFACE()
);
#513=(
BOUNDED_SURFACE()
B_SPLINE_SURFACE(5,1,((#39908,#39909),(#39910,#39911),(#39912,#39913),(#39914,
#39915),(#39916,#39917),(#39918,#39919),(#39920,#39921),(#39922,#39923),
(#39924,#39925),(#39926,#39927),(#39928,#39929),(#39930,#39931),(#39932,
#39933),(#39934,#39935),(#39936,#39937),(#39938,#39939),(#39940,#39941),
(#39942,#39943),(#39944,#39945),(#39946,#39947),(#39948,#39949),(#39950,
#39951),(#39952,#39953),(#39954,#39955),(#39956,#39957),(#39958,#39959),
(#39960,#39961),(#39962,#39963),(#39964,#39965),(#39966,#39967),(#39968,
#39969),(#39970,#39971),(#39972,#39973),(#39974,#39975),(#39976,#39977)),
 .UNSPECIFIED.,.F.,.F.,.F.)
B_SPLINE_SURFACE_WITH_KNOTS((6,1,1,1,1,1,1,1,1,1,1,1,1,1,1,1,1,1,1,1,1,
1,1,1,1,1,1,1,1,1,6),(2,2),(0.,0.0333333333333333,0.0666666666666667,0.1,
0.133333333333333,0.166666666666667,0.2,0.233333333333333,0.266666666666667,
0.3,0.333333333333333,0.366666666666667,0.4,0.433333333333333,0.466666666666667,
0.5,0.533333333333333,0.566666666666667,0.6,0.633333333333333,0.666666666666667,
0.7,0.733333333333333,0.766666666666667,0.8,0.833333333333333,0.866666666666667,
0.9,0.933333333333333,0.966666666666667,1.),(-5.,5.),.UNSPECIFIED.)
GEOMETRIC_REPRESENTATION_ITEM()
RATIONAL_B_SPLINE_SURFACE(((1.,1.),(1.,1.),(1.,1.),(1.,1.),(1.,1.),(1.,
1.),(1.,1.),(1.,1.),(1.,1.),(1.,1.),(1.,1.),(1.,1.),(1.,1.),(1.,1.),(1.,
1.),(1.,1.),(1.,1.),(1.,1.),(1.,1.),(1.,1.),(1.,1.),(1.,1.),(1.,1.),(1.,
1.),(1.,1.),(1.,1.),(1.,1.),(1.,1.),(1.,1.),(1.,1.),(1.,1.),(1.,1.),(1.,
1.),(1.,1.),(1.,1.)))
REPRESENTATION_ITEM('')
SURFACE()
);
#514=(
BOUNDED_SURFACE()
B_SPLINE_SURFACE(5,1,((#39986,#39987),(#39988,#39989),(#39990,#39991),(#39992,
#39993),(#39994,#39995),(#39996,#39997),(#39998,#39999),(#40000,#40001),
(#40002,#40003),(#40004,#40005),(#40006,#40007),(#40008,#40009),(#40010,
#40011),(#40012,#40013),(#40014,#40015),(#40016,#40017),(#40018,#40019),
(#40020,#40021),(#40022,#40023),(#40024,#40025),(#40026,#40027),(#40028,
#40029),(#40030,#40031),(#40032,#40033),(#40034,#40035),(#40036,#40037),
(#40038,#40039),(#40040,#40041),(#40042,#40043),(#40044,#40045),(#40046,
#40047),(#40048,#40049),(#40050,#40051),(#40052,#40053),(#40054,#40055)),
 .UNSPECIFIED.,.F.,.F.,.F.)
B_SPLINE_SURFACE_WITH_KNOTS((6,1,1,1,1,1,1,1,1,1,1,1,1,1,1,1,1,1,1,1,1,
1,1,1,1,1,1,1,1,1,6),(2,2),(-1.,-0.966666666666667,-0.933333333333333,-0.9,
-0.866666666666667,-0.833333333333333,-0.8,-0.766666666666667,-0.733333333333333,
-0.7,-0.666666666666667,-0.633333333333333,-0.6,-0.566666666666667,-0.533333333333333,
-0.5,-0.466666666666667,-0.433333333333333,-0.4,-0.366666666666667,-0.333333333333333,
-0.3,-0.266666666666667,-0.233333333333333,-0.2,-0.166666666666667,-0.133333333333333,
-0.1,-0.0666666666666667,-0.0333333333333333,0.),(-5.,5.),.UNSPECIFIED.)
GEOMETRIC_REPRESENTATION_ITEM()
RATIONAL_B_SPLINE_SURFACE(((1.,1.),(1.,1.),(1.,1.),(1.,1.),(1.,1.),(1.,
1.),(1.,1.),(1.,1.),(1.,1.),(1.,1.),(1.,1.),(1.,1.),(1.,1.),(1.,1.),(1.,
1.),(1.,1.),(1.,1.),(1.,1.),(1.,1.),(1.,1.),(1.,1.),(1.,1.),(1.,1.),(1.,
1.),(1.,1.),(1.,1.),(1.,1.),(1.,1.),(1.,1.),(1.,1.),(1.,1.),(1.,1.),(1.,
1.),(1.,1.),(1.,1.)))
REPRESENTATION_ITEM('')
SURFACE()
);
#515=(
BOUNDED_SURFACE()
B_SPLINE_SURFACE(5,1,((#40067,#40068),(#40069,#40070),(#40071,#40072),(#40073,
#40074),(#40075,#40076),(#40077,#40078),(#40079,#40080),(#40081,#40082),
(#40083,#40084),(#40085,#40086),(#40087,#40088),(#40089,#40090),(#40091,
#40092),(#40093,#40094),(#40095,#40096),(#40097,#40098),(#40099,#40100),
(#40101,#40102),(#40103,#40104),(#40105,#40106),(#40107,#40108),(#40109,
#40110),(#40111,#40112),(#40113,#40114),(#40115,#40116),(#40117,#40118),
(#40119,#40120),(#40121,#40122),(#40123,#40124),(#40125,#40126),(#40127,
#40128),(#40129,#40130),(#40131,#40132),(#40133,#40134),(#40135,#40136)),
 .UNSPECIFIED.,.F.,.F.,.F.)
B_SPLINE_SURFACE_WITH_KNOTS((6,1,1,1,1,1,1,1,1,1,1,1,1,1,1,1,1,1,1,1,1,
1,1,1,1,1,1,1,1,1,6),(2,2),(0.,0.0333333333333333,0.0666666666666667,0.1,
0.133333333333333,0.166666666666667,0.2,0.233333333333333,0.266666666666667,
0.3,0.333333333333333,0.366666666666667,0.4,0.433333333333333,0.466666666666667,
0.5,0.533333333333333,0.566666666666667,0.6,0.633333333333333,0.666666666666667,
0.7,0.733333333333333,0.766666666666667,0.8,0.833333333333333,0.866666666666667,
0.9,0.933333333333333,0.966666666666667,1.),(-5.,5.),.UNSPECIFIED.)
GEOMETRIC_REPRESENTATION_ITEM()
RATIONAL_B_SPLINE_SURFACE(((1.,1.),(1.,1.),(1.,1.),(1.,1.),(1.,1.),(1.,
1.),(1.,1.),(1.,1.),(1.,1.),(1.,1.),(1.,1.),(1.,1.),(1.,1.),(1.,1.),(1.,
1.),(1.,1.),(1.,1.),(1.,1.),(1.,1.),(1.,1.),(1.,1.),(1.,1.),(1.,1.),(1.,
1.),(1.,1.),(1.,1.),(1.,1.),(1.,1.),(1.,1.),(1.,1.),(1.,1.),(1.,1.),(1.,
1.),(1.,1.),(1.,1.)))
REPRESENTATION_ITEM('')
SURFACE()
);
#516=(
BOUNDED_SURFACE()
B_SPLINE_SURFACE(5,1,((#40145,#40146),(#40147,#40148),(#40149,#40150),(#40151,
#40152),(#40153,#40154),(#40155,#40156),(#40157,#40158),(#40159,#40160),
(#40161,#40162),(#40163,#40164),(#40165,#40166),(#40167,#40168),(#40169,
#40170),(#40171,#40172),(#40173,#40174),(#40175,#40176),(#40177,#40178),
(#40179,#40180),(#40181,#40182),(#40183,#40184),(#40185,#40186),(#40187,
#40188),(#40189,#40190),(#40191,#40192),(#40193,#40194),(#40195,#40196),
(#40197,#40198),(#40199,#40200),(#40201,#40202),(#40203,#40204),(#40205,
#40206),(#40207,#40208),(#40209,#40210),(#40211,#40212),(#40213,#40214)),
 .UNSPECIFIED.,.F.,.F.,.F.)
B_SPLINE_SURFACE_WITH_KNOTS((6,1,1,1,1,1,1,1,1,1,1,1,1,1,1,1,1,1,1,1,1,
1,1,1,1,1,1,1,1,1,6),(2,2),(-1.,-0.966666666666667,-0.933333333333333,-0.9,
-0.866666666666667,-0.833333333333333,-0.8,-0.766666666666667,-0.733333333333333,
-0.7,-0.666666666666667,-0.633333333333333,-0.6,-0.566666666666667,-0.533333333333333,
-0.5,-0.466666666666667,-0.433333333333333,-0.4,-0.366666666666667,-0.333333333333333,
-0.3,-0.266666666666667,-0.233333333333333,-0.2,-0.166666666666667,-0.133333333333333,
-0.1,-0.0666666666666667,-0.0333333333333333,0.),(-5.,5.),.UNSPECIFIED.)
GEOMETRIC_REPRESENTATION_ITEM()
RATIONAL_B_SPLINE_SURFACE(((1.,1.),(1.,1.),(1.,1.),(1.,1.),(1.,1.),(1.,
1.),(1.,1.),(1.,1.),(1.,1.),(1.,1.),(1.,1.),(1.,1.),(1.,1.),(1.,1.),(1.,
1.),(1.,1.),(1.,1.),(1.,1.),(1.,1.),(1.,1.),(1.,1.),(1.,1.),(1.,1.),(1.,
1.),(1.,1.),(1.,1.),(1.,1.),(1.,1.),(1.,1.),(1.,1.),(1.,1.),(1.,1.),(1.,
1.),(1.,1.),(1.,1.)))
REPRESENTATION_ITEM('')
SURFACE()
);
#517=(
BOUNDED_SURFACE()
B_SPLINE_SURFACE(5,1,((#40226,#40227),(#40228,#40229),(#40230,#40231),(#40232,
#40233),(#40234,#40235),(#40236,#40237),(#40238,#40239),(#40240,#40241),
(#40242,#40243),(#40244,#40245),(#40246,#40247),(#40248,#40249),(#40250,
#40251),(#40252,#40253),(#40254,#40255),(#40256,#40257),(#40258,#40259),
(#40260,#40261),(#40262,#40263),(#40264,#40265),(#40266,#40267),(#40268,
#40269),(#40270,#40271),(#40272,#40273),(#40274,#40275),(#40276,#40277),
(#40278,#40279),(#40280,#40281),(#40282,#40283),(#40284,#40285),(#40286,
#40287),(#40288,#40289),(#40290,#40291),(#40292,#40293),(#40294,#40295)),
 .UNSPECIFIED.,.F.,.F.,.F.)
B_SPLINE_SURFACE_WITH_KNOTS((6,1,1,1,1,1,1,1,1,1,1,1,1,1,1,1,1,1,1,1,1,
1,1,1,1,1,1,1,1,1,6),(2,2),(0.,0.0333333333333333,0.0666666666666667,0.1,
0.133333333333333,0.166666666666667,0.2,0.233333333333333,0.266666666666667,
0.3,0.333333333333333,0.366666666666667,0.4,0.433333333333333,0.466666666666667,
0.5,0.533333333333333,0.566666666666667,0.6,0.633333333333333,0.666666666666667,
0.7,0.733333333333333,0.766666666666667,0.8,0.833333333333333,0.866666666666667,
0.9,0.933333333333333,0.966666666666667,1.),(-5.,5.),.UNSPECIFIED.)
GEOMETRIC_REPRESENTATION_ITEM()
RATIONAL_B_SPLINE_SURFACE(((1.,1.),(1.,1.),(1.,1.),(1.,1.),(1.,1.),(1.,
1.),(1.,1.),(1.,1.),(1.,1.),(1.,1.),(1.,1.),(1.,1.),(1.,1.),(1.,1.),(1.,
1.),(1.,1.),(1.,1.),(1.,1.),(1.,1.),(1.,1.),(1.,1.),(1.,1.),(1.,1.),(1.,
1.),(1.,1.),(1.,1.),(1.,1.),(1.,1.),(1.,1.),(1.,1.),(1.,1.),(1.,1.),(1.,
1.),(1.,1.),(1.,1.)))
REPRESENTATION_ITEM('')
SURFACE()
);
#518=CYLINDRICAL_SURFACE('',#27096,6.25);
#519=CYLINDRICAL_SURFACE('',#27139,6.25);
#520=CYLINDRICAL_SURFACE('',#27145,3.);
#521=CYLINDRICAL_SURFACE('',#27154,3.);
#522=CYLINDRICAL_SURFACE('',#27159,4.64999999999896);
#523=CYLINDRICAL_SURFACE('',#27162,4.6500000000015);
#524=CYLINDRICAL_SURFACE('',#27165,4.64999999999968);
#525=CYLINDRICAL_SURFACE('',#27168,4.64999999999928);
#526=CYLINDRICAL_SURFACE('',#27171,4.6500000000004);
#527=CYLINDRICAL_SURFACE('',#27174,4.64999999999845);
#528=CYLINDRICAL_SURFACE('',#27177,4.64999999999964);
#529=CYLINDRICAL_SURFACE('',#27180,4.64999999999968);
#530=CYLINDRICAL_SURFACE('',#27183,4.64999999999896);
#531=CYLINDRICAL_SURFACE('',#27186,4.64999999999943);
#532=CYLINDRICAL_SURFACE('',#27189,4.64999999999985);
#533=CYLINDRICAL_SURFACE('',#27192,4.65000000000067);
#534=CYLINDRICAL_SURFACE('',#27195,4.65000000000029);
#535=CYLINDRICAL_SURFACE('',#27198,4.65000000000076);
#536=CYLINDRICAL_SURFACE('',#27201,4.6499999999995);
#537=CYLINDRICAL_SURFACE('',#27204,4.64999999999985);
#538=CYLINDRICAL_SURFACE('',#27207,4.65000000000067);
#539=CYLINDRICAL_SURFACE('',#27210,4.65000000000016);
#540=CYLINDRICAL_SURFACE('',#27213,6.);
#541=CYLINDRICAL_SURFACE('',#27214,6.);
#542=CYLINDRICAL_SURFACE('',#27215,6.);
#543=CYLINDRICAL_SURFACE('',#27216,6.);
#544=CYLINDRICAL_SURFACE('',#27217,6.);
#545=CYLINDRICAL_SURFACE('',#27218,6.);
#546=CYLINDRICAL_SURFACE('',#27219,6.);
#547=CYLINDRICAL_SURFACE('',#27220,6.);
#548=CYLINDRICAL_SURFACE('',#27221,6.);
#549=CYLINDRICAL_SURFACE('',#27222,6.);
#550=CYLINDRICAL_SURFACE('',#27223,6.);
#551=CYLINDRICAL_SURFACE('',#27224,6.);
#552=CYLINDRICAL_SURFACE('',#27225,6.);
#553=CYLINDRICAL_SURFACE('',#27226,6.);
#554=CYLINDRICAL_SURFACE('',#27227,6.);
#555=CYLINDRICAL_SURFACE('',#27228,6.);
#556=CYLINDRICAL_SURFACE('',#27229,6.);
#557=CYLINDRICAL_SURFACE('',#27230,6.);
#845=FACE_BOUND('',#4061,.T.);
#846=FACE_BOUND('',#4065,.T.);
#847=FACE_BOUND('',#4071,.T.);
#848=FACE_BOUND('',#4075,.T.);
#927=B_SPLINE_CURVE_WITH_KNOTS('',3,(#35359,#35360,#35361,#35362,#35363,
#35364,#35365,#35366),.UNSPECIFIED.,.F.,.F.,(4,2,2,4),(0.,0.132844638508084,
0.516072227163779,0.952446027985499),.UNSPECIFIED.);
#928=B_SPLINE_CURVE_WITH_KNOTS('',3,(#35370,#35371,#35372,#35373,#35374,
#35375,#35376,#35377,#35378,#35379,#35380,#35381,#35382,#35383,#35384,#35385,
#35386,#35387,#35388,#35389,#35390,#35391,#35392,#35393,#35394,#35395,#35396,
#35397,#35398,#35399,#35400,#35401,#35402,#35403,#35404,#35405,#35406,#35407,
#35408,#35409,#35410,#35411,#35412,#35413,#35414,#35415),.UNSPECIFIED.,
 .F.,.F.,(4,3,3,3,3,3,3,3,3,3,3,3,3,3,3,4),(0.0570515547696962,0.149568289595802,
0.223514482269147,0.282749049350133,0.347422910484109,0.403643225845913,
0.449479112897856,0.49960329648389,0.536801063595721,0.570796167721486,
0.605256849208612,0.653238995251095,0.689225604782957,0.723986222716722,
0.763860497206074,0.797185433378544),.UNSPECIFIED.);
#929=B_SPLINE_CURVE_WITH_KNOTS('',3,(#35423,#35424,#35425,#35426,#35427,
#35428,#35429,#35430),.UNSPECIFIED.,.F.,.F.,(4,2,2,4),(0.,0.132844645404084,
0.506252028814034,0.808059701573943),.UNSPECIFIED.);
#930=B_SPLINE_CURVE_WITH_KNOTS('',3,(#35434,#35435,#35436,#35437,#35438,
#35439,#35440,#35441,#35442,#35443,#35444,#35445,#35446,#35447,#35448,#35449,
#35450,#35451,#35452,#35453,#35454,#35455,#35456,#35457,#35458,#35459,#35460,
#35461,#35462,#35463,#35464,#35465,#35466,#35467,#35468,#35469,#35470,#35471,
#35472,#35473,#35474,#35475,#35476,#35477,#35478,#35479),.UNSPECIFIED.,
 .F.,.F.,(4,3,3,3,3,3,3,3,3,3,3,3,3,3,3,4),(0.119257110722831,0.259765467187379,
0.372070105050779,0.462031684316788,0.560254105414672,0.645637837542741,
0.715250379918589,0.791375706431016,0.847869238432041,0.899498775585672,
0.951835401168699,1.02470754148633,1.07936164672455,1.1321537960343,1.19271223244992,
1.24332396243922),.UNSPECIFIED.);
#931=B_SPLINE_CURVE_WITH_KNOTS('',3,(#35487,#35488,#35489,#35490,#35491,
#35492,#35493,#35494),.UNSPECIFIED.,.F.,.F.,(4,2,2,4),(0.,0.132844651236982,
0.50625209941203,0.808059823281027),.UNSPECIFIED.);
#932=B_SPLINE_CURVE_WITH_KNOTS('',3,(#35498,#35499,#35500,#35501,#35502,
#35503,#35504,#35505),.UNSPECIFIED.,.F.,.F.,(4,2,2,4),(0.119257110624965,
0.656228060783636,0.967756326223977,1.24332397370374),.UNSPECIFIED.);
#933=B_SPLINE_CURVE_WITH_KNOTS('',3,(#35513,#35514,#35515,#35516,#35517,
#35518,#35519,#35520),.UNSPECIFIED.,.F.,.F.,(4,2,2,4),(0.,0.13284465519222,
0.506252154763523,0.80805991875116),.UNSPECIFIED.);
#934=B_SPLINE_CURVE_WITH_KNOTS('',3,(#35524,#35525,#35526,#35527,#35528,
#35529,#35530,#35531),.UNSPECIFIED.,.F.,.F.,(4,2,2,4),(0.119257110675847,
0.656228061682481,0.967756327568862,1.2433239759647),.UNSPECIFIED.);
#935=B_SPLINE_CURVE_WITH_KNOTS('',3,(#35539,#35540,#35541,#35542,#35543,
#35544,#35545,#35546),.UNSPECIFIED.,.F.,.F.,(4,2,2,4),(0.,0.132844659512976,
0.506252186151232,0.808059968862547),.UNSPECIFIED.);
#936=B_SPLINE_CURVE_WITH_KNOTS('',3,(#35550,#35551,#35552,#35553,#35554,
#35555,#35556,#35557,#35558,#35559,#35560,#35561,#35562,#35563,#35564,#35565,
#35566,#35567,#35568,#35569,#35570,#35571,#35572,#35573,#35574,#35575,#35576,
#35577,#35578,#35579,#35580,#35581,#35582,#35583,#35584,#35585,#35586,#35587,
#35588,#35589,#35590,#35591,#35592,#35593,#35594,#35595),.UNSPECIFIED.,
 .F.,.F.,(4,3,3,3,3,3,3,3,3,3,3,3,3,3,3,4),(0.119257110749042,0.259765469653336,
0.372070124544791,0.462031702597275,0.560254122921395,0.645637855304144,
0.715250398053293,0.791375721829739,0.847869254348945,0.899498792238198,
0.951835419100633,1.02470755982132,1.07936166536184,1.13215381569044,1.19271225399545,
1.24332398198339),.UNSPECIFIED.);
#937=B_SPLINE_CURVE_WITH_KNOTS('',3,(#35603,#35604,#35605,#35606,#35607,
#35608,#35609,#35610),.UNSPECIFIED.,.F.,.F.,(4,2,2,4),(0.,0.132844660225076,
0.50625220794817,0.808060006746839),.UNSPECIFIED.);
#938=B_SPLINE_CURVE_WITH_KNOTS('',3,(#35614,#35615,#35616,#35617,#35618,
#35619,#35620,#35621,#35622,#35623,#35624,#35625,#35626,#35627,#35628,#35629,
#35630,#35631,#35632,#35633,#35634,#35635,#35636,#35637,#35638,#35639,#35640,
#35641,#35642,#35643,#35644,#35645,#35646,#35647,#35648,#35649,#35650,#35651,
#35652,#35653,#35654,#35655,#35656,#35657,#35658,#35659),.UNSPECIFIED.,
 .F.,.F.,(4,3,3,3,3,3,3,3,3,3,3,3,3,3,3,4),(0.119257110935751,0.259765470643982,
0.372070120535554,0.462031699629386,0.560254116907991,0.645637850869692,
0.715250394186009,0.791375722521945,0.847869255781902,0.899498793924427,
0.951835420553605,1.0247075625656,1.0793616690746,1.1321538192465,1.19271225740627,
1.2433239886016),.UNSPECIFIED.);
#939=B_SPLINE_CURVE_WITH_KNOTS('',3,(#35667,#35668,#35669,#35670,#35671,
#35672,#35673,#35674),.UNSPECIFIED.,.F.,.F.,(4,2,2,4),(0.,0.132844662938583,
0.506252246824074,0.808060074600784),.UNSPECIFIED.);
#940=B_SPLINE_CURVE_WITH_KNOTS('',3,(#35678,#35679,#35680,#35681,#35682,
#35683,#35684,#35685,#35686,#35687,#35688,#35689,#35690,#35691,#35692,#35693,
#35694,#35695,#35696,#35697,#35698,#35699,#35700,#35701,#35702,#35703,#35704,
#35705,#35706,#35707,#35708,#35709,#35710,#35711,#35712,#35713,#35714,#35715,
#35716,#35717,#35718,#35719,#35720,#35721,#35722,#35723),.UNSPECIFIED.,
 .F.,.F.,(4,3,3,3,3,3,3,3,3,3,3,3,3,3,3,4),(0.119257111119166,0.259765471826694,
0.37207011961253,0.462031700004267,0.560254117679798,0.645637852567247,
0.715250396938671,0.791375727041412,0.847869260758659,0.899498799503518,
0.951835426609056,1.02470756915164,1.07936167605858,1.13215382706252,1.19271226527703,
1.24332399677939),.UNSPECIFIED.);
#941=B_SPLINE_CURVE_WITH_KNOTS('',3,(#35731,#35732,#35733,#35734,#35735,
#35736,#35737,#35738),.UNSPECIFIED.,.F.,.F.,(4,2,2,4),(0.,0.132844662332266,
0.506252246901422,0.808060074727922),.UNSPECIFIED.);
#942=B_SPLINE_CURVE_WITH_KNOTS('',3,(#35742,#35743,#35744,#35745,#35746,
#35747,#35748,#35749,#35750,#35751,#35752,#35753,#35754,#35755,#35756,#35757,
#35758,#35759,#35760,#35761,#35762,#35763,#35764,#35765,#35766,#35767,#35768,
#35769,#35770,#35771,#35772,#35773,#35774,#35775,#35776,#35777,#35778,#35779,
#35780,#35781,#35782,#35783,#35784,#35785,#35786,#35787),.UNSPECIFIED.,
 .F.,.F.,(4,3,3,3,3,3,3,3,3,3,3,3,3,3,3,4),(0.119257111366122,0.259765473891839,
0.372070110740388,0.462031694612758,0.560254112754749,0.645637850106888,
0.715250395993883,0.791375732012897,0.847869266957768,0.899498806411333,
0.951835433730862,1.02470757819111,1.0793616865363,1.13215383802383,1.19271227633857,
1.24332401157186),.UNSPECIFIED.);
#943=B_SPLINE_CURVE_WITH_KNOTS('',3,(#35795,#35796,#35797,#35798,#35799,
#35800,#35801,#35802),.UNSPECIFIED.,.F.,.F.,(4,2,2,4),(0.,0.132844673397704,
0.506252379761466,0.808060307624835),.UNSPECIFIED.);
#944=B_SPLINE_CURVE_WITH_KNOTS('',3,(#35806,#35807,#35808,#35809,#35810,
#35811,#35812,#35813,#35814,#35815,#35816,#35817,#35818,#35819,#35820,#35821,
#35822,#35823,#35824,#35825,#35826,#35827,#35828,#35829,#35830,#35831,#35832,
#35833,#35834,#35835,#35836,#35837,#35838,#35839,#35840,#35841,#35842,#35843,
#35844,#35845,#35846,#35847,#35848,#35849,#35850,#35851),.UNSPECIFIED.,
 .F.,.F.,(4,3,3,3,3,3,3,3,3,3,3,3,3,3,3,4),(0.119257111629581,0.25976547574254,
0.372070105266965,0.462031691347436,0.560254108875743,0.645637848332932,
0.715250395621009,0.791375736838517,0.847869272800359,0.899498812911096,
0.951835440390312,1.02470758642605,1.07936169595285,1.13215384794752,1.19271228630097,
1.24332402453326),.UNSPECIFIED.);
#945=B_SPLINE_CURVE_WITH_KNOTS('',3,(#35859,#35860,#35861,#35862,#35863,
#35864,#35865,#35866),.UNSPECIFIED.,.F.,.F.,(4,2,2,4),(0.,0.13284466924466,
0.516072631745704,0.952446861020481),.UNSPECIFIED.);
#946=B_SPLINE_CURVE_WITH_KNOTS('',3,(#35870,#35871,#35872,#35873,#35874,
#35875),.UNSPECIFIED.,.F.,.F.,(4,2,4),(0.0570515528938123,0.427835960222195,
0.797185331883135),.UNSPECIFIED.);
#947=B_SPLINE_CURVE_WITH_KNOTS('',3,(#35883,#35884,#35885,#35886,#35887,
#35888,#35889,#35890),.UNSPECIFIED.,.F.,.F.,(4,2,2,4),(0.,0.132844667776373,
0.50625232484217,0.80806021526576),.UNSPECIFIED.);
#948=B_SPLINE_CURVE_WITH_KNOTS('',3,(#35894,#35895,#35896,#35897,#35898,
#35899,#35900,#35901),.UNSPECIFIED.,.F.,.F.,(4,2,2,4),(0.11925711175789,
0.65622808055564,0.96775635514001,1.2433240286364),.UNSPECIFIED.);
#949=B_SPLINE_CURVE_WITH_KNOTS('',3,(#35909,#35910,#35911,#35912,#35913,
#35914,#35915,#35916),.UNSPECIFIED.,.F.,.F.,(4,2,2,4),(0.,0.132844663472207,
0.506252284758126,0.808060148341119),.UNSPECIFIED.);
#950=B_SPLINE_CURVE_WITH_KNOTS('',3,(#35920,#35921,#35922,#35923,#35924,
#35925,#35926,#35927,#35928,#35929,#35930,#35931,#35932,#35933,#35934,#35935,
#35936,#35937,#35938,#35939,#35940,#35941,#35942,#35943,#35944,#35945,#35946,
#35947,#35948,#35949,#35950,#35951,#35952,#35953,#35954,#35955,#35956,#35957,
#35958,#35959,#35960,#35961,#35962,#35963,#35964,#35965),.UNSPECIFIED.,
 .F.,.F.,(4,3,3,3,3,3,3,3,3,3,3,3,3,3,3,4),(0.119257111880342,0.259765477112128,
0.372070088145812,0.462031678747241,0.560254098178944,0.645637840123405,
0.715250389444509,0.791375737515883,0.847869274543226,0.899498815448392,
0.951835443060419,1.02470759072897,1.07936170148039,1.13215385418117,1.19271229155254,
1.24332403373463),.UNSPECIFIED.);
#951=B_SPLINE_CURVE_WITH_KNOTS('',3,(#35973,#35974,#35975,#35976,#35977,
#35978,#35979,#35980),.UNSPECIFIED.,.F.,.F.,(4,2,2,4),(0.,0.132844658495434,
0.506252224582906,0.808060045014047),.UNSPECIFIED.);
#952=B_SPLINE_CURVE_WITH_KNOTS('',3,(#35984,#35985,#35986,#35987,#35988,
#35989,#35990,#35991,#35992,#35993,#35994,#35995,#35996,#35997,#35998,#35999,
#36000,#36001,#36002,#36003,#36004,#36005,#36006,#36007,#36008,#36009,#36010,
#36011,#36012,#36013,#36014,#36015,#36016,#36017,#36018,#36019,#36020,#36021,
#36022,#36023,#36024,#36025,#36026,#36027,#36028,#36029),.UNSPECIFIED.,
 .F.,.F.,(4,3,3,3,3,3,3,3,3,3,3,3,3,3,3,4),(0.119257111768233,0.259765476607262,
0.372070087318006,0.462031678446782,0.56025410111,0.645637842281308,0.715250391588022,
0.79137573761201,0.847869274220567,0.899498815109955,0.951835442916956,
1.02470758980783,1.07936169997599,1.13215385283319,1.19271229000116,1.24332403048047),
 .UNSPECIFIED.);
#953=B_SPLINE_CURVE_WITH_KNOTS('',3,(#36037,#36038,#36039,#36040,#36041,
#36042,#36043,#36044),.UNSPECIFIED.,.F.,.F.,(4,2,2,4),(0.,0.13284465245657,
0.506252146299661,0.808059910467814),.UNSPECIFIED.);
#954=B_SPLINE_CURVE_WITH_KNOTS('',3,(#36048,#36049,#36050,#36051,#36052,
#36053,#36054,#36055,#36056,#36057,#36058,#36059,#36060,#36061,#36062,#36063,
#36064,#36065,#36066,#36067,#36068,#36069,#36070,#36071,#36072,#36073,#36074,
#36075,#36076,#36077,#36078,#36079,#36080,#36081,#36082,#36083,#36084,#36085,
#36086,#36087,#36088,#36089,#36090,#36091,#36092,#36093),.UNSPECIFIED.,
 .F.,.F.,(4,3,3,3,3,3,3,3,3,3,3,3,3,3,3,4),(0.119257111589422,0.259765475268004,
0.372070087430169,0.462031677585357,0.560254102164649,0.645637842021328,
0.715250390618003,0.791375733532979,0.847869269468616,0.899498810014054,
0.951835437747858,1.02470758356541,1.07936169292858,1.13215384569843,1.19271228256891,
1.24332402101808),.UNSPECIFIED.);
#955=B_SPLINE_CURVE_WITH_KNOTS('',3,(#36101,#36102,#36103,#36104,#36105,
#36106,#36107,#36108),.UNSPECIFIED.,.F.,.F.,(4,2,2,4),(0.,0.132844642748753,
0.506252042985508,0.808059732577867),.UNSPECIFIED.);
#956=B_SPLINE_CURVE_WITH_KNOTS('',3,(#36112,#36113,#36114,#36115,#36116,
#36117,#36118,#36119,#36120,#36121,#36122,#36123,#36124,#36125,#36126,#36127,
#36128,#36129,#36130,#36131,#36132,#36133,#36134,#36135,#36136,#36137,#36138,
#36139,#36140,#36141,#36142,#36143,#36144,#36145,#36146,#36147,#36148,#36149,
#36150,#36151,#36152,#36153,#36154,#36155,#36156,#36157),.UNSPECIFIED.,
 .F.,.F.,(4,3,3,3,3,3,3,3,3,3,3,3,3,3,3,4),(0.11925711158155,0.259765474036443,
0.37207007811818,0.462031669168862,0.560254093454163,0.64563783317498,0.715250381276493,
0.791375725677586,0.847869261370474,0.899498801276523,0.951835428081933,
1.02470757386662,1.07936168320514,1.132153835061,1.19271227143741,1.2433240112207),
 .UNSPECIFIED.);
#957=B_SPLINE_CURVE_WITH_KNOTS('',3,(#36165,#36166,#36167,#36168,#36169,
#36170,#36171,#36172),.UNSPECIFIED.,.F.,.F.,(4,2,2,4),(0.,0.132844640346774,
0.506251998634185,0.808059655501969),.UNSPECIFIED.);
#958=B_SPLINE_CURVE_WITH_KNOTS('',3,(#36176,#36177,#36178,#36179,#36180,
#36181,#36182,#36183,#36184,#36185,#36186,#36187,#36188,#36189,#36190,#36191,
#36192,#36193,#36194,#36195,#36196,#36197,#36198,#36199,#36200,#36201,#36202,
#36203,#36204,#36205,#36206,#36207,#36208,#36209,#36210,#36211,#36212,#36213,
#36214,#36215,#36216,#36217,#36218,#36219,#36220,#36221),.UNSPECIFIED.,
 .F.,.F.,(4,3,3,3,3,3,3,3,3,3,3,3,3,3,3,4),(0.119257111275641,0.259765471844383,
0.372070088547094,0.462031674851804,0.56025409860193,0.645637835754886,
0.715250382069428,0.791375720258739,0.847869254704594,0.899498793847599,
0.951835420477167,1.02470756431427,1.0793616721921,1.13215382332698,1.19271225959965,
1.24332399582558),.UNSPECIFIED.);
#959=B_SPLINE_CURVE_WITH_KNOTS('',3,(#36229,#36230,#36231,#36232,#36233,
#36234,#36235,#36236),.UNSPECIFIED.,.F.,.F.,(4,2,2,4),(0.,0.132844649562065,
0.506252093176766,0.808059817747012),.UNSPECIFIED.);
#960=B_SPLINE_CURVE_WITH_KNOTS('',3,(#36240,#36241,#36242,#36243,#36244,
#36245,#36246,#36247,#36248,#36249,#36250,#36251,#36252,#36253,#36254,#36255,
#36256,#36257,#36258,#36259,#36260,#36261,#36262,#36263,#36264,#36265,#36266,
#36267,#36268,#36269,#36270,#36271,#36272,#36273,#36274,#36275,#36276,#36277,
#36278,#36279,#36280,#36281,#36282,#36283,#36284,#36285),.UNSPECIFIED.,
 .F.,.F.,(4,3,3,3,3,3,3,3,3,3,3,3,3,3,3,4),(0.11925711110465,0.259765470177295,
0.372070093314613,0.462031677669758,0.560254099913928,0.645637835385414,
0.715250380522247,0.791375714853033,0.847869248457131,0.899498786975331,
0.951835413282065,1.024707555883,1.07936166283371,1.13215381358851,1.19271224958777,
1.24332398368582),.UNSPECIFIED.);
#961=B_SPLINE_CURVE_WITH_KNOTS('',3,(#36293,#36294,#36295,#36296,#36297,
#36298,#36299,#36300),.UNSPECIFIED.,.F.,.F.,(4,2,2,4),(0.,0.132844633425521,
0.506251897062758,0.808059476130729),.UNSPECIFIED.);
#962=B_SPLINE_CURVE_WITH_KNOTS('',3,(#36304,#36305,#36306,#36307,#36308,
#36309,#36310,#36311,#36312,#36313,#36314,#36315,#36316,#36317,#36318,#36319,
#36320,#36321,#36322,#36323,#36324,#36325,#36326,#36327,#36328,#36329,#36330,
#36331,#36332,#36333,#36334,#36335,#36336,#36337,#36338,#36339,#36340,#36341,
#36342,#36343,#36344,#36345,#36346,#36347,#36348,#36349),.UNSPECIFIED.,
 .F.,.F.,(4,3,3,3,3,3,3,3,3,3,3,3,3,3,3,4),(0.119257110965343,0.259765469256534,
0.372070096273217,0.462031679137717,0.560254101459727,0.64563783593912,
0.715250380224683,0.791375712237953,0.847869245370068,0.89949878344051,
0.951835409469422,1.02470755142578,1.07936165789306,1.13215380812679,1.19271224425172,
1.24332397729487),.UNSPECIFIED.);
#963=B_SPLINE_CURVE_WITH_KNOTS('',3,(#36370,#36371,#36372,#36373,#36374,
#36375,#36376,#36377,#36378,#36379,#36380,#36381,#36382,#36383,#36384,#36385,
#36386,#36387,#36388,#36389,#36390,#36391,#36392,#36393,#36394,#36395,#36396,
#36397,#36398,#36399,#36400,#36401,#36402,#36403,#36404,#36405,#36406,#36407,
#36408,#36409,#36410,#36411,#36412,#36413,#36414,#36415),.UNSPECIFIED.,
 .F.,.F.,(4,3,3,3,3,3,3,3,3,3,3,3,3,3,3,4),(0.0570515530865148,0.149568276755442,
0.223514452534054,0.28274901337513,0.34742285854684,0.403643169033227,0.449479051155942,
0.49960323633162,0.536800999594909,0.570796099675367,0.605256776272716,
0.65323891781402,0.689225523969997,0.723986137492795,0.763860406328189,
0.79718534243793),.UNSPECIFIED.);
#964=B_SPLINE_CURVE_WITH_KNOTS('',3,(#36423,#36424,#36425,#36426,#36427,
#36428,#36429,#36430),.UNSPECIFIED.,.F.,.F.,(4,2,2,4),(0.,0.132844666637408,
0.506252309287785,0.808060187337575),.UNSPECIFIED.);
#965=B_SPLINE_CURVE_WITH_KNOTS('',3,(#36434,#36435,#36436,#36437,#36438,
#36439,#36440,#36441,#36442,#36443,#36444,#36445,#36446,#36447,#36448,#36449,
#36450,#36451,#36452,#36453,#36454,#36455,#36456,#36457,#36458,#36459,#36460,
#36461,#36462,#36463,#36464,#36465,#36466,#36467,#36468,#36469,#36470,#36471,
#36472,#36473,#36474,#36475,#36476,#36477,#36478,#36479),.UNSPECIFIED.,
 .F.,.F.,(4,3,3,3,3,3,3,3,3,3,3,3,3,3,3,4),(0.119257111738278,0.259765477798221,
0.372070100839862,0.462031689948238,0.560254109920137,0.645637851207348,
0.715250400204313,0.791375744757855,0.847869281690351,0.899498822750789,
0.951835450996311,1.02470759830169,1.07936170878072,1.13215386181501,1.1927123002489,
1.24332404021782),.UNSPECIFIED.);
#966=B_SPLINE_CURVE_WITH_KNOTS('',3,(#36487,#36488,#36489,#36490,#36491,
#36492,#36493,#36494),.UNSPECIFIED.,.F.,.F.,(4,2,2,4),(0.,0.132844665315855,
0.50625230445513,0.808060181601913),.UNSPECIFIED.);
#967=B_SPLINE_CURVE_WITH_KNOTS('',3,(#36498,#36499,#36500,#36501,#36502,
#36503,#36504,#36505,#36506,#36507,#36508,#36509,#36510,#36511,#36512,#36513,
#36514,#36515,#36516,#36517,#36518,#36519,#36520,#36521,#36522,#36523,#36524,
#36525,#36526,#36527,#36528,#36529,#36530,#36531,#36532,#36533,#36534,#36535,
#36536,#36537,#36538,#36539,#36540,#36541,#36542,#36543),.UNSPECIFIED.,
 .F.,.F.,(4,3,3,3,3,3,3,3,3,3,3,3,3,3,3,4),(0.119257111812372,0.259765475731827,
0.372070092505628,0.462031681270809,0.560254101069256,0.645637841331601,
0.71525038929406,0.791375733485408,0.847869269695733,0.899498809903491,
0.951835437077337,1.02470758360001,1.07936169349201,1.13215384552011,1.19271228284677,
1.24332402316801),.UNSPECIFIED.);
#968=B_SPLINE_CURVE_WITH_KNOTS('',3,(#36551,#36552,#36553,#36554,#36555,
#36556,#36557,#36558),.UNSPECIFIED.,.F.,.F.,(4,2,2,4),(0.,0.132844658784055,
0.506252224782715,0.808060043839757),.UNSPECIFIED.);
#969=B_SPLINE_CURVE_WITH_KNOTS('',3,(#36562,#36563,#36564,#36565,#36566,
#36567,#36568,#36569,#36570,#36571,#36572,#36573,#36574,#36575,#36576,#36577,
#36578,#36579,#36580,#36581,#36582,#36583,#36584,#36585,#36586,#36587,#36588,
#36589,#36590,#36591,#36592,#36593,#36594,#36595,#36596,#36597,#36598,#36599,
#36600,#36601,#36602,#36603,#36604,#36605,#36606,#36607),.UNSPECIFIED.,
 .F.,.F.,(4,3,3,3,3,3,3,3,3,3,3,3,3,3,3,4),(0.119257111835025,0.259765477191931,
0.372070087807762,0.46203167897918,0.560254100528681,0.64563784229888,0.715250391776462,
0.79137573900606,0.847869275966586,0.899498816981767,0.951835444817433,
1.02470759228564,1.0793617028868,1.13215385580022,1.19271229305914,1.24332403469027),
 .UNSPECIFIED.);
#970=B_SPLINE_CURVE_WITH_KNOTS('',3,(#36615,#36616,#36617,#36618,#36619,
#36620,#36621,#36622),.UNSPECIFIED.,.F.,.F.,(4,2,2,4),(0.,0.132844654191751,
0.506252166964219,0.808059945349378),.UNSPECIFIED.);
#971=B_SPLINE_CURVE_WITH_KNOTS('',3,(#36626,#36627,#36628,#36629,#36630,
#36631,#36632,#36633),.UNSPECIFIED.,.F.,.F.,(4,2,2,4),(0.119257111680258,
0.656228079177594,0.967756353404116,1.24332402668173),.UNSPECIFIED.);
#972=B_SPLINE_CURVE_WITH_KNOTS('',3,(#36641,#36642,#36643,#36644,#36645,
#36646,#36647,#36648),.UNSPECIFIED.,.F.,.F.,(4,2,2,4),(0.,0.132844645447949,
0.506252076671479,0.808059790455401),.UNSPECIFIED.);
#973=B_SPLINE_CURVE_WITH_KNOTS('',3,(#36652,#36653,#36654,#36655,#36656,
#36657,#36658,#36659,#36660,#36661,#36662,#36663,#36664,#36665,#36666,#36667,
#36668,#36669,#36670,#36671,#36672,#36673,#36674,#36675,#36676,#36677,#36678,
#36679,#36680,#36681,#36682,#36683,#36684,#36685,#36686,#36687,#36688,#36689,
#36690,#36691,#36692,#36693,#36694,#36695,#36696,#36697),.UNSPECIFIED.,
 .F.,.F.,(4,3,3,3,3,3,3,3,3,3,3,3,3,3,3,4),(0.119257111683661,0.259765474766316,
0.372070077979508,0.46203166925924,0.560254093713209,0.64563783404217,0.715250382509683,
0.791375727925691,0.847869263978092,0.899498804160855,0.951835431203088,
1.02470757748854,1.07936168720263,1.13215383920229,1.1927122757105,1.2433240163449),
 .UNSPECIFIED.);
#974=B_SPLINE_CURVE_WITH_KNOTS('',3,(#36705,#36706,#36707,#36708,#36709,
#36710,#36711,#36712),.UNSPECIFIED.,.F.,.F.,(4,2,2,4),(0.,0.132844642681371,
0.506252033924115,0.808059717106107),.UNSPECIFIED.);
#975=B_SPLINE_CURVE_WITH_KNOTS('',3,(#36716,#36717,#36718,#36719,#36720,
#36721,#36722,#36723,#36724,#36725,#36726,#36727,#36728,#36729,#36730,#36731,
#36732,#36733,#36734,#36735,#36736,#36737,#36738,#36739,#36740,#36741,#36742,
#36743,#36744,#36745,#36746,#36747,#36748,#36749,#36750,#36751,#36752,#36753,
#36754,#36755,#36756,#36757,#36758,#36759,#36760,#36761),.UNSPECIFIED.,
 .F.,.F.,(4,3,3,3,3,3,3,3,3,3,3,3,3,3,3,4),(0.119257111394877,0.259765472481849,
0.372070087964051,0.462031675530459,0.560254099488109,0.645637837063428,
0.715250383674388,0.791375722358766,0.847869257075252,0.899498796470126,
0.951835423266047,1.0247075674722,1.07936167562681,1.13215382714539,1.19271226332587,
1.24332400009066),.UNSPECIFIED.);
#976=B_SPLINE_CURVE_WITH_KNOTS('',3,(#36769,#36770,#36771,#36772,#36773,
#36774,#36775,#36776),.UNSPECIFIED.,.F.,.F.,(4,2,2,4),(0.,0.132844642259177,
0.506252014111271,0.808059681312646),.UNSPECIFIED.);
#977=B_SPLINE_CURVE_WITH_KNOTS('',3,(#36780,#36781,#36782,#36783,#36784,
#36785,#36786,#36787,#36788,#36789,#36790,#36791,#36792,#36793,#36794,#36795,
#36796,#36797,#36798,#36799,#36800,#36801,#36802,#36803,#36804,#36805,#36806,
#36807,#36808,#36809,#36810,#36811,#36812,#36813,#36814,#36815,#36816,#36817,
#36818,#36819,#36820,#36821,#36822,#36823,#36824,#36825),.UNSPECIFIED.,
 .F.,.F.,(4,3,3,3,3,3,3,3,3,3,3,3,3,3,3,4),(0.119257111232989,0.259765470932784,
0.372070089852755,0.462031675399422,0.560254097898976,0.645637834265523,
0.715250380101727,0.791375716804756,0.847869250808081,0.899498789609946,
0.951835416007403,1.02470755921339,1.07936166661788,1.1321538176216,1.19271225354742,
1.24332398883135),.UNSPECIFIED.);
#978=B_SPLINE_CURVE_WITH_KNOTS('',3,(#36833,#36834,#36835,#36836,#36837,
#36838,#36839,#36840),.UNSPECIFIED.,.F.,.F.,(4,2,2,4),(0.,0.132844644201326,
0.506252033181429,0.808059713879001),.UNSPECIFIED.);
#979=B_SPLINE_CURVE_WITH_KNOTS('',3,(#36844,#36845,#36846,#36847,#36848,
#36849,#36850,#36851,#36852,#36853,#36854,#36855,#36856,#36857,#36858,#36859,
#36860,#36861,#36862,#36863,#36864,#36865,#36866,#36867,#36868,#36869,#36870,
#36871,#36872,#36873,#36874,#36875,#36876,#36877,#36878,#36879,#36880,#36881,
#36882,#36883,#36884,#36885,#36886,#36887,#36888,#36889),.UNSPECIFIED.,
 .F.,.F.,(4,3,3,3,3,3,3,3,3,3,3,3,3,3,3,4),(0.119257111061743,0.259765469697972,
0.372070088944832,0.46203167354931,0.56025409772518,0.645637833028479,0.715250378035739,
0.791375712286345,0.847869245769498,0.899498784092187,0.951835410097075,
1.0247075526107,1.07936165949592,1.13215380990758,1.19271224573097,1.24332398015157),
 .UNSPECIFIED.);
#980=B_SPLINE_CURVE_WITH_KNOTS('',3,(#36897,#36898,#36899,#36900,#36901,
#36902,#36903,#36904),.UNSPECIFIED.,.F.,.F.,(4,2,2,4),(0.,0.132844636748929,
0.516072211405751,0.952445994998063),.UNSPECIFIED.);
#981=B_SPLINE_CURVE_WITH_KNOTS('',3,(#36908,#36909,#36910,#36911,#36912,
#36913,#36914,#36915,#36916,#36917,#36918,#36919,#36920,#36921,#36922,#36923,
#36924,#36925,#36926,#36927,#36928,#36929,#36930,#36931,#36932,#36933,#36934,
#36935,#36936,#36937,#36938,#36939,#36940,#36941,#36942,#36943,#36944,#36945,
#36946,#36947,#36948,#36949,#36950,#36951,#36952,#36953),.UNSPECIFIED.,
 .F.,.F.,(4,3,3,3,3,3,3,3,3,3,3,3,3,3,3,4),(0.0570515546134941,0.149568288423378,
0.223514476692031,0.282749043798704,0.347422904353558,0.403643219445934,
0.449479106333475,0.499603290613782,0.53680105742363,0.570796161259589,
0.605256842334552,0.653238988024055,0.689225597291183,0.723986214927346,
0.763860488675733,0.797185425092567),.UNSPECIFIED.);
#982=B_SPLINE_CURVE_WITH_KNOTS('',3,(#36961,#36962,#36963,#36964,#36965,
#36966,#36967,#36968),.UNSPECIFIED.,.F.,.F.,(4,2,2,4),(0.,0.132844644704538,
0.506252021113135,0.808059690353989),.UNSPECIFIED.);
#983=B_SPLINE_CURVE_WITH_KNOTS('',3,(#36972,#36973,#36974,#36975,#36976,
#36977,#36978,#36979),.UNSPECIFIED.,.F.,.F.,(4,2,2,4),(0.119257110771861,
0.65622806320778,0.967756328874099,1.24332396436209),.UNSPECIFIED.);
#984=B_SPLINE_CURVE_WITH_KNOTS('',3,(#36987,#36988,#36989,#36990,#36991,
#36992,#36993,#36994),.UNSPECIFIED.,.F.,.F.,(4,2,2,4),(0.,0.132844648302869,
0.506252066960849,0.808059767961743),.UNSPECIFIED.);
#985=B_SPLINE_CURVE_WITH_KNOTS('',3,(#36998,#36999,#37000,#37001,#37002,
#37003,#37004,#37005,#37006,#37007,#37008,#37009,#37010,#37011,#37012,#37013,
#37014,#37015,#37016,#37017,#37018,#37019,#37020,#37021,#37022,#37023,#37024,
#37025,#37026,#37027,#37028,#37029,#37030,#37031,#37032,#37033,#37034,#37035,
#37036,#37037,#37038,#37039,#37040,#37041,#37042,#37043),.UNSPECIFIED.,
 .F.,.F.,(4,3,3,3,3,3,3,3,3,3,3,3,3,3,3,4),(0.119257110621164,0.259765468263962,
0.372070112199727,0.462031691450782,0.560254114472962,0.645637846634284,
0.715250389295661,0.791375714007369,0.847869246226891,0.899498783860491,
0.951835410214567,1.02470755060181,1.07936165589224,1.13215380591584,1.19271224305412,
1.24332397176354),.UNSPECIFIED.);
#986=B_SPLINE_CURVE_WITH_KNOTS('',3,(#37051,#37052,#37053,#37054,#37055,
#37056,#37057,#37058),.UNSPECIFIED.,.F.,.F.,(4,2,2,4),(0.,0.132844653773461,
0.506252139652089,0.808059893305447),.UNSPECIFIED.);
#987=B_SPLINE_CURVE_WITH_KNOTS('',3,(#37062,#37063,#37064,#37065,#37066,
#37067,#37068,#37069,#37070,#37071,#37072,#37073,#37074,#37075,#37076,#37077,
#37078,#37079,#37080,#37081,#37082,#37083,#37084,#37085,#37086,#37087,#37088,
#37089,#37090,#37091,#37092,#37093,#37094,#37095,#37096,#37097,#37098,#37099,
#37100,#37101,#37102,#37103,#37104,#37105,#37106,#37107),.UNSPECIFIED.,
 .F.,.F.,(4,3,3,3,3,3,3,3,3,3,3,3,3,3,3,4),(0.119257110641572,0.259765468385939,
0.372070117379027,0.462031695480993,0.560254117172397,0.64563784910041,
0.715250391578671,0.791375715315744,0.847869247475839,0.899498785035086,
0.951835411419915,1.02470755171406,1.07936165693467,1.13215380684117,1.19271224435265,
1.24332397259651),.UNSPECIFIED.);
#988=B_SPLINE_CURVE_WITH_KNOTS('',3,(#37115,#37116,#37117,#37118,#37119,
#37120,#37121,#37122),.UNSPECIFIED.,.F.,.F.,(4,2,2,4),(0.,0.13284465680416,
0.506252153781493,0.80805991374936),.UNSPECIFIED.);
#989=B_SPLINE_CURVE_WITH_KNOTS('',3,(#37126,#37127,#37128,#37129,#37130,
#37131,#37132,#37133,#37134,#37135,#37136,#37137,#37138,#37139,#37140,#37141,
#37142,#37143,#37144,#37145,#37146,#37147,#37148,#37149,#37150,#37151,#37152,
#37153,#37154,#37155,#37156,#37157,#37158,#37159,#37160,#37161,#37162,#37163,
#37164,#37165,#37166,#37167,#37168,#37169,#37170,#37171),.UNSPECIFIED.,
 .F.,.F.,(4,3,3,3,3,3,3,3,3,3,3,3,3,3,3,4),(0.119257110659739,0.259765468839433,
0.372070119778476,0.462031697519513,0.560254116817873,0.645637849227801,
0.715250391720227,0.79137571663617,0.84786924906881,0.899498786754164,0.951835413160386,
1.02470755389461,1.07936165944528,1.13215380946011,1.19271224707953,1.24332397609729),
 .UNSPECIFIED.);
#990=B_SPLINE_CURVE_WITH_KNOTS('',3,(#37179,#37180,#37181,#37182,#37183,
#37184,#37185,#37186),.UNSPECIFIED.,.F.,.F.,(4,2,2,4),(0.,0.13284465770136,
0.506252176893417,0.808059953558626),.UNSPECIFIED.);
#991=B_SPLINE_CURVE_WITH_KNOTS('',3,(#37190,#37191,#37192,#37193,#37194,
#37195,#37196,#37197),.UNSPECIFIED.,.F.,.F.,(4,2,2,4),(0.119257110811679,
0.656228064026157,0.967756330899547,1.24332398190981),.UNSPECIFIED.);
#992=B_SPLINE_CURVE_WITH_KNOTS('',3,(#37205,#37206,#37207,#37208,#37209,
#37210,#37211,#37212),.UNSPECIFIED.,.F.,.F.,(4,2,2,4),(0.,0.132844660625905,
0.506252215494008,0.808060020062334),.UNSPECIFIED.);
#993=B_SPLINE_CURVE_WITH_KNOTS('',3,(#37216,#37217,#37218,#37219,#37220,
#37221,#37222,#37223,#37224,#37225,#37226,#37227,#37228,#37229,#37230,#37231,
#37232,#37233,#37234,#37235,#37236,#37237,#37238,#37239,#37240,#37241,#37242,
#37243,#37244,#37245,#37246,#37247,#37248,#37249,#37250,#37251,#37252,#37253,
#37254,#37255,#37256,#37257,#37258,#37259,#37260,#37261),.UNSPECIFIED.,
 .F.,.F.,(4,3,3,3,3,3,3,3,3,3,3,3,3,3,3,4),(0.119257111071676,0.259765471515195,
0.372070113835674,0.462031695224013,0.560254113799293,0.64563784890186,
0.715250393228207,0.791375724377874,0.847869258158118,0.899498796808649,
0.951835423647897,1.02470756639088,1.07936167344812,1.13215382428839,1.19271226217066,
1.24332399461983),.UNSPECIFIED.);
#994=B_SPLINE_CURVE_WITH_KNOTS('',3,(#37269,#37270,#37271,#37272,#37273,
#37274,#37275,#37276),.UNSPECIFIED.,.F.,.F.,(4,2,2,4),(0.,0.132844661742616,
0.506252230084776,0.808060044866463),.UNSPECIFIED.);
#995=B_SPLINE_CURVE_WITH_KNOTS('',3,(#37280,#37281,#37282,#37283,#37284,
#37285,#37286,#37287,#37288,#37289,#37290,#37291,#37292,#37293,#37294,#37295,
#37296,#37297,#37298,#37299,#37300,#37301,#37302,#37303,#37304,#37305,#37306,
#37307,#37308,#37309,#37310,#37311,#37312,#37313,#37314,#37315,#37316,#37317,
#37318,#37319,#37320,#37321,#37322,#37323,#37324,#37325),.UNSPECIFIED.,
 .F.,.F.,(4,3,3,3,3,3,3,3,3,3,3,3,3,3,3,4),(0.119257111238407,0.259765472915745,
0.372070114012319,0.462031696197013,0.560254114345044,0.645637850634053,
0.715250395662769,0.791375729222669,0.847869263651974,0.89949880268746,
0.951835429736583,1.02470757346672,1.07936168126432,1.13215383237257,1.19271227073433,
1.24332400465711),.UNSPECIFIED.);
#996=B_SPLINE_CURVE_WITH_KNOTS('',3,(#37333,#37334,#37335,#37336,#37337,
#37338,#37339,#37340),.UNSPECIFIED.,.F.,.F.,(4,2,2,4),(0.,0.132844672918338,
0.50625237183672,0.808060292904816),.UNSPECIFIED.);
#997=B_SPLINE_CURVE_WITH_KNOTS('',3,(#37344,#37345,#37346,#37347,#37348,
#37349,#37350,#37351,#37352,#37353,#37354,#37355,#37356,#37357,#37358,#37359,
#37360,#37361,#37362,#37363,#37364,#37365,#37366,#37367,#37368,#37369,#37370,
#37371,#37372,#37373,#37374,#37375,#37376,#37377,#37378,#37379,#37380,#37381,
#37382,#37383,#37384,#37385,#37386,#37387,#37388,#37389),.UNSPECIFIED.,
 .F.,.F.,(4,3,3,3,3,3,3,3,3,3,3,3,3,3,3,4),(0.119257111410954,0.25976547452879,
0.372070109798341,0.462031694258679,0.560254111872906,0.645637849932998,
0.71525039623539,0.791375733920728,0.847869269224843,0.899498808890005,
0.951835436167286,1.02470758121388,1.07936168999882,1.13215384163373,1.1927122800387,
1.24332401635365),.UNSPECIFIED.);
#998=B_SPLINE_CURVE_WITH_KNOTS('',3,(#37397,#37398,#37399,#37400,#37401,
#37402,#37403,#37404),.UNSPECIFIED.,.F.,.F.,(4,2,2,4),(0.,0.132844669264716,
0.51607262788724,0.952446854621337),.UNSPECIFIED.);
#999=B_SPLINE_CURVE_WITH_KNOTS('',3,(#37513,#37514,#37515,#37516,#37517,
#37518),.UNSPECIFIED.,.F.,.F.,(4,2,4),(0.,5.,9.6),.UNSPECIFIED.);
#1000=B_SPLINE_CURVE_WITH_KNOTS('',3,(#37593,#37594,#37595,#37596,#37597,
#37598),.UNSPECIFIED.,.F.,.F.,(4,2,4),(0.,5.,9.6),.UNSPECIFIED.);
#1001=B_SPLINE_CURVE_WITH_KNOTS('',3,(#37672,#37673,#37674,#37675,#37676,
#37677),.UNSPECIFIED.,.F.,.F.,(4,2,4),(0.,5.,9.6),.UNSPECIFIED.);
#1002=B_SPLINE_CURVE_WITH_KNOTS('',3,(#37752,#37753,#37754,#37755,#37756,
#37757),.UNSPECIFIED.,.F.,.F.,(4,2,4),(0.,5.,9.6),.UNSPECIFIED.);
#1003=B_SPLINE_CURVE_WITH_KNOTS('',3,(#37831,#37832,#37833,#37834,#37835,
#37836),.UNSPECIFIED.,.F.,.F.,(4,2,4),(0.,5.,9.6),.UNSPECIFIED.);
#1004=B_SPLINE_CURVE_WITH_KNOTS('',3,(#37911,#37912,#37913,#37914,#37915,
#37916),.UNSPECIFIED.,.F.,.F.,(4,2,4),(0.,5.,9.6),.UNSPECIFIED.);
#1005=B_SPLINE_CURVE_WITH_KNOTS('',3,(#37990,#37991,#37992,#37993,#37994,
#37995),.UNSPECIFIED.,.F.,.F.,(4,2,4),(0.,5.,9.6),.UNSPECIFIED.);
#1006=B_SPLINE_CURVE_WITH_KNOTS('',3,(#38070,#38071,#38072,#38073,#38074,
#38075),.UNSPECIFIED.,.F.,.F.,(4,2,4),(0.,5.,9.6),.UNSPECIFIED.);
#1007=B_SPLINE_CURVE_WITH_KNOTS('',3,(#38149,#38150,#38151,#38152,#38153,
#38154),.UNSPECIFIED.,.F.,.F.,(4,2,4),(0.,5.,9.6),.UNSPECIFIED.);
#1008=B_SPLINE_CURVE_WITH_KNOTS('',3,(#38229,#38230,#38231,#38232,#38233,
#38234),.UNSPECIFIED.,.F.,.F.,(4,2,4),(0.,5.,9.6),.UNSPECIFIED.);
#1009=B_SPLINE_CURVE_WITH_KNOTS('',3,(#38308,#38309,#38310,#38311,#38312,
#38313),.UNSPECIFIED.,.F.,.F.,(4,2,4),(0.,5.,9.6),.UNSPECIFIED.);
#1010=B_SPLINE_CURVE_WITH_KNOTS('',3,(#38388,#38389,#38390,#38391,#38392,
#38393),.UNSPECIFIED.,.F.,.F.,(4,2,4),(0.,5.,9.6),.UNSPECIFIED.);
#1011=B_SPLINE_CURVE_WITH_KNOTS('',3,(#38467,#38468,#38469,#38470,#38471,
#38472),.UNSPECIFIED.,.F.,.F.,(4,2,4),(0.,5.,9.6),.UNSPECIFIED.);
#1012=B_SPLINE_CURVE_WITH_KNOTS('',3,(#38547,#38548,#38549,#38550,#38551,
#38552),.UNSPECIFIED.,.F.,.F.,(4,2,4),(0.,5.,9.6),.UNSPECIFIED.);
#1013=B_SPLINE_CURVE_WITH_KNOTS('',3,(#38626,#38627,#38628,#38629,#38630,
#38631),.UNSPECIFIED.,.F.,.F.,(4,2,4),(0.,5.,9.6),.UNSPECIFIED.);
#1014=B_SPLINE_CURVE_WITH_KNOTS('',3,(#38706,#38707,#38708,#38709,#38710,
#38711),.UNSPECIFIED.,.F.,.F.,(4,2,4),(0.,5.,9.6),.UNSPECIFIED.);
#1015=B_SPLINE_CURVE_WITH_KNOTS('',3,(#38785,#38786,#38787,#38788,#38789,
#38790),.UNSPECIFIED.,.F.,.F.,(4,2,4),(0.,5.,9.6),.UNSPECIFIED.);
#1016=B_SPLINE_CURVE_WITH_KNOTS('',3,(#38865,#38866,#38867,#38868,#38869,
#38870),.UNSPECIFIED.,.F.,.F.,(4,2,4),(0.,5.,9.6),.UNSPECIFIED.);
#1017=B_SPLINE_CURVE_WITH_KNOTS('',3,(#38944,#38945,#38946,#38947,#38948,
#38949),.UNSPECIFIED.,.F.,.F.,(4,2,4),(0.,5.,9.6),.UNSPECIFIED.);
#1018=B_SPLINE_CURVE_WITH_KNOTS('',3,(#39024,#39025,#39026,#39027,#39028,
#39029),.UNSPECIFIED.,.F.,.F.,(4,2,4),(0.,5.,9.6),.UNSPECIFIED.);
#1019=B_SPLINE_CURVE_WITH_KNOTS('',3,(#39103,#39104,#39105,#39106,#39107,
#39108),.UNSPECIFIED.,.F.,.F.,(4,2,4),(0.,5.,9.6),.UNSPECIFIED.);
#1020=B_SPLINE_CURVE_WITH_KNOTS('',3,(#39183,#39184,#39185,#39186,#39187,
#39188),.UNSPECIFIED.,.F.,.F.,(4,2,4),(0.,5.,9.6),.UNSPECIFIED.);
#1021=B_SPLINE_CURVE_WITH_KNOTS('',3,(#39262,#39263,#39264,#39265,#39266,
#39267),.UNSPECIFIED.,.F.,.F.,(4,2,4),(0.,5.,9.6),.UNSPECIFIED.);
#1022=B_SPLINE_CURVE_WITH_KNOTS('',3,(#39342,#39343,#39344,#39345,#39346,
#39347),.UNSPECIFIED.,.F.,.F.,(4,2,4),(0.,5.,9.6),.UNSPECIFIED.);
#1023=B_SPLINE_CURVE_WITH_KNOTS('',3,(#39421,#39422,#39423,#39424,#39425,
#39426),.UNSPECIFIED.,.F.,.F.,(4,2,4),(0.,5.,9.6),.UNSPECIFIED.);
#1024=B_SPLINE_CURVE_WITH_KNOTS('',3,(#39501,#39502,#39503,#39504,#39505,
#39506),.UNSPECIFIED.,.F.,.F.,(4,2,4),(0.,5.,9.6),.UNSPECIFIED.);
#1025=B_SPLINE_CURVE_WITH_KNOTS('',3,(#39580,#39581,#39582,#39583,#39584,
#39585),.UNSPECIFIED.,.F.,.F.,(4,2,4),(0.,5.,9.6),.UNSPECIFIED.);
#1026=B_SPLINE_CURVE_WITH_KNOTS('',3,(#39660,#39661,#39662,#39663,#39664,
#39665),.UNSPECIFIED.,.F.,.F.,(4,2,4),(0.,5.,9.6),.UNSPECIFIED.);
#1027=B_SPLINE_CURVE_WITH_KNOTS('',3,(#39739,#39740,#39741,#39742,#39743,
#39744),.UNSPECIFIED.,.F.,.F.,(4,2,4),(0.,5.,9.6),.UNSPECIFIED.);
#1028=B_SPLINE_CURVE_WITH_KNOTS('',3,(#39819,#39820,#39821,#39822,#39823,
#39824),.UNSPECIFIED.,.F.,.F.,(4,2,4),(0.,5.,9.6),.UNSPECIFIED.);
#1029=B_SPLINE_CURVE_WITH_KNOTS('',3,(#39898,#39899,#39900,#39901,#39902,
#39903),.UNSPECIFIED.,.F.,.F.,(4,2,4),(0.,5.,9.6),.UNSPECIFIED.);
#1030=B_SPLINE_CURVE_WITH_KNOTS('',3,(#39978,#39979,#39980,#39981,#39982,
#39983),.UNSPECIFIED.,.F.,.F.,(4,2,4),(0.,5.,9.6),.UNSPECIFIED.);
#1031=B_SPLINE_CURVE_WITH_KNOTS('',3,(#40057,#40058,#40059,#40060,#40061,
#40062),.UNSPECIFIED.,.F.,.F.,(4,2,4),(0.,5.,9.6),.UNSPECIFIED.);
#1032=B_SPLINE_CURVE_WITH_KNOTS('',3,(#40137,#40138,#40139,#40140,#40141,
#40142),.UNSPECIFIED.,.F.,.F.,(4,2,4),(0.,5.,9.6),.UNSPECIFIED.);
#1033=B_SPLINE_CURVE_WITH_KNOTS('',3,(#40216,#40217,#40218,#40219,#40220,
#40221),.UNSPECIFIED.,.F.,.F.,(4,2,4),(0.,5.,9.6),.UNSPECIFIED.);
#1034=B_SPLINE_CURVE_WITH_KNOTS('',3,(#40296,#40297,#40298,#40299,#40300,
#40301),.UNSPECIFIED.,.F.,.F.,(4,2,4),(0.,5.,9.6),.UNSPECIFIED.);
#1680=PLANE('',#27059);
#1681=PLANE('',#27102);
#1682=PLANE('',#27141);
#1683=PLANE('',#27147);
#1684=PLANE('',#27152);
#1685=PLANE('',#27158);
#1686=PLANE('',#27160);
#1687=PLANE('',#27161);
#1688=PLANE('',#27163);
#1689=PLANE('',#27164);
#1690=PLANE('',#27166);
#1691=PLANE('',#27167);
#1692=PLANE('',#27169);
#1693=PLANE('',#27170);
#1694=PLANE('',#27172);
#1695=PLANE('',#27173);
#1696=PLANE('',#27175);
#1697=PLANE('',#27176);
#1698=PLANE('',#27178);
#1699=PLANE('',#27179);
#1700=PLANE('',#27181);
#1701=PLANE('',#27182);
#1702=PLANE('',#27184);
#1703=PLANE('',#27185);
#1704=PLANE('',#27187);
#1705=PLANE('',#27188);
#1706=PLANE('',#27190);
#1707=PLANE('',#27191);
#1708=PLANE('',#27193);
#1709=PLANE('',#27194);
#1710=PLANE('',#27196);
#1711=PLANE('',#27197);
#1712=PLANE('',#27199);
#1713=PLANE('',#27200);
#1714=PLANE('',#27202);
#1715=PLANE('',#27203);
#1716=PLANE('',#27205);
#1717=PLANE('',#27206);
#1718=PLANE('',#27208);
#1719=PLANE('',#27209);
#1720=PLANE('',#27211);
#1721=PLANE('',#27212);
#2570=FACE_OUTER_BOUND('',#4059,.T.);
#2571=FACE_OUTER_BOUND('',#4060,.T.);
#2572=FACE_OUTER_BOUND('',#4062,.T.);
#2573=FACE_OUTER_BOUND('',#4063,.T.);
#2574=FACE_OUTER_BOUND('',#4064,.T.);
#2575=FACE_OUTER_BOUND('',#4066,.T.);
#2576=FACE_OUTER_BOUND('',#4067,.T.);
#2577=FACE_OUTER_BOUND('',#4068,.T.);
#2578=FACE_OUTER_BOUND('',#4069,.T.);
#2579=FACE_OUTER_BOUND('',#4070,.T.);
#2580=FACE_OUTER_BOUND('',#4072,.T.);
#2581=FACE_OUTER_BOUND('',#4073,.T.);
#2582=FACE_OUTER_BOUND('',#4074,.T.);
#2583=FACE_OUTER_BOUND('',#4076,.T.);
#2584=FACE_OUTER_BOUND('',#4077,.T.);
#2585=FACE_OUTER_BOUND('',#4078,.T.);
#2586=FACE_OUTER_BOUND('',#4079,.T.);
#2587=FACE_OUTER_BOUND('',#4080,.T.);
#2588=FACE_OUTER_BOUND('',#4081,.T.);
#2589=FACE_OUTER_BOUND('',#4082,.T.);
#2590=FACE_OUTER_BOUND('',#4083,.T.);
#2591=FACE_OUTER_BOUND('',#4084,.T.);
#2592=FACE_OUTER_BOUND('',#4085,.T.);
#2593=FACE_OUTER_BOUND('',#4086,.T.);
#2594=FACE_OUTER_BOUND('',#4087,.T.);
#2595=FACE_OUTER_BOUND('',#4088,.T.);
#2596=FACE_OUTER_BOUND('',#4089,.T.);
#2597=FACE_OUTER_BOUND('',#4090,.T.);
#2598=FACE_OUTER_BOUND('',#4091,.T.);
#2599=FACE_OUTER_BOUND('',#4092,.T.);
#2600=FACE_OUTER_BOUND('',#4093,.T.);
#2601=FACE_OUTER_BOUND('',#4094,.T.);
#2602=FACE_OUTER_BOUND('',#4095,.T.);
#2603=FACE_OUTER_BOUND('',#4096,.T.);
#2604=FACE_OUTER_BOUND('',#4097,.T.);
#2605=FACE_OUTER_BOUND('',#4098,.T.);
#2606=FACE_OUTER_BOUND('',#4099,.T.);
#2607=FACE_OUTER_BOUND('',#4100,.T.);
#2608=FACE_OUTER_BOUND('',#4101,.T.);
#2609=FACE_OUTER_BOUND('',#4102,.T.);
#2610=FACE_OUTER_BOUND('',#4103,.T.);
#2611=FACE_OUTER_BOUND('',#4104,.T.);
#2612=FACE_OUTER_BOUND('',#4105,.T.);
#2613=FACE_OUTER_BOUND('',#4106,.T.);
#2614=FACE_OUTER_BOUND('',#4107,.T.);
#2615=FACE_OUTER_BOUND('',#4108,.T.);
#2616=FACE_OUTER_BOUND('',#4109,.T.);
#2617=FACE_OUTER_BOUND('',#4110,.T.);
#2618=FACE_OUTER_BOUND('',#4111,.T.);
#2619=FACE_OUTER_BOUND('',#4112,.T.);
#2620=FACE_OUTER_BOUND('',#4113,.T.);
#2621=FACE_OUTER_BOUND('',#4114,.T.);
#2622=FACE_OUTER_BOUND('',#4115,.T.);
#2623=FACE_OUTER_BOUND('',#4116,.T.);
#2624=FACE_OUTER_BOUND('',#4117,.T.);
#2625=FACE_OUTER_BOUND('',#4118,.T.);
#2626=FACE_OUTER_BOUND('',#4119,.T.);
#2627=FACE_OUTER_BOUND('',#4120,.T.);
#2628=FACE_OUTER_BOUND('',#4121,.T.);
#2629=FACE_OUTER_BOUND('',#4122,.T.);
#2630=FACE_OUTER_BOUND('',#4123,.T.);
#2631=FACE_OUTER_BOUND('',#4124,.T.);
#2632=FACE_OUTER_BOUND('',#4125,.T.);
#2633=FACE_OUTER_BOUND('',#4126,.T.);
#2634=FACE_OUTER_BOUND('',#4127,.T.);
#2635=FACE_OUTER_BOUND('',#4128,.T.);
#2636=FACE_OUTER_BOUND('',#4129,.T.);
#2637=FACE_OUTER_BOUND('',#4130,.T.);
#2638=FACE_OUTER_BOUND('',#4131,.T.);
#2639=FACE_OUTER_BOUND('',#4132,.T.);
#2640=FACE_OUTER_BOUND('',#4133,.T.);
#2641=FACE_OUTER_BOUND('',#4134,.T.);
#2642=FACE_OUTER_BOUND('',#4135,.T.);
#2643=FACE_OUTER_BOUND('',#4136,.T.);
#2644=FACE_OUTER_BOUND('',#4137,.T.);
#2645=FACE_OUTER_BOUND('',#4138,.T.);
#2646=FACE_OUTER_BOUND('',#4139,.T.);
#2647=FACE_OUTER_BOUND('',#4140,.T.);
#2648=FACE_OUTER_BOUND('',#4141,.T.);
#2649=FACE_OUTER_BOUND('',#4142,.T.);
#2650=FACE_OUTER_BOUND('',#4143,.T.);
#2651=FACE_OUTER_BOUND('',#4144,.T.);
#2652=FACE_OUTER_BOUND('',#4145,.T.);
#2653=FACE_OUTER_BOUND('',#4146,.T.);
#2654=FACE_OUTER_BOUND('',#4147,.T.);
#2655=FACE_OUTER_BOUND('',#4148,.T.);
#2656=FACE_OUTER_BOUND('',#4149,.T.);
#2657=FACE_OUTER_BOUND('',#4150,.T.);
#2658=FACE_OUTER_BOUND('',#4151,.T.);
#2659=FACE_OUTER_BOUND('',#4152,.T.);
#2660=FACE_OUTER_BOUND('',#4153,.T.);
#2661=FACE_OUTER_BOUND('',#4154,.T.);
#2662=FACE_OUTER_BOUND('',#4155,.T.);
#2663=FACE_OUTER_BOUND('',#4156,.T.);
#2664=FACE_OUTER_BOUND('',#4157,.T.);
#2665=FACE_OUTER_BOUND('',#4158,.T.);
#2666=FACE_OUTER_BOUND('',#4159,.T.);
#2667=FACE_OUTER_BOUND('',#4160,.T.);
#2668=FACE_OUTER_BOUND('',#4161,.T.);
#2669=FACE_OUTER_BOUND('',#4162,.T.);
#2670=FACE_OUTER_BOUND('',#4163,.T.);
#2671=FACE_OUTER_BOUND('',#4164,.T.);
#2672=FACE_OUTER_BOUND('',#4165,.T.);
#2673=FACE_OUTER_BOUND('',#4166,.T.);
#2674=FACE_OUTER_BOUND('',#4167,.T.);
#2675=FACE_OUTER_BOUND('',#4168,.T.);
#2676=FACE_OUTER_BOUND('',#4169,.T.);
#2677=FACE_OUTER_BOUND('',#4170,.T.);
#2678=FACE_OUTER_BOUND('',#4171,.T.);
#2679=FACE_OUTER_BOUND('',#4172,.T.);
#2680=FACE_OUTER_BOUND('',#4173,.T.);
#2681=FACE_OUTER_BOUND('',#4174,.T.);
#2682=FACE_OUTER_BOUND('',#4175,.T.);
#2683=FACE_OUTER_BOUND('',#4176,.T.);
#2684=FACE_OUTER_BOUND('',#4177,.T.);
#2685=FACE_OUTER_BOUND('',#4178,.T.);
#2686=FACE_OUTER_BOUND('',#4179,.T.);
#2687=FACE_OUTER_BOUND('',#4180,.T.);
#2688=FACE_OUTER_BOUND('',#4181,.T.);
#2689=FACE_OUTER_BOUND('',#4182,.T.);
#2690=FACE_OUTER_BOUND('',#4183,.T.);
#2691=FACE_OUTER_BOUND('',#4184,.T.);
#2692=FACE_OUTER_BOUND('',#4185,.T.);
#2693=FACE_OUTER_BOUND('',#4186,.T.);
#4059=EDGE_LOOP('',(#17498,#17499,#17500,#17501,#17502));
#4060=EDGE_LOOP('',(#17503));
#4061=EDGE_LOOP('',(#17504,#17505,#17506,#17507,#17508,#17509,#17510,#17511,
#17512,#17513,#17514,#17515,#17516,#17517,#17518,#17519,#17520,#17521,#17522,
#17523,#17524,#17525,#17526,#17527,#17528,#17529,#17530,#17531,#17532,#17533,
#17534,#17535,#17536,#17537,#17538,#17539,#17540,#17541,#17542,#17543,#17544,
#17545,#17546,#17547,#17548,#17549,#17550,#17551,#17552,#17553,#17554,#17555,
#17556,#17557,#17558,#17559,#17560,#17561,#17562,#17563,#17564,#17565,#17566,
#17567,#17568,#17569,#17570,#17571,#17572,#17573,#17574,#17575,#17576,#17577,
#17578,#17579,#17580,#17581,#17582,#17583,#17584,#17585,#17586,#17587,#17588,
#17589,#17590,#17591,#17592,#17593,#17594,#17595,#17596,#17597,#17598,#17599,
#17600,#17601,#17602,#17603,#17604,#17605,#17606,#17607,#17608,#17609,#17610,
#17611));
#4062=EDGE_LOOP('',(#17612,#17613,#17614,#17615,#17616));
#4063=EDGE_LOOP('',(#17617,#17618,#17619,#17620,#17621));
#4064=EDGE_LOOP('',(#17622));
#4065=EDGE_LOOP('',(#17623,#17624,#17625,#17626,#17627,#17628,#17629,#17630,
#17631,#17632,#17633,#17634,#17635,#17636,#17637,#17638,#17639,#17640,#17641,
#17642,#17643,#17644,#17645,#17646,#17647,#17648,#17649,#17650,#17651,#17652,
#17653,#17654,#17655,#17656,#17657,#17658,#17659,#17660,#17661,#17662,#17663,
#17664,#17665,#17666,#17667,#17668,#17669,#17670,#17671,#17672,#17673,#17674,
#17675,#17676,#17677,#17678,#17679,#17680,#17681,#17682,#17683,#17684,#17685,
#17686,#17687,#17688,#17689,#17690,#17691,#17692,#17693,#17694,#17695,#17696,
#17697,#17698,#17699,#17700,#17701,#17702,#17703,#17704,#17705,#17706,#17707,
#17708,#17709,#17710,#17711,#17712,#17713,#17714,#17715,#17716,#17717,#17718,
#17719,#17720,#17721,#17722,#17723,#17724,#17725,#17726,#17727,#17728,#17729,
#17730));
#4066=EDGE_LOOP('',(#17731,#17732,#17733,#17734,#17735));
#4067=EDGE_LOOP('',(#17736));
#4068=EDGE_LOOP('',(#17737,#17738,#17739,#17740));
#4069=EDGE_LOOP('',(#17741,#17742,#17743,#17744));
#4070=EDGE_LOOP('',(#17745));
#4071=EDGE_LOOP('',(#17746));
#4072=EDGE_LOOP('',(#17747,#17748,#17749,#17750));
#4073=EDGE_LOOP('',(#17751,#17752,#17753,#17754));
#4074=EDGE_LOOP('',(#17755));
#4075=EDGE_LOOP('',(#17756));
#4076=EDGE_LOOP('',(#17757,#17758,#17759,#17760));
#4077=EDGE_LOOP('',(#17761,#17762,#17763,#17764));
#4078=EDGE_LOOP('',(#17765));
#4079=EDGE_LOOP('',(#17766,#17767,#17768,#17769));
#4080=EDGE_LOOP('',(#17770,#17771,#17772,#17773));
#4081=EDGE_LOOP('',(#17774,#17775,#17776,#17777));
#4082=EDGE_LOOP('',(#17778,#17779,#17780,#17781));
#4083=EDGE_LOOP('',(#17782,#17783,#17784,#17785));
#4084=EDGE_LOOP('',(#17786,#17787,#17788,#17789));
#4085=EDGE_LOOP('',(#17790,#17791,#17792,#17793));
#4086=EDGE_LOOP('',(#17794,#17795,#17796,#17797));
#4087=EDGE_LOOP('',(#17798,#17799,#17800,#17801));
#4088=EDGE_LOOP('',(#17802,#17803,#17804,#17805));
#4089=EDGE_LOOP('',(#17806,#17807,#17808,#17809));
#4090=EDGE_LOOP('',(#17810,#17811,#17812,#17813));
#4091=EDGE_LOOP('',(#17814,#17815,#17816,#17817));
#4092=EDGE_LOOP('',(#17818,#17819,#17820,#17821));
#4093=EDGE_LOOP('',(#17822,#17823,#17824,#17825));
#4094=EDGE_LOOP('',(#17826,#17827,#17828,#17829));
#4095=EDGE_LOOP('',(#17830,#17831,#17832,#17833));
#4096=EDGE_LOOP('',(#17834,#17835,#17836,#17837));
#4097=EDGE_LOOP('',(#17838,#17839,#17840,#17841));
#4098=EDGE_LOOP('',(#17842,#17843,#17844,#17845));
#4099=EDGE_LOOP('',(#17846,#17847,#17848,#17849));
#4100=EDGE_LOOP('',(#17850,#17851,#17852,#17853));
#4101=EDGE_LOOP('',(#17854,#17855,#17856,#17857));
#4102=EDGE_LOOP('',(#17858,#17859,#17860,#17861));
#4103=EDGE_LOOP('',(#17862,#17863,#17864,#17865));
#4104=EDGE_LOOP('',(#17866,#17867,#17868,#17869));
#4105=EDGE_LOOP('',(#17870,#17871,#17872,#17873));
#4106=EDGE_LOOP('',(#17874,#17875,#17876,#17877));
#4107=EDGE_LOOP('',(#17878,#17879,#17880,#17881));
#4108=EDGE_LOOP('',(#17882,#17883,#17884,#17885));
#4109=EDGE_LOOP('',(#17886,#17887,#17888,#17889));
#4110=EDGE_LOOP('',(#17890,#17891,#17892,#17893));
#4111=EDGE_LOOP('',(#17894,#17895,#17896,#17897));
#4112=EDGE_LOOP('',(#17898,#17899,#17900,#17901));
#4113=EDGE_LOOP('',(#17902,#17903,#17904,#17905));
#4114=EDGE_LOOP('',(#17906,#17907,#17908,#17909));
#4115=EDGE_LOOP('',(#17910,#17911,#17912,#17913));
#4116=EDGE_LOOP('',(#17914,#17915,#17916,#17917));
#4117=EDGE_LOOP('',(#17918,#17919,#17920,#17921));
#4118=EDGE_LOOP('',(#17922,#17923,#17924,#17925));
#4119=EDGE_LOOP('',(#17926,#17927,#17928,#17929));
#4120=EDGE_LOOP('',(#17930,#17931,#17932,#17933));
#4121=EDGE_LOOP('',(#17934,#17935,#17936,#17937));
#4122=EDGE_LOOP('',(#17938,#17939,#17940,#17941));
#4123=EDGE_LOOP('',(#17942,#17943,#17944,#17945));
#4124=EDGE_LOOP('',(#17946,#17947,#17948,#17949));
#4125=EDGE_LOOP('',(#17950,#17951,#17952,#17953));
#4126=EDGE_LOOP('',(#17954,#17955,#17956,#17957));
#4127=EDGE_LOOP('',(#17958,#17959,#17960,#17961));
#4128=EDGE_LOOP('',(#17962,#17963,#17964,#17965));
#4129=EDGE_LOOP('',(#17966,#17967,#17968,#17969));
#4130=EDGE_LOOP('',(#17970,#17971,#17972,#17973));
#4131=EDGE_LOOP('',(#17974,#17975,#17976,#17977));
#4132=EDGE_LOOP('',(#17978,#17979,#17980,#17981));
#4133=EDGE_LOOP('',(#17982,#17983,#17984,#17985));
#4134=EDGE_LOOP('',(#17986,#17987,#17988,#17989));
#4135=EDGE_LOOP('',(#17990,#17991,#17992,#17993));
#4136=EDGE_LOOP('',(#17994,#17995,#17996,#17997));
#4137=EDGE_LOOP('',(#17998,#17999,#18000,#18001));
#4138=EDGE_LOOP('',(#18002,#18003,#18004,#18005));
#4139=EDGE_LOOP('',(#18006,#18007,#18008,#18009));
#4140=EDGE_LOOP('',(#18010,#18011,#18012,#18013));
#4141=EDGE_LOOP('',(#18014,#18015,#18016,#18017));
#4142=EDGE_LOOP('',(#18018,#18019,#18020,#18021));
#4143=EDGE_LOOP('',(#18022,#18023,#18024,#18025));
#4144=EDGE_LOOP('',(#18026,#18027,#18028,#18029));
#4145=EDGE_LOOP('',(#18030,#18031,#18032,#18033));
#4146=EDGE_LOOP('',(#18034,#18035,#18036,#18037));
#4147=EDGE_LOOP('',(#18038,#18039,#18040,#18041));
#4148=EDGE_LOOP('',(#18042,#18043,#18044,#18045));
#4149=EDGE_LOOP('',(#18046,#18047,#18048,#18049));
#4150=EDGE_LOOP('',(#18050,#18051,#18052,#18053));
#4151=EDGE_LOOP('',(#18054,#18055,#18056,#18057));
#4152=EDGE_LOOP('',(#18058,#18059,#18060,#18061));
#4153=EDGE_LOOP('',(#18062,#18063,#18064,#18065));
#4154=EDGE_LOOP('',(#18066,#18067,#18068,#18069));
#4155=EDGE_LOOP('',(#18070,#18071,#18072,#18073));
#4156=EDGE_LOOP('',(#18074,#18075,#18076,#18077));
#4157=EDGE_LOOP('',(#18078,#18079,#18080,#18081));
#4158=EDGE_LOOP('',(#18082,#18083,#18084,#18085));
#4159=EDGE_LOOP('',(#18086,#18087,#18088,#18089));
#4160=EDGE_LOOP('',(#18090,#18091,#18092,#18093));
#4161=EDGE_LOOP('',(#18094,#18095,#18096,#18097));
#4162=EDGE_LOOP('',(#18098,#18099,#18100,#18101));
#4163=EDGE_LOOP('',(#18102,#18103,#18104,#18105));
#4164=EDGE_LOOP('',(#18106,#18107,#18108,#18109));
#4165=EDGE_LOOP('',(#18110,#18111,#18112,#18113));
#4166=EDGE_LOOP('',(#18114,#18115,#18116,#18117));
#4167=EDGE_LOOP('',(#18118,#18119,#18120,#18121));
#4168=EDGE_LOOP('',(#18122,#18123,#18124,#18125));
#4169=EDGE_LOOP('',(#18126,#18127,#18128,#18129));
#4170=EDGE_LOOP('',(#18130,#18131,#18132,#18133));
#4171=EDGE_LOOP('',(#18134,#18135,#18136,#18137));
#4172=EDGE_LOOP('',(#18138,#18139,#18140,#18141));
#4173=EDGE_LOOP('',(#18142,#18143,#18144,#18145));
#4174=EDGE_LOOP('',(#18146,#18147,#18148,#18149));
#4175=EDGE_LOOP('',(#18150,#18151,#18152,#18153));
#4176=EDGE_LOOP('',(#18154,#18155,#18156,#18157));
#4177=EDGE_LOOP('',(#18158,#18159,#18160,#18161));
#4178=EDGE_LOOP('',(#18162,#18163,#18164,#18165));
#4179=EDGE_LOOP('',(#18166,#18167,#18168,#18169));
#4180=EDGE_LOOP('',(#18170,#18171,#18172,#18173));
#4181=EDGE_LOOP('',(#18174,#18175,#18176,#18177));
#4182=EDGE_LOOP('',(#18178,#18179,#18180,#18181));
#4183=EDGE_LOOP('',(#18182,#18183,#18184,#18185));
#4184=EDGE_LOOP('',(#18186,#18187,#18188,#18189));
#4185=EDGE_LOOP('',(#18190,#18191,#18192,#18193));
#4186=EDGE_LOOP('',(#18194,#18195,#18196,#18197));
#5630=LINE('',#35354,#8127);
#5631=LINE('',#35417,#8128);
#5632=LINE('',#35421,#8129);
#5633=LINE('',#35481,#8130);
#5634=LINE('',#35485,#8131);
#5635=LINE('',#35507,#8132);
#5636=LINE('',#35511,#8133);
#5637=LINE('',#35533,#8134);
#5638=LINE('',#35537,#8135);
#5639=LINE('',#35597,#8136);
#5640=LINE('',#35601,#8137);
#5641=LINE('',#35661,#8138);
#5642=LINE('',#35665,#8139);
#5643=LINE('',#35725,#8140);
#5644=LINE('',#35729,#8141);
#5645=LINE('',#35789,#8142);
#5646=LINE('',#35793,#8143);
#5647=LINE('',#35853,#8144);
#5648=LINE('',#35857,#8145);
#5649=LINE('',#35877,#8146);
#5650=LINE('',#35881,#8147);
#5651=LINE('',#35903,#8148);
#5652=LINE('',#35907,#8149);
#5653=LINE('',#35967,#8150);
#5654=LINE('',#35971,#8151);
#5655=LINE('',#36031,#8152);
#5656=LINE('',#36035,#8153);
#5657=LINE('',#36095,#8154);
#5658=LINE('',#36099,#8155);
#5659=LINE('',#36159,#8156);
#5660=LINE('',#36163,#8157);
#5661=LINE('',#36223,#8158);
#5662=LINE('',#36227,#8159);
#5663=LINE('',#36287,#8160);
#5664=LINE('',#36291,#8161);
#5665=LINE('',#36351,#8162);
#5666=LINE('',#36354,#8163);
#5667=LINE('',#36358,#8164);
#5668=LINE('',#36363,#8165);
#5669=LINE('',#36417,#8166);
#5670=LINE('',#36421,#8167);
#5671=LINE('',#36481,#8168);
#5672=LINE('',#36485,#8169);
#5673=LINE('',#36545,#8170);
#5674=LINE('',#36549,#8171);
#5675=LINE('',#36609,#8172);
#5676=LINE('',#36613,#8173);
#5677=LINE('',#36635,#8174);
#5678=LINE('',#36639,#8175);
#5679=LINE('',#36699,#8176);
#5680=LINE('',#36703,#8177);
#5681=LINE('',#36763,#8178);
#5682=LINE('',#36767,#8179);
#5683=LINE('',#36827,#8180);
#5684=LINE('',#36831,#8181);
#5685=LINE('',#36891,#8182);
#5686=LINE('',#36895,#8183);
#5687=LINE('',#36955,#8184);
#5688=LINE('',#36959,#8185);
#5689=LINE('',#36981,#8186);
#5690=LINE('',#36985,#8187);
#5691=LINE('',#37045,#8188);
#5692=LINE('',#37049,#8189);
#5693=LINE('',#37109,#8190);
#5694=LINE('',#37113,#8191);
#5695=LINE('',#37173,#8192);
#5696=LINE('',#37177,#8193);
#5697=LINE('',#37199,#8194);
#5698=LINE('',#37203,#8195);
#5699=LINE('',#37263,#8196);
#5700=LINE('',#37267,#8197);
#5701=LINE('',#37327,#8198);
#5702=LINE('',#37331,#8199);
#5703=LINE('',#37391,#8200);
#5704=LINE('',#37395,#8201);
#5705=LINE('',#37408,#8202);
#5706=LINE('',#37416,#8203);
#5707=LINE('',#37420,#8204);
#5708=LINE('',#37425,#8205);
#5709=LINE('',#37429,#8206);
#5710=LINE('',#37436,#8207);
#5711=LINE('',#37440,#8208);
#5712=LINE('',#37512,#8209);
#5713=LINE('',#37520,#8210);
#5714=LINE('',#37521,#8211);
#5715=LINE('',#37599,#8212);
#5716=LINE('',#37671,#8213);
#5717=LINE('',#37679,#8214);
#5718=LINE('',#37680,#8215);
#5719=LINE('',#37758,#8216);
#5720=LINE('',#37830,#8217);
#5721=LINE('',#37838,#8218);
#5722=LINE('',#37839,#8219);
#5723=LINE('',#37917,#8220);
#5724=LINE('',#37989,#8221);
#5725=LINE('',#37997,#8222);
#5726=LINE('',#37998,#8223);
#5727=LINE('',#38076,#8224);
#5728=LINE('',#38148,#8225);
#5729=LINE('',#38156,#8226);
#5730=LINE('',#38157,#8227);
#5731=LINE('',#38235,#8228);
#5732=LINE('',#38307,#8229);
#5733=LINE('',#38315,#8230);
#5734=LINE('',#38316,#8231);
#5735=LINE('',#38394,#8232);
#5736=LINE('',#38466,#8233);
#5737=LINE('',#38474,#8234);
#5738=LINE('',#38475,#8235);
#5739=LINE('',#38553,#8236);
#5740=LINE('',#38625,#8237);
#5741=LINE('',#38633,#8238);
#5742=LINE('',#38634,#8239);
#5743=LINE('',#38712,#8240);
#5744=LINE('',#38784,#8241);
#5745=LINE('',#38792,#8242);
#5746=LINE('',#38793,#8243);
#5747=LINE('',#38871,#8244);
#5748=LINE('',#38943,#8245);
#5749=LINE('',#38951,#8246);
#5750=LINE('',#38952,#8247);
#5751=LINE('',#39030,#8248);
#5752=LINE('',#39102,#8249);
#5753=LINE('',#39110,#8250);
#5754=LINE('',#39111,#8251);
#5755=LINE('',#39189,#8252);
#5756=LINE('',#39261,#8253);
#5757=LINE('',#39269,#8254);
#5758=LINE('',#39270,#8255);
#5759=LINE('',#39348,#8256);
#5760=LINE('',#39420,#8257);
#5761=LINE('',#39428,#8258);
#5762=LINE('',#39429,#8259);
#5763=LINE('',#39507,#8260);
#5764=LINE('',#39579,#8261);
#5765=LINE('',#39587,#8262);
#5766=LINE('',#39588,#8263);
#5767=LINE('',#39666,#8264);
#5768=LINE('',#39738,#8265);
#5769=LINE('',#39746,#8266);
#5770=LINE('',#39747,#8267);
#5771=LINE('',#39825,#8268);
#5772=LINE('',#39897,#8269);
#5773=LINE('',#39905,#8270);
#5774=LINE('',#39906,#8271);
#5775=LINE('',#39984,#8272);
#5776=LINE('',#40056,#8273);
#5777=LINE('',#40064,#8274);
#5778=LINE('',#40065,#8275);
#5779=LINE('',#40143,#8276);
#5780=LINE('',#40215,#8277);
#5781=LINE('',#40223,#8278);
#5782=LINE('',#40224,#8279);
#5783=LINE('',#40302,#8280);
#8127=VECTOR('',#28995,6.175);
#8128=VECTOR('',#29002,1.);
#8129=VECTOR('',#29005,1.);
#8130=VECTOR('',#29008,1.);
#8131=VECTOR('',#29011,1.);
#8132=VECTOR('',#29014,1.);
#8133=VECTOR('',#29017,1.);
#8134=VECTOR('',#29020,1.);
#8135=VECTOR('',#29023,1.);
#8136=VECTOR('',#29026,1.);
#8137=VECTOR('',#29029,1.);
#8138=VECTOR('',#29032,1.);
#8139=VECTOR('',#29035,1.);
#8140=VECTOR('',#29038,1.);
#8141=VECTOR('',#29041,1.);
#8142=VECTOR('',#29044,1.);
#8143=VECTOR('',#29047,1.);
#8144=VECTOR('',#29050,1.);
#8145=VECTOR('',#29053,1.);
#8146=VECTOR('',#29056,1.);
#8147=VECTOR('',#29059,1.);
#8148=VECTOR('',#29062,1.);
#8149=VECTOR('',#29065,1.);
#8150=VECTOR('',#29068,1.);
#8151=VECTOR('',#29071,1.);
#8152=VECTOR('',#29074,1.);
#8153=VECTOR('',#29077,1.);
#8154=VECTOR('',#29080,1.);
#8155=VECTOR('',#29083,1.);
#8156=VECTOR('',#29086,1.);
#8157=VECTOR('',#29089,1.);
#8158=VECTOR('',#29092,1.);
#8159=VECTOR('',#29095,1.);
#8160=VECTOR('',#29098,1.);
#8161=VECTOR('',#29101,1.);
#8162=VECTOR('',#29104,1.);
#8163=VECTOR('',#29107,1.);
#8164=VECTOR('',#29112,6.25);
#8165=VECTOR('',#29117,6.175);
#8166=VECTOR('',#29124,1.);
#8167=VECTOR('',#29127,1.);
#8168=VECTOR('',#29130,1.);
#8169=VECTOR('',#29133,1.);
#8170=VECTOR('',#29136,1.);
#8171=VECTOR('',#29139,1.);
#8172=VECTOR('',#29142,1.);
#8173=VECTOR('',#29145,1.);
#8174=VECTOR('',#29148,1.);
#8175=VECTOR('',#29151,1.);
#8176=VECTOR('',#29154,1.);
#8177=VECTOR('',#29157,1.);
#8178=VECTOR('',#29160,1.);
#8179=VECTOR('',#29163,1.);
#8180=VECTOR('',#29166,1.);
#8181=VECTOR('',#29169,1.);
#8182=VECTOR('',#29172,1.);
#8183=VECTOR('',#29175,1.);
#8184=VECTOR('',#29178,1.);
#8185=VECTOR('',#29181,1.);
#8186=VECTOR('',#29184,1.);
#8187=VECTOR('',#29187,1.);
#8188=VECTOR('',#29190,1.);
#8189=VECTOR('',#29193,1.);
#8190=VECTOR('',#29196,1.);
#8191=VECTOR('',#29199,1.);
#8192=VECTOR('',#29202,1.);
#8193=VECTOR('',#29205,1.);
#8194=VECTOR('',#29208,1.);
#8195=VECTOR('',#29211,1.);
#8196=VECTOR('',#29214,1.);
#8197=VECTOR('',#29217,1.);
#8198=VECTOR('',#29220,1.);
#8199=VECTOR('',#29223,1.);
#8200=VECTOR('',#29226,1.);
#8201=VECTOR('',#29229,1.);
#8202=VECTOR('',#29234,6.25);
#8203=VECTOR('',#29245,2.95);
#8204=VECTOR('',#29250,3.);
#8205=VECTOR('',#29257,6.175);
#8206=VECTOR('',#29262,6.175);
#8207=VECTOR('',#29271,3.);
#8208=VECTOR('',#29276,2.95);
#8209=VECTOR('',#29279,1.);
#8210=VECTOR('',#29282,1.);
#8211=VECTOR('',#29283,1.);
#8212=VECTOR('',#29286,1.);
#8213=VECTOR('',#29289,1.);
#8214=VECTOR('',#29292,1.);
#8215=VECTOR('',#29293,1.);
#8216=VECTOR('',#29296,1.);
#8217=VECTOR('',#29299,1.);
#8218=VECTOR('',#29302,1.);
#8219=VECTOR('',#29303,1.);
#8220=VECTOR('',#29306,1.);
#8221=VECTOR('',#29309,1.);
#8222=VECTOR('',#29312,1.);
#8223=VECTOR('',#29313,1.);
#8224=VECTOR('',#29316,1.);
#8225=VECTOR('',#29319,1.);
#8226=VECTOR('',#29322,1.);
#8227=VECTOR('',#29323,1.);
#8228=VECTOR('',#29326,1.);
#8229=VECTOR('',#29329,1.);
#8230=VECTOR('',#29332,1.);
#8231=VECTOR('',#29333,1.);
#8232=VECTOR('',#29336,1.);
#8233=VECTOR('',#29339,1.);
#8234=VECTOR('',#29342,1.);
#8235=VECTOR('',#29343,1.);
#8236=VECTOR('',#29346,1.);
#8237=VECTOR('',#29349,1.);
#8238=VECTOR('',#29352,1.);
#8239=VECTOR('',#29353,1.);
#8240=VECTOR('',#29356,1.);
#8241=VECTOR('',#29359,1.);
#8242=VECTOR('',#29362,1.);
#8243=VECTOR('',#29363,1.);
#8244=VECTOR('',#29366,1.);
#8245=VECTOR('',#29369,1.);
#8246=VECTOR('',#29372,1.);
#8247=VECTOR('',#29373,1.);
#8248=VECTOR('',#29376,1.);
#8249=VECTOR('',#29379,1.);
#8250=VECTOR('',#29382,1.);
#8251=VECTOR('',#29383,1.);
#8252=VECTOR('',#29386,1.);
#8253=VECTOR('',#29389,1.);
#8254=VECTOR('',#29392,1.);
#8255=VECTOR('',#29393,1.);
#8256=VECTOR('',#29396,1.);
#8257=VECTOR('',#29399,1.);
#8258=VECTOR('',#29402,1.);
#8259=VECTOR('',#29403,1.);
#8260=VECTOR('',#29406,1.);
#8261=VECTOR('',#29409,1.);
#8262=VECTOR('',#29412,1.);
#8263=VECTOR('',#29413,1.);
#8264=VECTOR('',#29416,1.);
#8265=VECTOR('',#29419,1.);
#8266=VECTOR('',#29422,1.);
#8267=VECTOR('',#29423,1.);
#8268=VECTOR('',#29426,1.);
#8269=VECTOR('',#29429,1.);
#8270=VECTOR('',#29432,1.);
#8271=VECTOR('',#29433,1.);
#8272=VECTOR('',#29436,1.);
#8273=VECTOR('',#29439,1.);
#8274=VECTOR('',#29442,1.);
#8275=VECTOR('',#29443,1.);
#8276=VECTOR('',#29446,1.);
#8277=VECTOR('',#29449,1.);
#8278=VECTOR('',#29452,1.);
#8279=VECTOR('',#29453,1.);
#8280=VECTOR('',#29456,1.);
#10624=CIRCLE('',#27056,6.25);
#10625=CIRCLE('',#27057,6.25);
#10626=CIRCLE('',#27058,6.1);
#10627=CIRCLE('',#27060,6.);
#10628=CIRCLE('',#27061,4.6500000000004);
#10629=CIRCLE('',#27062,6.);
#10630=CIRCLE('',#27063,4.64999999999896);
#10631=CIRCLE('',#27064,6.);
#10632=CIRCLE('',#27065,4.64999999999943);
#10633=CIRCLE('',#27066,6.);
#10634=CIRCLE('',#27067,4.64999999999968);
#10635=CIRCLE('',#27068,6.);
#10636=CIRCLE('',#27069,4.64999999999985);
#10637=CIRCLE('',#27070,6.);
#10638=CIRCLE('',#27071,4.64999999999964);
#10639=CIRCLE('',#27072,6.);
#10640=CIRCLE('',#27073,4.65000000000067);
#10641=CIRCLE('',#27074,6.);
#10642=CIRCLE('',#27075,4.64999999999845);
#10643=CIRCLE('',#27076,6.);
#10644=CIRCLE('',#27077,4.65000000000029);
#10645=CIRCLE('',#27078,6.);
#10646=CIRCLE('',#27079,4.65000000000076);
#10647=CIRCLE('',#27080,6.);
#10648=CIRCLE('',#27081,4.64999999999928);
#10649=CIRCLE('',#27082,6.);
#10650=CIRCLE('',#27083,4.6499999999995);
#10651=CIRCLE('',#27084,6.);
#10652=CIRCLE('',#27085,4.64999999999968);
#10653=CIRCLE('',#27086,6.);
#10654=CIRCLE('',#27087,4.64999999999985);
#10655=CIRCLE('',#27088,6.);
#10656=CIRCLE('',#27089,4.6500000000015);
#10657=CIRCLE('',#27090,6.);
#10658=CIRCLE('',#27091,4.65000000000067);
#10659=CIRCLE('',#27092,6.);
#10660=CIRCLE('',#27093,4.64999999999896);
#10661=CIRCLE('',#27094,6.);
#10662=CIRCLE('',#27095,4.65000000000016);
#10663=CIRCLE('',#27097,6.25);
#10664=CIRCLE('',#27099,6.1);
#10665=CIRCLE('',#27100,6.25);
#10666=CIRCLE('',#27101,6.25);
#10667=CIRCLE('',#27103,4.65000000000016);
#10668=CIRCLE('',#27104,6.);
#10669=CIRCLE('',#27105,4.64999999999896);
#10670=CIRCLE('',#27106,6.);
#10671=CIRCLE('',#27107,4.65000000000067);
#10672=CIRCLE('',#27108,6.);
#10673=CIRCLE('',#27109,4.6500000000015);
#10674=CIRCLE('',#27110,6.);
#10675=CIRCLE('',#27111,4.64999999999985);
#10676=CIRCLE('',#27112,6.);
#10677=CIRCLE('',#27113,4.64999999999968);
#10678=CIRCLE('',#27114,6.);
#10679=CIRCLE('',#27115,4.6499999999995);
#10680=CIRCLE('',#27116,6.);
#10681=CIRCLE('',#27117,4.64999999999928);
#10682=CIRCLE('',#27118,6.);
#10683=CIRCLE('',#27119,4.65000000000076);
#10684=CIRCLE('',#27120,6.);
#10685=CIRCLE('',#27121,4.65000000000029);
#10686=CIRCLE('',#27122,6.);
#10687=CIRCLE('',#27123,4.64999999999845);
#10688=CIRCLE('',#27124,6.);
#10689=CIRCLE('',#27125,4.65000000000067);
#10690=CIRCLE('',#27126,6.);
#10691=CIRCLE('',#27127,4.64999999999964);
#10692=CIRCLE('',#27128,6.);
#10693=CIRCLE('',#27129,4.64999999999985);
#10694=CIRCLE('',#27130,6.);
#10695=CIRCLE('',#27131,4.64999999999968);
#10696=CIRCLE('',#27132,6.);
#10697=CIRCLE('',#27133,4.64999999999943);
#10698=CIRCLE('',#27134,6.);
#10699=CIRCLE('',#27135,4.64999999999896);
#10700=CIRCLE('',#27136,6.);
#10701=CIRCLE('',#27137,4.6500000000004);
#10702=CIRCLE('',#27138,6.);
#10703=CIRCLE('',#27140,6.25);
#10704=CIRCLE('',#27142,2.9);
#10705=CIRCLE('',#27144,3.);
#10706=CIRCLE('',#27146,3.);
#10707=CIRCLE('',#27148,6.1);
#10708=CIRCLE('',#27151,6.1);
#10709=CIRCLE('',#27153,3.);
#10710=CIRCLE('',#27155,3.);
#10711=CIRCLE('',#27157,2.9);
#11139=VERTEX_POINT('',#35349);
#11140=VERTEX_POINT('',#35350);
#11141=VERTEX_POINT('',#35353);
#11142=VERTEX_POINT('',#35357);
#11143=VERTEX_POINT('',#35358);
#11144=VERTEX_POINT('',#35367);
#11145=VERTEX_POINT('',#35369);
#11146=VERTEX_POINT('',#35416);
#11147=VERTEX_POINT('',#35418);
#11148=VERTEX_POINT('',#35420);
#11149=VERTEX_POINT('',#35422);
#11150=VERTEX_POINT('',#35431);
#11151=VERTEX_POINT('',#35433);
#11152=VERTEX_POINT('',#35480);
#11153=VERTEX_POINT('',#35482);
#11154=VERTEX_POINT('',#35484);
#11155=VERTEX_POINT('',#35486);
#11156=VERTEX_POINT('',#35495);
#11157=VERTEX_POINT('',#35497);
#11158=VERTEX_POINT('',#35506);
#11159=VERTEX_POINT('',#35508);
#11160=VERTEX_POINT('',#35510);
#11161=VERTEX_POINT('',#35512);
#11162=VERTEX_POINT('',#35521);
#11163=VERTEX_POINT('',#35523);
#11164=VERTEX_POINT('',#35532);
#11165=VERTEX_POINT('',#35534);
#11166=VERTEX_POINT('',#35536);
#11167=VERTEX_POINT('',#35538);
#11168=VERTEX_POINT('',#35547);
#11169=VERTEX_POINT('',#35549);
#11170=VERTEX_POINT('',#35596);
#11171=VERTEX_POINT('',#35598);
#11172=VERTEX_POINT('',#35600);
#11173=VERTEX_POINT('',#35602);
#11174=VERTEX_POINT('',#35611);
#11175=VERTEX_POINT('',#35613);
#11176=VERTEX_POINT('',#35660);
#11177=VERTEX_POINT('',#35662);
#11178=VERTEX_POINT('',#35664);
#11179=VERTEX_POINT('',#35666);
#11180=VERTEX_POINT('',#35675);
#11181=VERTEX_POINT('',#35677);
#11182=VERTEX_POINT('',#35724);
#11183=VERTEX_POINT('',#35726);
#11184=VERTEX_POINT('',#35728);
#11185=VERTEX_POINT('',#35730);
#11186=VERTEX_POINT('',#35739);
#11187=VERTEX_POINT('',#35741);
#11188=VERTEX_POINT('',#35788);
#11189=VERTEX_POINT('',#35790);
#11190=VERTEX_POINT('',#35792);
#11191=VERTEX_POINT('',#35794);
#11192=VERTEX_POINT('',#35803);
#11193=VERTEX_POINT('',#35805);
#11194=VERTEX_POINT('',#35852);
#11195=VERTEX_POINT('',#35854);
#11196=VERTEX_POINT('',#35856);
#11197=VERTEX_POINT('',#35858);
#11198=VERTEX_POINT('',#35867);
#11199=VERTEX_POINT('',#35869);
#11200=VERTEX_POINT('',#35876);
#11201=VERTEX_POINT('',#35878);
#11202=VERTEX_POINT('',#35880);
#11203=VERTEX_POINT('',#35882);
#11204=VERTEX_POINT('',#35891);
#11205=VERTEX_POINT('',#35893);
#11206=VERTEX_POINT('',#35902);
#11207=VERTEX_POINT('',#35904);
#11208=VERTEX_POINT('',#35906);
#11209=VERTEX_POINT('',#35908);
#11210=VERTEX_POINT('',#35917);
#11211=VERTEX_POINT('',#35919);
#11212=VERTEX_POINT('',#35966);
#11213=VERTEX_POINT('',#35968);
#11214=VERTEX_POINT('',#35970);
#11215=VERTEX_POINT('',#35972);
#11216=VERTEX_POINT('',#35981);
#11217=VERTEX_POINT('',#35983);
#11218=VERTEX_POINT('',#36030);
#11219=VERTEX_POINT('',#36032);
#11220=VERTEX_POINT('',#36034);
#11221=VERTEX_POINT('',#36036);
#11222=VERTEX_POINT('',#36045);
#11223=VERTEX_POINT('',#36047);
#11224=VERTEX_POINT('',#36094);
#11225=VERTEX_POINT('',#36096);
#11226=VERTEX_POINT('',#36098);
#11227=VERTEX_POINT('',#36100);
#11228=VERTEX_POINT('',#36109);
#11229=VERTEX_POINT('',#36111);
#11230=VERTEX_POINT('',#36158);
#11231=VERTEX_POINT('',#36160);
#11232=VERTEX_POINT('',#36162);
#11233=VERTEX_POINT('',#36164);
#11234=VERTEX_POINT('',#36173);
#11235=VERTEX_POINT('',#36175);
#11236=VERTEX_POINT('',#36222);
#11237=VERTEX_POINT('',#36224);
#11238=VERTEX_POINT('',#36226);
#11239=VERTEX_POINT('',#36228);
#11240=VERTEX_POINT('',#36237);
#11241=VERTEX_POINT('',#36239);
#11242=VERTEX_POINT('',#36286);
#11243=VERTEX_POINT('',#36288);
#11244=VERTEX_POINT('',#36290);
#11245=VERTEX_POINT('',#36292);
#11246=VERTEX_POINT('',#36301);
#11247=VERTEX_POINT('',#36303);
#11248=VERTEX_POINT('',#36350);
#11249=VERTEX_POINT('',#36352);
#11250=VERTEX_POINT('',#36356);
#11251=VERTEX_POINT('',#36360);
#11252=VERTEX_POINT('',#36362);
#11253=VERTEX_POINT('',#36364);
#11254=VERTEX_POINT('',#36368);
#11255=VERTEX_POINT('',#36369);
#11256=VERTEX_POINT('',#36416);
#11257=VERTEX_POINT('',#36418);
#11258=VERTEX_POINT('',#36420);
#11259=VERTEX_POINT('',#36422);
#11260=VERTEX_POINT('',#36431);
#11261=VERTEX_POINT('',#36433);
#11262=VERTEX_POINT('',#36480);
#11263=VERTEX_POINT('',#36482);
#11264=VERTEX_POINT('',#36484);
#11265=VERTEX_POINT('',#36486);
#11266=VERTEX_POINT('',#36495);
#11267=VERTEX_POINT('',#36497);
#11268=VERTEX_POINT('',#36544);
#11269=VERTEX_POINT('',#36546);
#11270=VERTEX_POINT('',#36548);
#11271=VERTEX_POINT('',#36550);
#11272=VERTEX_POINT('',#36559);
#11273=VERTEX_POINT('',#36561);
#11274=VERTEX_POINT('',#36608);
#11275=VERTEX_POINT('',#36610);
#11276=VERTEX_POINT('',#36612);
#11277=VERTEX_POINT('',#36614);
#11278=VERTEX_POINT('',#36623);
#11279=VERTEX_POINT('',#36625);
#11280=VERTEX_POINT('',#36634);
#11281=VERTEX_POINT('',#36636);
#11282=VERTEX_POINT('',#36638);
#11283=VERTEX_POINT('',#36640);
#11284=VERTEX_POINT('',#36649);
#11285=VERTEX_POINT('',#36651);
#11286=VERTEX_POINT('',#36698);
#11287=VERTEX_POINT('',#36700);
#11288=VERTEX_POINT('',#36702);
#11289=VERTEX_POINT('',#36704);
#11290=VERTEX_POINT('',#36713);
#11291=VERTEX_POINT('',#36715);
#11292=VERTEX_POINT('',#36762);
#11293=VERTEX_POINT('',#36764);
#11294=VERTEX_POINT('',#36766);
#11295=VERTEX_POINT('',#36768);
#11296=VERTEX_POINT('',#36777);
#11297=VERTEX_POINT('',#36779);
#11298=VERTEX_POINT('',#36826);
#11299=VERTEX_POINT('',#36828);
#11300=VERTEX_POINT('',#36830);
#11301=VERTEX_POINT('',#36832);
#11302=VERTEX_POINT('',#36841);
#11303=VERTEX_POINT('',#36843);
#11304=VERTEX_POINT('',#36890);
#11305=VERTEX_POINT('',#36892);
#11306=VERTEX_POINT('',#36894);
#11307=VERTEX_POINT('',#36896);
#11308=VERTEX_POINT('',#36905);
#11309=VERTEX_POINT('',#36907);
#11310=VERTEX_POINT('',#36954);
#11311=VERTEX_POINT('',#36956);
#11312=VERTEX_POINT('',#36958);
#11313=VERTEX_POINT('',#36960);
#11314=VERTEX_POINT('',#36969);
#11315=VERTEX_POINT('',#36971);
#11316=VERTEX_POINT('',#36980);
#11317=VERTEX_POINT('',#36982);
#11318=VERTEX_POINT('',#36984);
#11319=VERTEX_POINT('',#36986);
#11320=VERTEX_POINT('',#36995);
#11321=VERTEX_POINT('',#36997);
#11322=VERTEX_POINT('',#37044);
#11323=VERTEX_POINT('',#37046);
#11324=VERTEX_POINT('',#37048);
#11325=VERTEX_POINT('',#37050);
#11326=VERTEX_POINT('',#37059);
#11327=VERTEX_POINT('',#37061);
#11328=VERTEX_POINT('',#37108);
#11329=VERTEX_POINT('',#37110);
#11330=VERTEX_POINT('',#37112);
#11331=VERTEX_POINT('',#37114);
#11332=VERTEX_POINT('',#37123);
#11333=VERTEX_POINT('',#37125);
#11334=VERTEX_POINT('',#37172);
#11335=VERTEX_POINT('',#37174);
#11336=VERTEX_POINT('',#37176);
#11337=VERTEX_POINT('',#37178);
#11338=VERTEX_POINT('',#37187);
#11339=VERTEX_POINT('',#37189);
#11340=VERTEX_POINT('',#37198);
#11341=VERTEX_POINT('',#37200);
#11342=VERTEX_POINT('',#37202);
#11343=VERTEX_POINT('',#37204);
#11344=VERTEX_POINT('',#37213);
#11345=VERTEX_POINT('',#37215);
#11346=VERTEX_POINT('',#37262);
#11347=VERTEX_POINT('',#37264);
#11348=VERTEX_POINT('',#37266);
#11349=VERTEX_POINT('',#37268);
#11350=VERTEX_POINT('',#37277);
#11351=VERTEX_POINT('',#37279);
#11352=VERTEX_POINT('',#37326);
#11353=VERTEX_POINT('',#37328);
#11354=VERTEX_POINT('',#37330);
#11355=VERTEX_POINT('',#37332);
#11356=VERTEX_POINT('',#37341);
#11357=VERTEX_POINT('',#37343);
#11358=VERTEX_POINT('',#37390);
#11359=VERTEX_POINT('',#37392);
#11360=VERTEX_POINT('',#37394);
#11361=VERTEX_POINT('',#37396);
#11362=VERTEX_POINT('',#37407);
#11363=VERTEX_POINT('',#37411);
#11364=VERTEX_POINT('',#37414);
#11365=VERTEX_POINT('',#37418);
#11366=VERTEX_POINT('',#37422);
#11367=VERTEX_POINT('',#37427);
#11368=VERTEX_POINT('',#37431);
#11369=VERTEX_POINT('',#37434);
#11370=VERTEX_POINT('',#37438);
#13602=EDGE_CURVE('',#11139,#11140,#10624,.T.);
#13603=EDGE_CURVE('',#11140,#11139,#10625,.T.);
#13604=EDGE_CURVE('',#11139,#11141,#5630,.T.);
#13605=EDGE_CURVE('',#11141,#11141,#10626,.T.);
#13606=EDGE_CURVE('',#11142,#11143,#927,.T.);
#13607=EDGE_CURVE('',#11143,#11144,#10627,.T.);
#13608=EDGE_CURVE('',#11144,#11145,#928,.T.);
#13609=EDGE_CURVE('',#11145,#11146,#5631,.T.);
#13610=EDGE_CURVE('',#11146,#11147,#10628,.T.);
#13611=EDGE_CURVE('',#11147,#11148,#5632,.T.);
#13612=EDGE_CURVE('',#11148,#11149,#929,.T.);
#13613=EDGE_CURVE('',#11149,#11150,#10629,.T.);
#13614=EDGE_CURVE('',#11150,#11151,#930,.T.);
#13615=EDGE_CURVE('',#11151,#11152,#5633,.T.);
#13616=EDGE_CURVE('',#11152,#11153,#10630,.T.);
#13617=EDGE_CURVE('',#11153,#11154,#5634,.T.);
#13618=EDGE_CURVE('',#11154,#11155,#931,.T.);
#13619=EDGE_CURVE('',#11155,#11156,#10631,.T.);
#13620=EDGE_CURVE('',#11156,#11157,#932,.T.);
#13621=EDGE_CURVE('',#11157,#11158,#5635,.T.);
#13622=EDGE_CURVE('',#11158,#11159,#10632,.T.);
#13623=EDGE_CURVE('',#11159,#11160,#5636,.T.);
#13624=EDGE_CURVE('',#11160,#11161,#933,.T.);
#13625=EDGE_CURVE('',#11161,#11162,#10633,.T.);
#13626=EDGE_CURVE('',#11162,#11163,#934,.T.);
#13627=EDGE_CURVE('',#11163,#11164,#5637,.T.);
#13628=EDGE_CURVE('',#11164,#11165,#10634,.T.);
#13629=EDGE_CURVE('',#11165,#11166,#5638,.T.);
#13630=EDGE_CURVE('',#11166,#11167,#935,.T.);
#13631=EDGE_CURVE('',#11167,#11168,#10635,.T.);
#13632=EDGE_CURVE('',#11168,#11169,#936,.T.);
#13633=EDGE_CURVE('',#11169,#11170,#5639,.T.);
#13634=EDGE_CURVE('',#11170,#11171,#10636,.T.);
#13635=EDGE_CURVE('',#11171,#11172,#5640,.T.);
#13636=EDGE_CURVE('',#11172,#11173,#937,.T.);
#13637=EDGE_CURVE('',#11173,#11174,#10637,.T.);
#13638=EDGE_CURVE('',#11174,#11175,#938,.T.);
#13639=EDGE_CURVE('',#11175,#11176,#5641,.T.);
#13640=EDGE_CURVE('',#11176,#11177,#10638,.T.);
#13641=EDGE_CURVE('',#11177,#11178,#5642,.T.);
#13642=EDGE_CURVE('',#11178,#11179,#939,.T.);
#13643=EDGE_CURVE('',#11179,#11180,#10639,.T.);
#13644=EDGE_CURVE('',#11180,#11181,#940,.T.);
#13645=EDGE_CURVE('',#11181,#11182,#5643,.T.);
#13646=EDGE_CURVE('',#11182,#11183,#10640,.T.);
#13647=EDGE_CURVE('',#11183,#11184,#5644,.T.);
#13648=EDGE_CURVE('',#11184,#11185,#941,.T.);
#13649=EDGE_CURVE('',#11185,#11186,#10641,.T.);
#13650=EDGE_CURVE('',#11186,#11187,#942,.T.);
#13651=EDGE_CURVE('',#11187,#11188,#5645,.T.);
#13652=EDGE_CURVE('',#11188,#11189,#10642,.T.);
#13653=EDGE_CURVE('',#11189,#11190,#5646,.T.);
#13654=EDGE_CURVE('',#11190,#11191,#943,.T.);
#13655=EDGE_CURVE('',#11191,#11192,#10643,.T.);
#13656=EDGE_CURVE('',#11192,#11193,#944,.T.);
#13657=EDGE_CURVE('',#11193,#11194,#5647,.T.);
#13658=EDGE_CURVE('',#11194,#11195,#10644,.T.);
#13659=EDGE_CURVE('',#11195,#11196,#5648,.T.);
#13660=EDGE_CURVE('',#11196,#11197,#945,.T.);
#13661=EDGE_CURVE('',#11197,#11198,#10645,.T.);
#13662=EDGE_CURVE('',#11198,#11199,#946,.T.);
#13663=EDGE_CURVE('',#11199,#11200,#5649,.T.);
#13664=EDGE_CURVE('',#11200,#11201,#10646,.T.);
#13665=EDGE_CURVE('',#11201,#11202,#5650,.T.);
#13666=EDGE_CURVE('',#11202,#11203,#947,.T.);
#13667=EDGE_CURVE('',#11203,#11204,#10647,.T.);
#13668=EDGE_CURVE('',#11204,#11205,#948,.T.);
#13669=EDGE_CURVE('',#11205,#11206,#5651,.T.);
#13670=EDGE_CURVE('',#11206,#11207,#10648,.T.);
#13671=EDGE_CURVE('',#11207,#11208,#5652,.T.);
#13672=EDGE_CURVE('',#11208,#11209,#949,.T.);
#13673=EDGE_CURVE('',#11209,#11210,#10649,.T.);
#13674=EDGE_CURVE('',#11210,#11211,#950,.T.);
#13675=EDGE_CURVE('',#11211,#11212,#5653,.T.);
#13676=EDGE_CURVE('',#11212,#11213,#10650,.T.);
#13677=EDGE_CURVE('',#11213,#11214,#5654,.T.);
#13678=EDGE_CURVE('',#11214,#11215,#951,.T.);
#13679=EDGE_CURVE('',#11215,#11216,#10651,.T.);
#13680=EDGE_CURVE('',#11216,#11217,#952,.T.);
#13681=EDGE_CURVE('',#11217,#11218,#5655,.T.);
#13682=EDGE_CURVE('',#11218,#11219,#10652,.T.);
#13683=EDGE_CURVE('',#11219,#11220,#5656,.T.);
#13684=EDGE_CURVE('',#11220,#11221,#953,.T.);
#13685=EDGE_CURVE('',#11221,#11222,#10653,.T.);
#13686=EDGE_CURVE('',#11222,#11223,#954,.T.);
#13687=EDGE_CURVE('',#11223,#11224,#5657,.T.);
#13688=EDGE_CURVE('',#11224,#11225,#10654,.T.);
#13689=EDGE_CURVE('',#11225,#11226,#5658,.T.);
#13690=EDGE_CURVE('',#11226,#11227,#955,.T.);
#13691=EDGE_CURVE('',#11227,#11228,#10655,.T.);
#13692=EDGE_CURVE('',#11228,#11229,#956,.T.);
#13693=EDGE_CURVE('',#11229,#11230,#5659,.T.);
#13694=EDGE_CURVE('',#11230,#11231,#10656,.T.);
#13695=EDGE_CURVE('',#11231,#11232,#5660,.T.);
#13696=EDGE_CURVE('',#11232,#11233,#957,.T.);
#13697=EDGE_CURVE('',#11233,#11234,#10657,.T.);
#13698=EDGE_CURVE('',#11234,#11235,#958,.T.);
#13699=EDGE_CURVE('',#11235,#11236,#5661,.T.);
#13700=EDGE_CURVE('',#11236,#11237,#10658,.T.);
#13701=EDGE_CURVE('',#11237,#11238,#5662,.T.);
#13702=EDGE_CURVE('',#11238,#11239,#959,.T.);
#13703=EDGE_CURVE('',#11239,#11240,#10659,.T.);
#13704=EDGE_CURVE('',#11240,#11241,#960,.T.);
#13705=EDGE_CURVE('',#11241,#11242,#5663,.T.);
#13706=EDGE_CURVE('',#11242,#11243,#10660,.T.);
#13707=EDGE_CURVE('',#11243,#11244,#5664,.T.);
#13708=EDGE_CURVE('',#11244,#11245,#961,.T.);
#13709=EDGE_CURVE('',#11245,#11246,#10661,.T.);
#13710=EDGE_CURVE('',#11246,#11247,#962,.T.);
#13711=EDGE_CURVE('',#11247,#11248,#5665,.T.);
#13712=EDGE_CURVE('',#11248,#11249,#10662,.T.);
#13713=EDGE_CURVE('',#11249,#11142,#5666,.T.);
#13714=EDGE_CURVE('',#11250,#11250,#10663,.T.);
#13715=EDGE_CURVE('',#11250,#11140,#5667,.T.);
#13716=EDGE_CURVE('',#11251,#11251,#10664,.T.);
#13717=EDGE_CURVE('',#11251,#11252,#5668,.T.);
#13718=EDGE_CURVE('',#11252,#11253,#10665,.T.);
#13719=EDGE_CURVE('',#11253,#11252,#10666,.T.);
#13720=EDGE_CURVE('',#11254,#11255,#963,.T.);
#13721=EDGE_CURVE('',#11255,#11256,#5669,.T.);
#13722=EDGE_CURVE('',#11256,#11257,#10667,.T.);
#13723=EDGE_CURVE('',#11257,#11258,#5670,.T.);
#13724=EDGE_CURVE('',#11258,#11259,#964,.T.);
#13725=EDGE_CURVE('',#11259,#11260,#10668,.T.);
#13726=EDGE_CURVE('',#11260,#11261,#965,.T.);
#13727=EDGE_CURVE('',#11261,#11262,#5671,.T.);
#13728=EDGE_CURVE('',#11262,#11263,#10669,.T.);
#13729=EDGE_CURVE('',#11263,#11264,#5672,.T.);
#13730=EDGE_CURVE('',#11264,#11265,#966,.T.);
#13731=EDGE_CURVE('',#11265,#11266,#10670,.T.);
#13732=EDGE_CURVE('',#11266,#11267,#967,.T.);
#13733=EDGE_CURVE('',#11267,#11268,#5673,.T.);
#13734=EDGE_CURVE('',#11268,#11269,#10671,.T.);
#13735=EDGE_CURVE('',#11269,#11270,#5674,.T.);
#13736=EDGE_CURVE('',#11270,#11271,#968,.T.);
#13737=EDGE_CURVE('',#11271,#11272,#10672,.T.);
#13738=EDGE_CURVE('',#11272,#11273,#969,.T.);
#13739=EDGE_CURVE('',#11273,#11274,#5675,.T.);
#13740=EDGE_CURVE('',#11274,#11275,#10673,.T.);
#13741=EDGE_CURVE('',#11275,#11276,#5676,.T.);
#13742=EDGE_CURVE('',#11276,#11277,#970,.T.);
#13743=EDGE_CURVE('',#11277,#11278,#10674,.T.);
#13744=EDGE_CURVE('',#11278,#11279,#971,.T.);
#13745=EDGE_CURVE('',#11279,#11280,#5677,.T.);
#13746=EDGE_CURVE('',#11280,#11281,#10675,.T.);
#13747=EDGE_CURVE('',#11281,#11282,#5678,.T.);
#13748=EDGE_CURVE('',#11282,#11283,#972,.T.);
#13749=EDGE_CURVE('',#11283,#11284,#10676,.T.);
#13750=EDGE_CURVE('',#11284,#11285,#973,.T.);
#13751=EDGE_CURVE('',#11285,#11286,#5679,.T.);
#13752=EDGE_CURVE('',#11286,#11287,#10677,.T.);
#13753=EDGE_CURVE('',#11287,#11288,#5680,.T.);
#13754=EDGE_CURVE('',#11288,#11289,#974,.T.);
#13755=EDGE_CURVE('',#11289,#11290,#10678,.T.);
#13756=EDGE_CURVE('',#11290,#11291,#975,.T.);
#13757=EDGE_CURVE('',#11291,#11292,#5681,.T.);
#13758=EDGE_CURVE('',#11292,#11293,#10679,.T.);
#13759=EDGE_CURVE('',#11293,#11294,#5682,.T.);
#13760=EDGE_CURVE('',#11294,#11295,#976,.T.);
#13761=EDGE_CURVE('',#11295,#11296,#10680,.T.);
#13762=EDGE_CURVE('',#11296,#11297,#977,.T.);
#13763=EDGE_CURVE('',#11297,#11298,#5683,.T.);
#13764=EDGE_CURVE('',#11298,#11299,#10681,.T.);
#13765=EDGE_CURVE('',#11299,#11300,#5684,.T.);
#13766=EDGE_CURVE('',#11300,#11301,#978,.T.);
#13767=EDGE_CURVE('',#11301,#11302,#10682,.T.);
#13768=EDGE_CURVE('',#11302,#11303,#979,.T.);
#13769=EDGE_CURVE('',#11303,#11304,#5685,.T.);
#13770=EDGE_CURVE('',#11304,#11305,#10683,.T.);
#13771=EDGE_CURVE('',#11305,#11306,#5686,.T.);
#13772=EDGE_CURVE('',#11306,#11307,#980,.T.);
#13773=EDGE_CURVE('',#11307,#11308,#10684,.T.);
#13774=EDGE_CURVE('',#11308,#11309,#981,.T.);
#13775=EDGE_CURVE('',#11309,#11310,#5687,.T.);
#13776=EDGE_CURVE('',#11310,#11311,#10685,.T.);
#13777=EDGE_CURVE('',#11311,#11312,#5688,.T.);
#13778=EDGE_CURVE('',#11312,#11313,#982,.T.);
#13779=EDGE_CURVE('',#11313,#11314,#10686,.T.);
#13780=EDGE_CURVE('',#11314,#11315,#983,.T.);
#13781=EDGE_CURVE('',#11315,#11316,#5689,.T.);
#13782=EDGE_CURVE('',#11316,#11317,#10687,.T.);
#13783=EDGE_CURVE('',#11317,#11318,#5690,.T.);
#13784=EDGE_CURVE('',#11318,#11319,#984,.T.);
#13785=EDGE_CURVE('',#11319,#11320,#10688,.T.);
#13786=EDGE_CURVE('',#11320,#11321,#985,.T.);
#13787=EDGE_CURVE('',#11321,#11322,#5691,.T.);
#13788=EDGE_CURVE('',#11322,#11323,#10689,.T.);
#13789=EDGE_CURVE('',#11323,#11324,#5692,.T.);
#13790=EDGE_CURVE('',#11324,#11325,#986,.T.);
#13791=EDGE_CURVE('',#11325,#11326,#10690,.T.);
#13792=EDGE_CURVE('',#11326,#11327,#987,.T.);
#13793=EDGE_CURVE('',#11327,#11328,#5693,.T.);
#13794=EDGE_CURVE('',#11328,#11329,#10691,.T.);
#13795=EDGE_CURVE('',#11329,#11330,#5694,.T.);
#13796=EDGE_CURVE('',#11330,#11331,#988,.T.);
#13797=EDGE_CURVE('',#11331,#11332,#10692,.T.);
#13798=EDGE_CURVE('',#11332,#11333,#989,.T.);
#13799=EDGE_CURVE('',#11333,#11334,#5695,.T.);
#13800=EDGE_CURVE('',#11334,#11335,#10693,.T.);
#13801=EDGE_CURVE('',#11335,#11336,#5696,.T.);
#13802=EDGE_CURVE('',#11336,#11337,#990,.T.);
#13803=EDGE_CURVE('',#11337,#11338,#10694,.T.);
#13804=EDGE_CURVE('',#11338,#11339,#991,.T.);
#13805=EDGE_CURVE('',#11339,#11340,#5697,.T.);
#13806=EDGE_CURVE('',#11340,#11341,#10695,.T.);
#13807=EDGE_CURVE('',#11341,#11342,#5698,.T.);
#13808=EDGE_CURVE('',#11342,#11343,#992,.T.);
#13809=EDGE_CURVE('',#11343,#11344,#10696,.T.);
#13810=EDGE_CURVE('',#11344,#11345,#993,.T.);
#13811=EDGE_CURVE('',#11345,#11346,#5699,.T.);
#13812=EDGE_CURVE('',#11346,#11347,#10697,.T.);
#13813=EDGE_CURVE('',#11347,#11348,#5700,.T.);
#13814=EDGE_CURVE('',#11348,#11349,#994,.T.);
#13815=EDGE_CURVE('',#11349,#11350,#10698,.T.);
#13816=EDGE_CURVE('',#11350,#11351,#995,.T.);
#13817=EDGE_CURVE('',#11351,#11352,#5701,.T.);
#13818=EDGE_CURVE('',#11352,#11353,#10699,.T.);
#13819=EDGE_CURVE('',#11353,#11354,#5702,.T.);
#13820=EDGE_CURVE('',#11354,#11355,#996,.T.);
#13821=EDGE_CURVE('',#11355,#11356,#10700,.T.);
#13822=EDGE_CURVE('',#11356,#11357,#997,.T.);
#13823=EDGE_CURVE('',#11357,#11358,#5703,.T.);
#13824=EDGE_CURVE('',#11358,#11359,#10701,.T.);
#13825=EDGE_CURVE('',#11359,#11360,#5704,.T.);
#13826=EDGE_CURVE('',#11360,#11361,#998,.T.);
#13827=EDGE_CURVE('',#11361,#11254,#10702,.T.);
#13828=EDGE_CURVE('',#11253,#11362,#5705,.T.);
#13829=EDGE_CURVE('',#11362,#11362,#10703,.T.);
#13830=EDGE_CURVE('',#11363,#11363,#10704,.T.);
#13831=EDGE_CURVE('',#11364,#11364,#10705,.T.);
#13832=EDGE_CURVE('',#11364,#11363,#5706,.T.);
#13833=EDGE_CURVE('',#11365,#11365,#10706,.T.);
#13834=EDGE_CURVE('',#11365,#11364,#5707,.T.);
#13835=EDGE_CURVE('',#11366,#11366,#10707,.T.);
#13836=EDGE_CURVE('',#11362,#11366,#5708,.T.);
#13837=EDGE_CURVE('',#11367,#11367,#10708,.T.);
#13838=EDGE_CURVE('',#11367,#11250,#5709,.T.);
#13839=EDGE_CURVE('',#11368,#11368,#10709,.T.);
#13840=EDGE_CURVE('',#11369,#11369,#10710,.T.);
#13841=EDGE_CURVE('',#11369,#11368,#5710,.T.);
#13842=EDGE_CURVE('',#11370,#11370,#10711,.T.);
#13843=EDGE_CURVE('',#11370,#11369,#5711,.T.);
#13844=EDGE_CURVE('',#11241,#11264,#5712,.T.);
#13845=EDGE_CURVE('',#11265,#11240,#999,.T.);
#13846=EDGE_CURVE('',#11262,#11243,#5713,.T.);
#13847=EDGE_CURVE('',#11242,#11263,#5714,.T.);
#13848=EDGE_CURVE('',#11245,#11260,#1000,.T.);
#13849=EDGE_CURVE('',#11244,#11261,#5715,.T.);
#13850=EDGE_CURVE('',#11229,#11276,#5716,.T.);
#13851=EDGE_CURVE('',#11277,#11228,#1001,.T.);
#13852=EDGE_CURVE('',#11274,#11231,#5717,.T.);
#13853=EDGE_CURVE('',#11230,#11275,#5718,.T.);
#13854=EDGE_CURVE('',#11233,#11272,#1002,.T.);
#13855=EDGE_CURVE('',#11232,#11273,#5719,.T.);
#13856=EDGE_CURVE('',#11217,#11288,#5720,.T.);
#13857=EDGE_CURVE('',#11289,#11216,#1003,.T.);
#13858=EDGE_CURVE('',#11286,#11219,#5721,.T.);
#13859=EDGE_CURVE('',#11218,#11287,#5722,.T.);
#13860=EDGE_CURVE('',#11221,#11284,#1004,.T.);
#13861=EDGE_CURVE('',#11220,#11285,#5723,.T.);
#13862=EDGE_CURVE('',#11205,#11300,#5724,.T.);
#13863=EDGE_CURVE('',#11301,#11204,#1005,.T.);
#13864=EDGE_CURVE('',#11298,#11207,#5725,.T.);
#13865=EDGE_CURVE('',#11206,#11299,#5726,.T.);
#13866=EDGE_CURVE('',#11209,#11296,#1006,.T.);
#13867=EDGE_CURVE('',#11208,#11297,#5727,.T.);
#13868=EDGE_CURVE('',#11145,#11360,#5728,.T.);
#13869=EDGE_CURVE('',#11361,#11144,#1007,.T.);
#13870=EDGE_CURVE('',#11358,#11147,#5729,.T.);
#13871=EDGE_CURVE('',#11146,#11359,#5730,.T.);
#13872=EDGE_CURVE('',#11149,#11356,#1008,.T.);
#13873=EDGE_CURVE('',#11148,#11357,#5731,.T.);
#13874=EDGE_CURVE('',#11187,#11318,#5732,.T.);
#13875=EDGE_CURVE('',#11319,#11186,#1009,.T.);
#13876=EDGE_CURVE('',#11316,#11189,#5733,.T.);
#13877=EDGE_CURVE('',#11188,#11317,#5734,.T.);
#13878=EDGE_CURVE('',#11191,#11314,#1010,.T.);
#13879=EDGE_CURVE('',#11190,#11315,#5735,.T.);
#13880=EDGE_CURVE('',#11175,#11330,#5736,.T.);
#13881=EDGE_CURVE('',#11331,#11174,#1011,.T.);
#13882=EDGE_CURVE('',#11328,#11177,#5737,.T.);
#13883=EDGE_CURVE('',#11176,#11329,#5738,.T.);
#13884=EDGE_CURVE('',#11179,#11326,#1012,.T.);
#13885=EDGE_CURVE('',#11178,#11327,#5739,.T.);
#13886=EDGE_CURVE('',#11163,#11342,#5740,.T.);
#13887=EDGE_CURVE('',#11343,#11162,#1013,.T.);
#13888=EDGE_CURVE('',#11340,#11165,#5741,.T.);
#13889=EDGE_CURVE('',#11164,#11341,#5742,.T.);
#13890=EDGE_CURVE('',#11167,#11338,#1014,.T.);
#13891=EDGE_CURVE('',#11166,#11339,#5743,.T.);
#13892=EDGE_CURVE('',#11151,#11354,#5744,.T.);
#13893=EDGE_CURVE('',#11355,#11150,#1015,.T.);
#13894=EDGE_CURVE('',#11352,#11153,#5745,.T.);
#13895=EDGE_CURVE('',#11152,#11353,#5746,.T.);
#13896=EDGE_CURVE('',#11155,#11350,#1016,.T.);
#13897=EDGE_CURVE('',#11154,#11351,#5747,.T.);
#13898=EDGE_CURVE('',#11157,#11348,#5748,.T.);
#13899=EDGE_CURVE('',#11349,#11156,#1017,.T.);
#13900=EDGE_CURVE('',#11346,#11159,#5749,.T.);
#13901=EDGE_CURVE('',#11158,#11347,#5750,.T.);
#13902=EDGE_CURVE('',#11161,#11344,#1018,.T.);
#13903=EDGE_CURVE('',#11160,#11345,#5751,.T.);
#13904=EDGE_CURVE('',#11169,#11336,#5752,.T.);
#13905=EDGE_CURVE('',#11337,#11168,#1019,.T.);
#13906=EDGE_CURVE('',#11334,#11171,#5753,.T.);
#13907=EDGE_CURVE('',#11170,#11335,#5754,.T.);
#13908=EDGE_CURVE('',#11173,#11332,#1020,.T.);
#13909=EDGE_CURVE('',#11172,#11333,#5755,.T.);
#13910=EDGE_CURVE('',#11181,#11324,#5756,.T.);
#13911=EDGE_CURVE('',#11325,#11180,#1021,.T.);
#13912=EDGE_CURVE('',#11322,#11183,#5757,.T.);
#13913=EDGE_CURVE('',#11182,#11323,#5758,.T.);
#13914=EDGE_CURVE('',#11185,#11320,#1022,.T.);
#13915=EDGE_CURVE('',#11184,#11321,#5759,.T.);
#13916=EDGE_CURVE('',#11193,#11312,#5760,.T.);
#13917=EDGE_CURVE('',#11313,#11192,#1023,.T.);
#13918=EDGE_CURVE('',#11310,#11195,#5761,.T.);
#13919=EDGE_CURVE('',#11194,#11311,#5762,.T.);
#13920=EDGE_CURVE('',#11197,#11308,#1024,.T.);
#13921=EDGE_CURVE('',#11196,#11309,#5763,.T.);
#13922=EDGE_CURVE('',#11199,#11306,#5764,.T.);
#13923=EDGE_CURVE('',#11307,#11198,#1025,.T.);
#13924=EDGE_CURVE('',#11304,#11201,#5765,.T.);
#13925=EDGE_CURVE('',#11200,#11305,#5766,.T.);
#13926=EDGE_CURVE('',#11203,#11302,#1026,.T.);
#13927=EDGE_CURVE('',#11202,#11303,#5767,.T.);
#13928=EDGE_CURVE('',#11211,#11294,#5768,.T.);
#13929=EDGE_CURVE('',#11295,#11210,#1027,.T.);
#13930=EDGE_CURVE('',#11292,#11213,#5769,.T.);
#13931=EDGE_CURVE('',#11212,#11293,#5770,.T.);
#13932=EDGE_CURVE('',#11215,#11290,#1028,.T.);
#13933=EDGE_CURVE('',#11214,#11291,#5771,.T.);
#13934=EDGE_CURVE('',#11223,#11282,#5772,.T.);
#13935=EDGE_CURVE('',#11283,#11222,#1029,.T.);
#13936=EDGE_CURVE('',#11280,#11225,#5773,.T.);
#13937=EDGE_CURVE('',#11224,#11281,#5774,.T.);
#13938=EDGE_CURVE('',#11227,#11278,#1030,.T.);
#13939=EDGE_CURVE('',#11226,#11279,#5775,.T.);
#13940=EDGE_CURVE('',#11235,#11270,#5776,.T.);
#13941=EDGE_CURVE('',#11271,#11234,#1031,.T.);
#13942=EDGE_CURVE('',#11268,#11237,#5777,.T.);
#13943=EDGE_CURVE('',#11236,#11269,#5778,.T.);
#13944=EDGE_CURVE('',#11239,#11266,#1032,.T.);
#13945=EDGE_CURVE('',#11238,#11267,#5779,.T.);
#13946=EDGE_CURVE('',#11247,#11258,#5780,.T.);
#13947=EDGE_CURVE('',#11259,#11246,#1033,.T.);
#13948=EDGE_CURVE('',#11256,#11249,#5781,.T.);
#13949=EDGE_CURVE('',#11248,#11257,#5782,.T.);
#13950=EDGE_CURVE('',#11143,#11254,#1034,.T.);
#13951=EDGE_CURVE('',#11142,#11255,#5783,.T.);
#17498=ORIENTED_EDGE('',*,*,#13602,.T.);
#17499=ORIENTED_EDGE('',*,*,#13603,.T.);
#17500=ORIENTED_EDGE('',*,*,#13604,.T.);
#17501=ORIENTED_EDGE('',*,*,#13605,.T.);
#17502=ORIENTED_EDGE('',*,*,#13604,.F.);
#17503=ORIENTED_EDGE('',*,*,#13605,.F.);
#17504=ORIENTED_EDGE('',*,*,#13606,.T.);
#17505=ORIENTED_EDGE('',*,*,#13607,.T.);
#17506=ORIENTED_EDGE('',*,*,#13608,.T.);
#17507=ORIENTED_EDGE('',*,*,#13609,.T.);
#17508=ORIENTED_EDGE('',*,*,#13610,.T.);
#17509=ORIENTED_EDGE('',*,*,#13611,.T.);
#17510=ORIENTED_EDGE('',*,*,#13612,.T.);
#17511=ORIENTED_EDGE('',*,*,#13613,.T.);
#17512=ORIENTED_EDGE('',*,*,#13614,.T.);
#17513=ORIENTED_EDGE('',*,*,#13615,.T.);
#17514=ORIENTED_EDGE('',*,*,#13616,.T.);
#17515=ORIENTED_EDGE('',*,*,#13617,.T.);
#17516=ORIENTED_EDGE('',*,*,#13618,.T.);
#17517=ORIENTED_EDGE('',*,*,#13619,.T.);
#17518=ORIENTED_EDGE('',*,*,#13620,.T.);
#17519=ORIENTED_EDGE('',*,*,#13621,.T.);
#17520=ORIENTED_EDGE('',*,*,#13622,.T.);
#17521=ORIENTED_EDGE('',*,*,#13623,.T.);
#17522=ORIENTED_EDGE('',*,*,#13624,.T.);
#17523=ORIENTED_EDGE('',*,*,#13625,.T.);
#17524=ORIENTED_EDGE('',*,*,#13626,.T.);
#17525=ORIENTED_EDGE('',*,*,#13627,.T.);
#17526=ORIENTED_EDGE('',*,*,#13628,.T.);
#17527=ORIENTED_EDGE('',*,*,#13629,.T.);
#17528=ORIENTED_EDGE('',*,*,#13630,.T.);
#17529=ORIENTED_EDGE('',*,*,#13631,.T.);
#17530=ORIENTED_EDGE('',*,*,#13632,.T.);
#17531=ORIENTED_EDGE('',*,*,#13633,.T.);
#17532=ORIENTED_EDGE('',*,*,#13634,.T.);
#17533=ORIENTED_EDGE('',*,*,#13635,.T.);
#17534=ORIENTED_EDGE('',*,*,#13636,.T.);
#17535=ORIENTED_EDGE('',*,*,#13637,.T.);
#17536=ORIENTED_EDGE('',*,*,#13638,.T.);
#17537=ORIENTED_EDGE('',*,*,#13639,.T.);
#17538=ORIENTED_EDGE('',*,*,#13640,.T.);
#17539=ORIENTED_EDGE('',*,*,#13641,.T.);
#17540=ORIENTED_EDGE('',*,*,#13642,.T.);
#17541=ORIENTED_EDGE('',*,*,#13643,.T.);
#17542=ORIENTED_EDGE('',*,*,#13644,.T.);
#17543=ORIENTED_EDGE('',*,*,#13645,.T.);
#17544=ORIENTED_EDGE('',*,*,#13646,.T.);
#17545=ORIENTED_EDGE('',*,*,#13647,.T.);
#17546=ORIENTED_EDGE('',*,*,#13648,.T.);
#17547=ORIENTED_EDGE('',*,*,#13649,.T.);
#17548=ORIENTED_EDGE('',*,*,#13650,.T.);
#17549=ORIENTED_EDGE('',*,*,#13651,.T.);
#17550=ORIENTED_EDGE('',*,*,#13652,.T.);
#17551=ORIENTED_EDGE('',*,*,#13653,.T.);
#17552=ORIENTED_EDGE('',*,*,#13654,.T.);
#17553=ORIENTED_EDGE('',*,*,#13655,.T.);
#17554=ORIENTED_EDGE('',*,*,#13656,.T.);
#17555=ORIENTED_EDGE('',*,*,#13657,.T.);
#17556=ORIENTED_EDGE('',*,*,#13658,.T.);
#17557=ORIENTED_EDGE('',*,*,#13659,.T.);
#17558=ORIENTED_EDGE('',*,*,#13660,.T.);
#17559=ORIENTED_EDGE('',*,*,#13661,.T.);
#17560=ORIENTED_EDGE('',*,*,#13662,.T.);
#17561=ORIENTED_EDGE('',*,*,#13663,.T.);
#17562=ORIENTED_EDGE('',*,*,#13664,.T.);
#17563=ORIENTED_EDGE('',*,*,#13665,.T.);
#17564=ORIENTED_EDGE('',*,*,#13666,.T.);
#17565=ORIENTED_EDGE('',*,*,#13667,.T.);
#17566=ORIENTED_EDGE('',*,*,#13668,.T.);
#17567=ORIENTED_EDGE('',*,*,#13669,.T.);
#17568=ORIENTED_EDGE('',*,*,#13670,.T.);
#17569=ORIENTED_EDGE('',*,*,#13671,.T.);
#17570=ORIENTED_EDGE('',*,*,#13672,.T.);
#17571=ORIENTED_EDGE('',*,*,#13673,.T.);
#17572=ORIENTED_EDGE('',*,*,#13674,.T.);
#17573=ORIENTED_EDGE('',*,*,#13675,.T.);
#17574=ORIENTED_EDGE('',*,*,#13676,.T.);
#17575=ORIENTED_EDGE('',*,*,#13677,.T.);
#17576=ORIENTED_EDGE('',*,*,#13678,.T.);
#17577=ORIENTED_EDGE('',*,*,#13679,.T.);
#17578=ORIENTED_EDGE('',*,*,#13680,.T.);
#17579=ORIENTED_EDGE('',*,*,#13681,.T.);
#17580=ORIENTED_EDGE('',*,*,#13682,.T.);
#17581=ORIENTED_EDGE('',*,*,#13683,.T.);
#17582=ORIENTED_EDGE('',*,*,#13684,.T.);
#17583=ORIENTED_EDGE('',*,*,#13685,.T.);
#17584=ORIENTED_EDGE('',*,*,#13686,.T.);
#17585=ORIENTED_EDGE('',*,*,#13687,.T.);
#17586=ORIENTED_EDGE('',*,*,#13688,.T.);
#17587=ORIENTED_EDGE('',*,*,#13689,.T.);
#17588=ORIENTED_EDGE('',*,*,#13690,.T.);
#17589=ORIENTED_EDGE('',*,*,#13691,.T.);
#17590=ORIENTED_EDGE('',*,*,#13692,.T.);
#17591=ORIENTED_EDGE('',*,*,#13693,.T.);
#17592=ORIENTED_EDGE('',*,*,#13694,.T.);
#17593=ORIENTED_EDGE('',*,*,#13695,.T.);
#17594=ORIENTED_EDGE('',*,*,#13696,.T.);
#17595=ORIENTED_EDGE('',*,*,#13697,.T.);
#17596=ORIENTED_EDGE('',*,*,#13698,.T.);
#17597=ORIENTED_EDGE('',*,*,#13699,.T.);
#17598=ORIENTED_EDGE('',*,*,#13700,.T.);
#17599=ORIENTED_EDGE('',*,*,#13701,.T.);
#17600=ORIENTED_EDGE('',*,*,#13702,.T.);
#17601=ORIENTED_EDGE('',*,*,#13703,.T.);
#17602=ORIENTED_EDGE('',*,*,#13704,.T.);
#17603=ORIENTED_EDGE('',*,*,#13705,.T.);
#17604=ORIENTED_EDGE('',*,*,#13706,.T.);
#17605=ORIENTED_EDGE('',*,*,#13707,.T.);
#17606=ORIENTED_EDGE('',*,*,#13708,.T.);
#17607=ORIENTED_EDGE('',*,*,#13709,.T.);
#17608=ORIENTED_EDGE('',*,*,#13710,.T.);
#17609=ORIENTED_EDGE('',*,*,#13711,.T.);
#17610=ORIENTED_EDGE('',*,*,#13712,.T.);
#17611=ORIENTED_EDGE('',*,*,#13713,.T.);
#17612=ORIENTED_EDGE('',*,*,#13714,.F.);
#17613=ORIENTED_EDGE('',*,*,#13715,.T.);
#17614=ORIENTED_EDGE('',*,*,#13602,.F.);
#17615=ORIENTED_EDGE('',*,*,#13603,.F.);
#17616=ORIENTED_EDGE('',*,*,#13715,.F.);
#17617=ORIENTED_EDGE('',*,*,#13716,.T.);
#17618=ORIENTED_EDGE('',*,*,#13717,.T.);
#17619=ORIENTED_EDGE('',*,*,#13718,.T.);
#17620=ORIENTED_EDGE('',*,*,#13719,.T.);
#17621=ORIENTED_EDGE('',*,*,#13717,.F.);
#17622=ORIENTED_EDGE('',*,*,#13716,.F.);
#17623=ORIENTED_EDGE('',*,*,#13720,.T.);
#17624=ORIENTED_EDGE('',*,*,#13721,.T.);
#17625=ORIENTED_EDGE('',*,*,#13722,.T.);
#17626=ORIENTED_EDGE('',*,*,#13723,.T.);
#17627=ORIENTED_EDGE('',*,*,#13724,.T.);
#17628=ORIENTED_EDGE('',*,*,#13725,.T.);
#17629=ORIENTED_EDGE('',*,*,#13726,.T.);
#17630=ORIENTED_EDGE('',*,*,#13727,.T.);
#17631=ORIENTED_EDGE('',*,*,#13728,.T.);
#17632=ORIENTED_EDGE('',*,*,#13729,.T.);
#17633=ORIENTED_EDGE('',*,*,#13730,.T.);
#17634=ORIENTED_EDGE('',*,*,#13731,.T.);
#17635=ORIENTED_EDGE('',*,*,#13732,.T.);
#17636=ORIENTED_EDGE('',*,*,#13733,.T.);
#17637=ORIENTED_EDGE('',*,*,#13734,.T.);
#17638=ORIENTED_EDGE('',*,*,#13735,.T.);
#17639=ORIENTED_EDGE('',*,*,#13736,.T.);
#17640=ORIENTED_EDGE('',*,*,#13737,.T.);
#17641=ORIENTED_EDGE('',*,*,#13738,.T.);
#17642=ORIENTED_EDGE('',*,*,#13739,.T.);
#17643=ORIENTED_EDGE('',*,*,#13740,.T.);
#17644=ORIENTED_EDGE('',*,*,#13741,.T.);
#17645=ORIENTED_EDGE('',*,*,#13742,.T.);
#17646=ORIENTED_EDGE('',*,*,#13743,.T.);
#17647=ORIENTED_EDGE('',*,*,#13744,.T.);
#17648=ORIENTED_EDGE('',*,*,#13745,.T.);
#17649=ORIENTED_EDGE('',*,*,#13746,.T.);
#17650=ORIENTED_EDGE('',*,*,#13747,.T.);
#17651=ORIENTED_EDGE('',*,*,#13748,.T.);
#17652=ORIENTED_EDGE('',*,*,#13749,.T.);
#17653=ORIENTED_EDGE('',*,*,#13750,.T.);
#17654=ORIENTED_EDGE('',*,*,#13751,.T.);
#17655=ORIENTED_EDGE('',*,*,#13752,.T.);
#17656=ORIENTED_EDGE('',*,*,#13753,.T.);
#17657=ORIENTED_EDGE('',*,*,#13754,.T.);
#17658=ORIENTED_EDGE('',*,*,#13755,.T.);
#17659=ORIENTED_EDGE('',*,*,#13756,.T.);
#17660=ORIENTED_EDGE('',*,*,#13757,.T.);
#17661=ORIENTED_EDGE('',*,*,#13758,.T.);
#17662=ORIENTED_EDGE('',*,*,#13759,.T.);
#17663=ORIENTED_EDGE('',*,*,#13760,.T.);
#17664=ORIENTED_EDGE('',*,*,#13761,.T.);
#17665=ORIENTED_EDGE('',*,*,#13762,.T.);
#17666=ORIENTED_EDGE('',*,*,#13763,.T.);
#17667=ORIENTED_EDGE('',*,*,#13764,.T.);
#17668=ORIENTED_EDGE('',*,*,#13765,.T.);
#17669=ORIENTED_EDGE('',*,*,#13766,.T.);
#17670=ORIENTED_EDGE('',*,*,#13767,.T.);
#17671=ORIENTED_EDGE('',*,*,#13768,.T.);
#17672=ORIENTED_EDGE('',*,*,#13769,.T.);
#17673=ORIENTED_EDGE('',*,*,#13770,.T.);
#17674=ORIENTED_EDGE('',*,*,#13771,.T.);
#17675=ORIENTED_EDGE('',*,*,#13772,.T.);
#17676=ORIENTED_EDGE('',*,*,#13773,.T.);
#17677=ORIENTED_EDGE('',*,*,#13774,.T.);
#17678=ORIENTED_EDGE('',*,*,#13775,.T.);
#17679=ORIENTED_EDGE('',*,*,#13776,.T.);
#17680=ORIENTED_EDGE('',*,*,#13777,.T.);
#17681=ORIENTED_EDGE('',*,*,#13778,.T.);
#17682=ORIENTED_EDGE('',*,*,#13779,.T.);
#17683=ORIENTED_EDGE('',*,*,#13780,.T.);
#17684=ORIENTED_EDGE('',*,*,#13781,.T.);
#17685=ORIENTED_EDGE('',*,*,#13782,.T.);
#17686=ORIENTED_EDGE('',*,*,#13783,.T.);
#17687=ORIENTED_EDGE('',*,*,#13784,.T.);
#17688=ORIENTED_EDGE('',*,*,#13785,.T.);
#17689=ORIENTED_EDGE('',*,*,#13786,.T.);
#17690=ORIENTED_EDGE('',*,*,#13787,.T.);
#17691=ORIENTED_EDGE('',*,*,#13788,.T.);
#17692=ORIENTED_EDGE('',*,*,#13789,.T.);
#17693=ORIENTED_EDGE('',*,*,#13790,.T.);
#17694=ORIENTED_EDGE('',*,*,#13791,.T.);
#17695=ORIENTED_EDGE('',*,*,#13792,.T.);
#17696=ORIENTED_EDGE('',*,*,#13793,.T.);
#17697=ORIENTED_EDGE('',*,*,#13794,.T.);
#17698=ORIENTED_EDGE('',*,*,#13795,.T.);
#17699=ORIENTED_EDGE('',*,*,#13796,.T.);
#17700=ORIENTED_EDGE('',*,*,#13797,.T.);
#17701=ORIENTED_EDGE('',*,*,#13798,.T.);
#17702=ORIENTED_EDGE('',*,*,#13799,.T.);
#17703=ORIENTED_EDGE('',*,*,#13800,.T.);
#17704=ORIENTED_EDGE('',*,*,#13801,.T.);
#17705=ORIENTED_EDGE('',*,*,#13802,.T.);
#17706=ORIENTED_EDGE('',*,*,#13803,.T.);
#17707=ORIENTED_EDGE('',*,*,#13804,.T.);
#17708=ORIENTED_EDGE('',*,*,#13805,.T.);
#17709=ORIENTED_EDGE('',*,*,#13806,.T.);
#17710=ORIENTED_EDGE('',*,*,#13807,.T.);
#17711=ORIENTED_EDGE('',*,*,#13808,.T.);
#17712=ORIENTED_EDGE('',*,*,#13809,.T.);
#17713=ORIENTED_EDGE('',*,*,#13810,.T.);
#17714=ORIENTED_EDGE('',*,*,#13811,.T.);
#17715=ORIENTED_EDGE('',*,*,#13812,.T.);
#17716=ORIENTED_EDGE('',*,*,#13813,.T.);
#17717=ORIENTED_EDGE('',*,*,#13814,.T.);
#17718=ORIENTED_EDGE('',*,*,#13815,.T.);
#17719=ORIENTED_EDGE('',*,*,#13816,.T.);
#17720=ORIENTED_EDGE('',*,*,#13817,.T.);
#17721=ORIENTED_EDGE('',*,*,#13818,.T.);
#17722=ORIENTED_EDGE('',*,*,#13819,.T.);
#17723=ORIENTED_EDGE('',*,*,#13820,.T.);
#17724=ORIENTED_EDGE('',*,*,#13821,.T.);
#17725=ORIENTED_EDGE('',*,*,#13822,.T.);
#17726=ORIENTED_EDGE('',*,*,#13823,.T.);
#17727=ORIENTED_EDGE('',*,*,#13824,.T.);
#17728=ORIENTED_EDGE('',*,*,#13825,.T.);
#17729=ORIENTED_EDGE('',*,*,#13826,.T.);
#17730=ORIENTED_EDGE('',*,*,#13827,.T.);
#17731=ORIENTED_EDGE('',*,*,#13718,.F.);
#17732=ORIENTED_EDGE('',*,*,#13719,.F.);
#17733=ORIENTED_EDGE('',*,*,#13828,.T.);
#17734=ORIENTED_EDGE('',*,*,#13829,.T.);
#17735=ORIENTED_EDGE('',*,*,#13828,.F.);
#17736=ORIENTED_EDGE('',*,*,#13830,.F.);
#17737=ORIENTED_EDGE('',*,*,#13831,.F.);
#17738=ORIENTED_EDGE('',*,*,#13832,.T.);
#17739=ORIENTED_EDGE('',*,*,#13830,.T.);
#17740=ORIENTED_EDGE('',*,*,#13832,.F.);
#17741=ORIENTED_EDGE('',*,*,#13833,.F.);
#17742=ORIENTED_EDGE('',*,*,#13834,.T.);
#17743=ORIENTED_EDGE('',*,*,#13831,.T.);
#17744=ORIENTED_EDGE('',*,*,#13834,.F.);
#17745=ORIENTED_EDGE('',*,*,#13835,.F.);
#17746=ORIENTED_EDGE('',*,*,#13833,.T.);
#17747=ORIENTED_EDGE('',*,*,#13829,.F.);
#17748=ORIENTED_EDGE('',*,*,#13836,.T.);
#17749=ORIENTED_EDGE('',*,*,#13835,.T.);
#17750=ORIENTED_EDGE('',*,*,#13836,.F.);
#17751=ORIENTED_EDGE('',*,*,#13837,.F.);
#17752=ORIENTED_EDGE('',*,*,#13838,.T.);
#17753=ORIENTED_EDGE('',*,*,#13714,.T.);
#17754=ORIENTED_EDGE('',*,*,#13838,.F.);
#17755=ORIENTED_EDGE('',*,*,#13837,.T.);
#17756=ORIENTED_EDGE('',*,*,#13839,.F.);
#17757=ORIENTED_EDGE('',*,*,#13840,.F.);
#17758=ORIENTED_EDGE('',*,*,#13841,.T.);
#17759=ORIENTED_EDGE('',*,*,#13839,.T.);
#17760=ORIENTED_EDGE('',*,*,#13841,.F.);
#17761=ORIENTED_EDGE('',*,*,#13842,.F.);
#17762=ORIENTED_EDGE('',*,*,#13843,.T.);
#17763=ORIENTED_EDGE('',*,*,#13840,.T.);
#17764=ORIENTED_EDGE('',*,*,#13843,.F.);
#17765=ORIENTED_EDGE('',*,*,#13842,.T.);
#17766=ORIENTED_EDGE('',*,*,#13730,.F.);
#17767=ORIENTED_EDGE('',*,*,#13844,.F.);
#17768=ORIENTED_EDGE('',*,*,#13704,.F.);
#17769=ORIENTED_EDGE('',*,*,#13845,.F.);
#17770=ORIENTED_EDGE('',*,*,#13728,.F.);
#17771=ORIENTED_EDGE('',*,*,#13846,.T.);
#17772=ORIENTED_EDGE('',*,*,#13706,.F.);
#17773=ORIENTED_EDGE('',*,*,#13847,.T.);
#17774=ORIENTED_EDGE('',*,*,#13729,.F.);
#17775=ORIENTED_EDGE('',*,*,#13847,.F.);
#17776=ORIENTED_EDGE('',*,*,#13705,.F.);
#17777=ORIENTED_EDGE('',*,*,#13844,.T.);
#17778=ORIENTED_EDGE('',*,*,#13726,.F.);
#17779=ORIENTED_EDGE('',*,*,#13848,.F.);
#17780=ORIENTED_EDGE('',*,*,#13708,.F.);
#17781=ORIENTED_EDGE('',*,*,#13849,.T.);
#17782=ORIENTED_EDGE('',*,*,#13727,.F.);
#17783=ORIENTED_EDGE('',*,*,#13849,.F.);
#17784=ORIENTED_EDGE('',*,*,#13707,.F.);
#17785=ORIENTED_EDGE('',*,*,#13846,.F.);
#17786=ORIENTED_EDGE('',*,*,#13742,.F.);
#17787=ORIENTED_EDGE('',*,*,#13850,.F.);
#17788=ORIENTED_EDGE('',*,*,#13692,.F.);
#17789=ORIENTED_EDGE('',*,*,#13851,.F.);
#17790=ORIENTED_EDGE('',*,*,#13740,.F.);
#17791=ORIENTED_EDGE('',*,*,#13852,.T.);
#17792=ORIENTED_EDGE('',*,*,#13694,.F.);
#17793=ORIENTED_EDGE('',*,*,#13853,.T.);
#17794=ORIENTED_EDGE('',*,*,#13741,.F.);
#17795=ORIENTED_EDGE('',*,*,#13853,.F.);
#17796=ORIENTED_EDGE('',*,*,#13693,.F.);
#17797=ORIENTED_EDGE('',*,*,#13850,.T.);
#17798=ORIENTED_EDGE('',*,*,#13738,.F.);
#17799=ORIENTED_EDGE('',*,*,#13854,.F.);
#17800=ORIENTED_EDGE('',*,*,#13696,.F.);
#17801=ORIENTED_EDGE('',*,*,#13855,.T.);
#17802=ORIENTED_EDGE('',*,*,#13739,.F.);
#17803=ORIENTED_EDGE('',*,*,#13855,.F.);
#17804=ORIENTED_EDGE('',*,*,#13695,.F.);
#17805=ORIENTED_EDGE('',*,*,#13852,.F.);
#17806=ORIENTED_EDGE('',*,*,#13754,.F.);
#17807=ORIENTED_EDGE('',*,*,#13856,.F.);
#17808=ORIENTED_EDGE('',*,*,#13680,.F.);
#17809=ORIENTED_EDGE('',*,*,#13857,.F.);
#17810=ORIENTED_EDGE('',*,*,#13752,.F.);
#17811=ORIENTED_EDGE('',*,*,#13858,.T.);
#17812=ORIENTED_EDGE('',*,*,#13682,.F.);
#17813=ORIENTED_EDGE('',*,*,#13859,.T.);
#17814=ORIENTED_EDGE('',*,*,#13753,.F.);
#17815=ORIENTED_EDGE('',*,*,#13859,.F.);
#17816=ORIENTED_EDGE('',*,*,#13681,.F.);
#17817=ORIENTED_EDGE('',*,*,#13856,.T.);
#17818=ORIENTED_EDGE('',*,*,#13750,.F.);
#17819=ORIENTED_EDGE('',*,*,#13860,.F.);
#17820=ORIENTED_EDGE('',*,*,#13684,.F.);
#17821=ORIENTED_EDGE('',*,*,#13861,.T.);
#17822=ORIENTED_EDGE('',*,*,#13751,.F.);
#17823=ORIENTED_EDGE('',*,*,#13861,.F.);
#17824=ORIENTED_EDGE('',*,*,#13683,.F.);
#17825=ORIENTED_EDGE('',*,*,#13858,.F.);
#17826=ORIENTED_EDGE('',*,*,#13766,.F.);
#17827=ORIENTED_EDGE('',*,*,#13862,.F.);
#17828=ORIENTED_EDGE('',*,*,#13668,.F.);
#17829=ORIENTED_EDGE('',*,*,#13863,.F.);
#17830=ORIENTED_EDGE('',*,*,#13764,.F.);
#17831=ORIENTED_EDGE('',*,*,#13864,.T.);
#17832=ORIENTED_EDGE('',*,*,#13670,.F.);
#17833=ORIENTED_EDGE('',*,*,#13865,.T.);
#17834=ORIENTED_EDGE('',*,*,#13765,.F.);
#17835=ORIENTED_EDGE('',*,*,#13865,.F.);
#17836=ORIENTED_EDGE('',*,*,#13669,.F.);
#17837=ORIENTED_EDGE('',*,*,#13862,.T.);
#17838=ORIENTED_EDGE('',*,*,#13762,.F.);
#17839=ORIENTED_EDGE('',*,*,#13866,.F.);
#17840=ORIENTED_EDGE('',*,*,#13672,.F.);
#17841=ORIENTED_EDGE('',*,*,#13867,.T.);
#17842=ORIENTED_EDGE('',*,*,#13763,.F.);
#17843=ORIENTED_EDGE('',*,*,#13867,.F.);
#17844=ORIENTED_EDGE('',*,*,#13671,.F.);
#17845=ORIENTED_EDGE('',*,*,#13864,.F.);
#17846=ORIENTED_EDGE('',*,*,#13826,.F.);
#17847=ORIENTED_EDGE('',*,*,#13868,.F.);
#17848=ORIENTED_EDGE('',*,*,#13608,.F.);
#17849=ORIENTED_EDGE('',*,*,#13869,.F.);
#17850=ORIENTED_EDGE('',*,*,#13824,.F.);
#17851=ORIENTED_EDGE('',*,*,#13870,.T.);
#17852=ORIENTED_EDGE('',*,*,#13610,.F.);
#17853=ORIENTED_EDGE('',*,*,#13871,.T.);
#17854=ORIENTED_EDGE('',*,*,#13825,.F.);
#17855=ORIENTED_EDGE('',*,*,#13871,.F.);
#17856=ORIENTED_EDGE('',*,*,#13609,.F.);
#17857=ORIENTED_EDGE('',*,*,#13868,.T.);
#17858=ORIENTED_EDGE('',*,*,#13822,.F.);
#17859=ORIENTED_EDGE('',*,*,#13872,.F.);
#17860=ORIENTED_EDGE('',*,*,#13612,.F.);
#17861=ORIENTED_EDGE('',*,*,#13873,.T.);
#17862=ORIENTED_EDGE('',*,*,#13823,.F.);
#17863=ORIENTED_EDGE('',*,*,#13873,.F.);
#17864=ORIENTED_EDGE('',*,*,#13611,.F.);
#17865=ORIENTED_EDGE('',*,*,#13870,.F.);
#17866=ORIENTED_EDGE('',*,*,#13784,.F.);
#17867=ORIENTED_EDGE('',*,*,#13874,.F.);
#17868=ORIENTED_EDGE('',*,*,#13650,.F.);
#17869=ORIENTED_EDGE('',*,*,#13875,.F.);
#17870=ORIENTED_EDGE('',*,*,#13782,.F.);
#17871=ORIENTED_EDGE('',*,*,#13876,.T.);
#17872=ORIENTED_EDGE('',*,*,#13652,.F.);
#17873=ORIENTED_EDGE('',*,*,#13877,.T.);
#17874=ORIENTED_EDGE('',*,*,#13783,.F.);
#17875=ORIENTED_EDGE('',*,*,#13877,.F.);
#17876=ORIENTED_EDGE('',*,*,#13651,.F.);
#17877=ORIENTED_EDGE('',*,*,#13874,.T.);
#17878=ORIENTED_EDGE('',*,*,#13780,.F.);
#17879=ORIENTED_EDGE('',*,*,#13878,.F.);
#17880=ORIENTED_EDGE('',*,*,#13654,.F.);
#17881=ORIENTED_EDGE('',*,*,#13879,.T.);
#17882=ORIENTED_EDGE('',*,*,#13781,.F.);
#17883=ORIENTED_EDGE('',*,*,#13879,.F.);
#17884=ORIENTED_EDGE('',*,*,#13653,.F.);
#17885=ORIENTED_EDGE('',*,*,#13876,.F.);
#17886=ORIENTED_EDGE('',*,*,#13796,.F.);
#17887=ORIENTED_EDGE('',*,*,#13880,.F.);
#17888=ORIENTED_EDGE('',*,*,#13638,.F.);
#17889=ORIENTED_EDGE('',*,*,#13881,.F.);
#17890=ORIENTED_EDGE('',*,*,#13794,.F.);
#17891=ORIENTED_EDGE('',*,*,#13882,.T.);
#17892=ORIENTED_EDGE('',*,*,#13640,.F.);
#17893=ORIENTED_EDGE('',*,*,#13883,.T.);
#17894=ORIENTED_EDGE('',*,*,#13795,.F.);
#17895=ORIENTED_EDGE('',*,*,#13883,.F.);
#17896=ORIENTED_EDGE('',*,*,#13639,.F.);
#17897=ORIENTED_EDGE('',*,*,#13880,.T.);
#17898=ORIENTED_EDGE('',*,*,#13792,.F.);
#17899=ORIENTED_EDGE('',*,*,#13884,.F.);
#17900=ORIENTED_EDGE('',*,*,#13642,.F.);
#17901=ORIENTED_EDGE('',*,*,#13885,.T.);
#17902=ORIENTED_EDGE('',*,*,#13793,.F.);
#17903=ORIENTED_EDGE('',*,*,#13885,.F.);
#17904=ORIENTED_EDGE('',*,*,#13641,.F.);
#17905=ORIENTED_EDGE('',*,*,#13882,.F.);
#17906=ORIENTED_EDGE('',*,*,#13808,.F.);
#17907=ORIENTED_EDGE('',*,*,#13886,.F.);
#17908=ORIENTED_EDGE('',*,*,#13626,.F.);
#17909=ORIENTED_EDGE('',*,*,#13887,.F.);
#17910=ORIENTED_EDGE('',*,*,#13806,.F.);
#17911=ORIENTED_EDGE('',*,*,#13888,.T.);
#17912=ORIENTED_EDGE('',*,*,#13628,.F.);
#17913=ORIENTED_EDGE('',*,*,#13889,.T.);
#17914=ORIENTED_EDGE('',*,*,#13807,.F.);
#17915=ORIENTED_EDGE('',*,*,#13889,.F.);
#17916=ORIENTED_EDGE('',*,*,#13627,.F.);
#17917=ORIENTED_EDGE('',*,*,#13886,.T.);
#17918=ORIENTED_EDGE('',*,*,#13804,.F.);
#17919=ORIENTED_EDGE('',*,*,#13890,.F.);
#17920=ORIENTED_EDGE('',*,*,#13630,.F.);
#17921=ORIENTED_EDGE('',*,*,#13891,.T.);
#17922=ORIENTED_EDGE('',*,*,#13805,.F.);
#17923=ORIENTED_EDGE('',*,*,#13891,.F.);
#17924=ORIENTED_EDGE('',*,*,#13629,.F.);
#17925=ORIENTED_EDGE('',*,*,#13888,.F.);
#17926=ORIENTED_EDGE('',*,*,#13820,.F.);
#17927=ORIENTED_EDGE('',*,*,#13892,.F.);
#17928=ORIENTED_EDGE('',*,*,#13614,.F.);
#17929=ORIENTED_EDGE('',*,*,#13893,.F.);
#17930=ORIENTED_EDGE('',*,*,#13818,.F.);
#17931=ORIENTED_EDGE('',*,*,#13894,.T.);
#17932=ORIENTED_EDGE('',*,*,#13616,.F.);
#17933=ORIENTED_EDGE('',*,*,#13895,.T.);
#17934=ORIENTED_EDGE('',*,*,#13819,.F.);
#17935=ORIENTED_EDGE('',*,*,#13895,.F.);
#17936=ORIENTED_EDGE('',*,*,#13615,.F.);
#17937=ORIENTED_EDGE('',*,*,#13892,.T.);
#17938=ORIENTED_EDGE('',*,*,#13816,.F.);
#17939=ORIENTED_EDGE('',*,*,#13896,.F.);
#17940=ORIENTED_EDGE('',*,*,#13618,.F.);
#17941=ORIENTED_EDGE('',*,*,#13897,.T.);
#17942=ORIENTED_EDGE('',*,*,#13817,.F.);
#17943=ORIENTED_EDGE('',*,*,#13897,.F.);
#17944=ORIENTED_EDGE('',*,*,#13617,.F.);
#17945=ORIENTED_EDGE('',*,*,#13894,.F.);
#17946=ORIENTED_EDGE('',*,*,#13814,.F.);
#17947=ORIENTED_EDGE('',*,*,#13898,.F.);
#17948=ORIENTED_EDGE('',*,*,#13620,.F.);
#17949=ORIENTED_EDGE('',*,*,#13899,.F.);
#17950=ORIENTED_EDGE('',*,*,#13812,.F.);
#17951=ORIENTED_EDGE('',*,*,#13900,.T.);
#17952=ORIENTED_EDGE('',*,*,#13622,.F.);
#17953=ORIENTED_EDGE('',*,*,#13901,.T.);
#17954=ORIENTED_EDGE('',*,*,#13813,.F.);
#17955=ORIENTED_EDGE('',*,*,#13901,.F.);
#17956=ORIENTED_EDGE('',*,*,#13621,.F.);
#17957=ORIENTED_EDGE('',*,*,#13898,.T.);
#17958=ORIENTED_EDGE('',*,*,#13810,.F.);
#17959=ORIENTED_EDGE('',*,*,#13902,.F.);
#17960=ORIENTED_EDGE('',*,*,#13624,.F.);
#17961=ORIENTED_EDGE('',*,*,#13903,.T.);
#17962=ORIENTED_EDGE('',*,*,#13811,.F.);
#17963=ORIENTED_EDGE('',*,*,#13903,.F.);
#17964=ORIENTED_EDGE('',*,*,#13623,.F.);
#17965=ORIENTED_EDGE('',*,*,#13900,.F.);
#17966=ORIENTED_EDGE('',*,*,#13802,.F.);
#17967=ORIENTED_EDGE('',*,*,#13904,.F.);
#17968=ORIENTED_EDGE('',*,*,#13632,.F.);
#17969=ORIENTED_EDGE('',*,*,#13905,.F.);
#17970=ORIENTED_EDGE('',*,*,#13800,.F.);
#17971=ORIENTED_EDGE('',*,*,#13906,.T.);
#17972=ORIENTED_EDGE('',*,*,#13634,.F.);
#17973=ORIENTED_EDGE('',*,*,#13907,.T.);
#17974=ORIENTED_EDGE('',*,*,#13801,.F.);
#17975=ORIENTED_EDGE('',*,*,#13907,.F.);
#17976=ORIENTED_EDGE('',*,*,#13633,.F.);
#17977=ORIENTED_EDGE('',*,*,#13904,.T.);
#17978=ORIENTED_EDGE('',*,*,#13798,.F.);
#17979=ORIENTED_EDGE('',*,*,#13908,.F.);
#17980=ORIENTED_EDGE('',*,*,#13636,.F.);
#17981=ORIENTED_EDGE('',*,*,#13909,.T.);
#17982=ORIENTED_EDGE('',*,*,#13799,.F.);
#17983=ORIENTED_EDGE('',*,*,#13909,.F.);
#17984=ORIENTED_EDGE('',*,*,#13635,.F.);
#17985=ORIENTED_EDGE('',*,*,#13906,.F.);
#17986=ORIENTED_EDGE('',*,*,#13790,.F.);
#17987=ORIENTED_EDGE('',*,*,#13910,.F.);
#17988=ORIENTED_EDGE('',*,*,#13644,.F.);
#17989=ORIENTED_EDGE('',*,*,#13911,.F.);
#17990=ORIENTED_EDGE('',*,*,#13788,.F.);
#17991=ORIENTED_EDGE('',*,*,#13912,.T.);
#17992=ORIENTED_EDGE('',*,*,#13646,.F.);
#17993=ORIENTED_EDGE('',*,*,#13913,.T.);
#17994=ORIENTED_EDGE('',*,*,#13789,.F.);
#17995=ORIENTED_EDGE('',*,*,#13913,.F.);
#17996=ORIENTED_EDGE('',*,*,#13645,.F.);
#17997=ORIENTED_EDGE('',*,*,#13910,.T.);
#17998=ORIENTED_EDGE('',*,*,#13786,.F.);
#17999=ORIENTED_EDGE('',*,*,#13914,.F.);
#18000=ORIENTED_EDGE('',*,*,#13648,.F.);
#18001=ORIENTED_EDGE('',*,*,#13915,.T.);
#18002=ORIENTED_EDGE('',*,*,#13787,.F.);
#18003=ORIENTED_EDGE('',*,*,#13915,.F.);
#18004=ORIENTED_EDGE('',*,*,#13647,.F.);
#18005=ORIENTED_EDGE('',*,*,#13912,.F.);
#18006=ORIENTED_EDGE('',*,*,#13778,.F.);
#18007=ORIENTED_EDGE('',*,*,#13916,.F.);
#18008=ORIENTED_EDGE('',*,*,#13656,.F.);
#18009=ORIENTED_EDGE('',*,*,#13917,.F.);
#18010=ORIENTED_EDGE('',*,*,#13776,.F.);
#18011=ORIENTED_EDGE('',*,*,#13918,.T.);
#18012=ORIENTED_EDGE('',*,*,#13658,.F.);
#18013=ORIENTED_EDGE('',*,*,#13919,.T.);
#18014=ORIENTED_EDGE('',*,*,#13777,.F.);
#18015=ORIENTED_EDGE('',*,*,#13919,.F.);
#18016=ORIENTED_EDGE('',*,*,#13657,.F.);
#18017=ORIENTED_EDGE('',*,*,#13916,.T.);
#18018=ORIENTED_EDGE('',*,*,#13774,.F.);
#18019=ORIENTED_EDGE('',*,*,#13920,.F.);
#18020=ORIENTED_EDGE('',*,*,#13660,.F.);
#18021=ORIENTED_EDGE('',*,*,#13921,.T.);
#18022=ORIENTED_EDGE('',*,*,#13775,.F.);
#18023=ORIENTED_EDGE('',*,*,#13921,.F.);
#18024=ORIENTED_EDGE('',*,*,#13659,.F.);
#18025=ORIENTED_EDGE('',*,*,#13918,.F.);
#18026=ORIENTED_EDGE('',*,*,#13772,.F.);
#18027=ORIENTED_EDGE('',*,*,#13922,.F.);
#18028=ORIENTED_EDGE('',*,*,#13662,.F.);
#18029=ORIENTED_EDGE('',*,*,#13923,.F.);
#18030=ORIENTED_EDGE('',*,*,#13770,.F.);
#18031=ORIENTED_EDGE('',*,*,#13924,.T.);
#18032=ORIENTED_EDGE('',*,*,#13664,.F.);
#18033=ORIENTED_EDGE('',*,*,#13925,.T.);
#18034=ORIENTED_EDGE('',*,*,#13771,.F.);
#18035=ORIENTED_EDGE('',*,*,#13925,.F.);
#18036=ORIENTED_EDGE('',*,*,#13663,.F.);
#18037=ORIENTED_EDGE('',*,*,#13922,.T.);
#18038=ORIENTED_EDGE('',*,*,#13768,.F.);
#18039=ORIENTED_EDGE('',*,*,#13926,.F.);
#18040=ORIENTED_EDGE('',*,*,#13666,.F.);
#18041=ORIENTED_EDGE('',*,*,#13927,.T.);
#18042=ORIENTED_EDGE('',*,*,#13769,.F.);
#18043=ORIENTED_EDGE('',*,*,#13927,.F.);
#18044=ORIENTED_EDGE('',*,*,#13665,.F.);
#18045=ORIENTED_EDGE('',*,*,#13924,.F.);
#18046=ORIENTED_EDGE('',*,*,#13760,.F.);
#18047=ORIENTED_EDGE('',*,*,#13928,.F.);
#18048=ORIENTED_EDGE('',*,*,#13674,.F.);
#18049=ORIENTED_EDGE('',*,*,#13929,.F.);
#18050=ORIENTED_EDGE('',*,*,#13758,.F.);
#18051=ORIENTED_EDGE('',*,*,#13930,.T.);
#18052=ORIENTED_EDGE('',*,*,#13676,.F.);
#18053=ORIENTED_EDGE('',*,*,#13931,.T.);
#18054=ORIENTED_EDGE('',*,*,#13759,.F.);
#18055=ORIENTED_EDGE('',*,*,#13931,.F.);
#18056=ORIENTED_EDGE('',*,*,#13675,.F.);
#18057=ORIENTED_EDGE('',*,*,#13928,.T.);
#18058=ORIENTED_EDGE('',*,*,#13756,.F.);
#18059=ORIENTED_EDGE('',*,*,#13932,.F.);
#18060=ORIENTED_EDGE('',*,*,#13678,.F.);
#18061=ORIENTED_EDGE('',*,*,#13933,.T.);
#18062=ORIENTED_EDGE('',*,*,#13757,.F.);
#18063=ORIENTED_EDGE('',*,*,#13933,.F.);
#18064=ORIENTED_EDGE('',*,*,#13677,.F.);
#18065=ORIENTED_EDGE('',*,*,#13930,.F.);
#18066=ORIENTED_EDGE('',*,*,#13748,.F.);
#18067=ORIENTED_EDGE('',*,*,#13934,.F.);
#18068=ORIENTED_EDGE('',*,*,#13686,.F.);
#18069=ORIENTED_EDGE('',*,*,#13935,.F.);
#18070=ORIENTED_EDGE('',*,*,#13746,.F.);
#18071=ORIENTED_EDGE('',*,*,#13936,.T.);
#18072=ORIENTED_EDGE('',*,*,#13688,.F.);
#18073=ORIENTED_EDGE('',*,*,#13937,.T.);
#18074=ORIENTED_EDGE('',*,*,#13747,.F.);
#18075=ORIENTED_EDGE('',*,*,#13937,.F.);
#18076=ORIENTED_EDGE('',*,*,#13687,.F.);
#18077=ORIENTED_EDGE('',*,*,#13934,.T.);
#18078=ORIENTED_EDGE('',*,*,#13744,.F.);
#18079=ORIENTED_EDGE('',*,*,#13938,.F.);
#18080=ORIENTED_EDGE('',*,*,#13690,.F.);
#18081=ORIENTED_EDGE('',*,*,#13939,.T.);
#18082=ORIENTED_EDGE('',*,*,#13745,.F.);
#18083=ORIENTED_EDGE('',*,*,#13939,.F.);
#18084=ORIENTED_EDGE('',*,*,#13689,.F.);
#18085=ORIENTED_EDGE('',*,*,#13936,.F.);
#18086=ORIENTED_EDGE('',*,*,#13736,.F.);
#18087=ORIENTED_EDGE('',*,*,#13940,.F.);
#18088=ORIENTED_EDGE('',*,*,#13698,.F.);
#18089=ORIENTED_EDGE('',*,*,#13941,.F.);
#18090=ORIENTED_EDGE('',*,*,#13734,.F.);
#18091=ORIENTED_EDGE('',*,*,#13942,.T.);
#18092=ORIENTED_EDGE('',*,*,#13700,.F.);
#18093=ORIENTED_EDGE('',*,*,#13943,.T.);
#18094=ORIENTED_EDGE('',*,*,#13735,.F.);
#18095=ORIENTED_EDGE('',*,*,#13943,.F.);
#18096=ORIENTED_EDGE('',*,*,#13699,.F.);
#18097=ORIENTED_EDGE('',*,*,#13940,.T.);
#18098=ORIENTED_EDGE('',*,*,#13732,.F.);
#18099=ORIENTED_EDGE('',*,*,#13944,.F.);
#18100=ORIENTED_EDGE('',*,*,#13702,.F.);
#18101=ORIENTED_EDGE('',*,*,#13945,.T.);
#18102=ORIENTED_EDGE('',*,*,#13733,.F.);
#18103=ORIENTED_EDGE('',*,*,#13945,.F.);
#18104=ORIENTED_EDGE('',*,*,#13701,.F.);
#18105=ORIENTED_EDGE('',*,*,#13942,.F.);
#18106=ORIENTED_EDGE('',*,*,#13724,.F.);
#18107=ORIENTED_EDGE('',*,*,#13946,.F.);
#18108=ORIENTED_EDGE('',*,*,#13710,.F.);
#18109=ORIENTED_EDGE('',*,*,#13947,.F.);
#18110=ORIENTED_EDGE('',*,*,#13722,.F.);
#18111=ORIENTED_EDGE('',*,*,#13948,.T.);
#18112=ORIENTED_EDGE('',*,*,#13712,.F.);
#18113=ORIENTED_EDGE('',*,*,#13949,.T.);
#18114=ORIENTED_EDGE('',*,*,#13723,.F.);
#18115=ORIENTED_EDGE('',*,*,#13949,.F.);
#18116=ORIENTED_EDGE('',*,*,#13711,.F.);
#18117=ORIENTED_EDGE('',*,*,#13946,.T.);
#18118=ORIENTED_EDGE('',*,*,#13720,.F.);
#18119=ORIENTED_EDGE('',*,*,#13950,.F.);
#18120=ORIENTED_EDGE('',*,*,#13606,.F.);
#18121=ORIENTED_EDGE('',*,*,#13951,.T.);
#18122=ORIENTED_EDGE('',*,*,#13721,.F.);
#18123=ORIENTED_EDGE('',*,*,#13951,.F.);
#18124=ORIENTED_EDGE('',*,*,#13713,.F.);
#18125=ORIENTED_EDGE('',*,*,#13948,.F.);
#18126=ORIENTED_EDGE('',*,*,#13920,.T.);
#18127=ORIENTED_EDGE('',*,*,#13773,.F.);
#18128=ORIENTED_EDGE('',*,*,#13923,.T.);
#18129=ORIENTED_EDGE('',*,*,#13661,.F.);
#18130=ORIENTED_EDGE('',*,*,#13896,.T.);
#18131=ORIENTED_EDGE('',*,*,#13815,.F.);
#18132=ORIENTED_EDGE('',*,*,#13899,.T.);
#18133=ORIENTED_EDGE('',*,*,#13619,.F.);
#18134=ORIENTED_EDGE('',*,*,#13890,.T.);
#18135=ORIENTED_EDGE('',*,*,#13803,.F.);
#18136=ORIENTED_EDGE('',*,*,#13905,.T.);
#18137=ORIENTED_EDGE('',*,*,#13631,.F.);
#18138=ORIENTED_EDGE('',*,*,#13887,.T.);
#18139=ORIENTED_EDGE('',*,*,#13625,.F.);
#18140=ORIENTED_EDGE('',*,*,#13902,.T.);
#18141=ORIENTED_EDGE('',*,*,#13809,.F.);
#18142=ORIENTED_EDGE('',*,*,#13884,.T.);
#18143=ORIENTED_EDGE('',*,*,#13791,.F.);
#18144=ORIENTED_EDGE('',*,*,#13911,.T.);
#18145=ORIENTED_EDGE('',*,*,#13643,.F.);
#18146=ORIENTED_EDGE('',*,*,#13881,.T.);
#18147=ORIENTED_EDGE('',*,*,#13637,.F.);
#18148=ORIENTED_EDGE('',*,*,#13908,.T.);
#18149=ORIENTED_EDGE('',*,*,#13797,.F.);
#18150=ORIENTED_EDGE('',*,*,#13878,.T.);
#18151=ORIENTED_EDGE('',*,*,#13779,.F.);
#18152=ORIENTED_EDGE('',*,*,#13917,.T.);
#18153=ORIENTED_EDGE('',*,*,#13655,.F.);
#18154=ORIENTED_EDGE('',*,*,#13875,.T.);
#18155=ORIENTED_EDGE('',*,*,#13649,.F.);
#18156=ORIENTED_EDGE('',*,*,#13914,.T.);
#18157=ORIENTED_EDGE('',*,*,#13785,.F.);
#18158=ORIENTED_EDGE('',*,*,#13872,.T.);
#18159=ORIENTED_EDGE('',*,*,#13821,.F.);
#18160=ORIENTED_EDGE('',*,*,#13893,.T.);
#18161=ORIENTED_EDGE('',*,*,#13613,.F.);
#18162=ORIENTED_EDGE('',*,*,#13869,.T.);
#18163=ORIENTED_EDGE('',*,*,#13607,.F.);
#18164=ORIENTED_EDGE('',*,*,#13950,.T.);
#18165=ORIENTED_EDGE('',*,*,#13827,.F.);
#18166=ORIENTED_EDGE('',*,*,#13866,.T.);
#18167=ORIENTED_EDGE('',*,*,#13761,.F.);
#18168=ORIENTED_EDGE('',*,*,#13929,.T.);
#18169=ORIENTED_EDGE('',*,*,#13673,.F.);
#18170=ORIENTED_EDGE('',*,*,#13863,.T.);
#18171=ORIENTED_EDGE('',*,*,#13667,.F.);
#18172=ORIENTED_EDGE('',*,*,#13926,.T.);
#18173=ORIENTED_EDGE('',*,*,#13767,.F.);
#18174=ORIENTED_EDGE('',*,*,#13860,.T.);
#18175=ORIENTED_EDGE('',*,*,#13749,.F.);
#18176=ORIENTED_EDGE('',*,*,#13935,.T.);
#18177=ORIENTED_EDGE('',*,*,#13685,.F.);
#18178=ORIENTED_EDGE('',*,*,#13857,.T.);
#18179=ORIENTED_EDGE('',*,*,#13679,.F.);
#18180=ORIENTED_EDGE('',*,*,#13932,.T.);
#18181=ORIENTED_EDGE('',*,*,#13755,.F.);
#18182=ORIENTED_EDGE('',*,*,#13854,.T.);
#18183=ORIENTED_EDGE('',*,*,#13737,.F.);
#18184=ORIENTED_EDGE('',*,*,#13941,.T.);
#18185=ORIENTED_EDGE('',*,*,#13697,.F.);
#18186=ORIENTED_EDGE('',*,*,#13851,.T.);
#18187=ORIENTED_EDGE('',*,*,#13691,.F.);
#18188=ORIENTED_EDGE('',*,*,#13938,.T.);
#18189=ORIENTED_EDGE('',*,*,#13743,.F.);
#18190=ORIENTED_EDGE('',*,*,#13848,.T.);
#18191=ORIENTED_EDGE('',*,*,#13725,.F.);
#18192=ORIENTED_EDGE('',*,*,#13947,.T.);
#18193=ORIENTED_EDGE('',*,*,#13709,.F.);
#18194=ORIENTED_EDGE('',*,*,#13845,.T.);
#18195=ORIENTED_EDGE('',*,*,#13703,.F.);
#18196=ORIENTED_EDGE('',*,*,#13944,.T.);
#18197=ORIENTED_EDGE('',*,*,#13731,.F.);
#25290=CONICAL_SURFACE('',#27055,6.175,0.785398163397445);
#25291=CONICAL_SURFACE('',#27098,6.175,0.785398163397448);
#25292=CONICAL_SURFACE('',#27143,2.95,0.785398163397439);
#25293=CONICAL_SURFACE('',#27149,6.175,0.785398163397442);
#25294=CONICAL_SURFACE('',#27150,6.175,0.785398163397442);
#25295=CONICAL_SURFACE('',#27156,2.95,0.785398163397439);
#25383=ADVANCED_FACE('',(#2570),#25290,.T.);
#25384=ADVANCED_FACE('',(#2571,#845),#1680,.T.);
#25385=ADVANCED_FACE('',(#2572),#518,.T.);
#25386=ADVANCED_FACE('',(#2573),#25291,.T.);
#25387=ADVANCED_FACE('',(#2574,#846),#1681,.T.);
#25388=ADVANCED_FACE('',(#2575),#519,.T.);
#25389=ADVANCED_FACE('',(#2576),#1682,.T.);
#25390=ADVANCED_FACE('',(#2577),#25292,.T.);
#25391=ADVANCED_FACE('',(#2578),#520,.T.);
#25392=ADVANCED_FACE('',(#2579,#847),#1683,.T.);
#25393=ADVANCED_FACE('',(#2580),#25293,.T.);
#25394=ADVANCED_FACE('',(#2581),#25294,.T.);
#25395=ADVANCED_FACE('',(#2582,#848),#1684,.T.);
#25396=ADVANCED_FACE('',(#2583),#521,.T.);
#25397=ADVANCED_FACE('',(#2584),#25295,.T.);
#25398=ADVANCED_FACE('',(#2585),#1685,.T.);
#25399=ADVANCED_FACE('',(#2586),#482,.F.);
#25400=ADVANCED_FACE('',(#2587),#522,.T.);
#25401=ADVANCED_FACE('',(#2588),#1686,.F.);
#25402=ADVANCED_FACE('',(#2589),#483,.F.);
#25403=ADVANCED_FACE('',(#2590),#1687,.F.);
#25404=ADVANCED_FACE('',(#2591),#484,.F.);
#25405=ADVANCED_FACE('',(#2592),#523,.T.);
#25406=ADVANCED_FACE('',(#2593),#1688,.F.);
#25407=ADVANCED_FACE('',(#2594),#485,.F.);
#25408=ADVANCED_FACE('',(#2595),#1689,.F.);
#25409=ADVANCED_FACE('',(#2596),#486,.F.);
#25410=ADVANCED_FACE('',(#2597),#524,.T.);
#25411=ADVANCED_FACE('',(#2598),#1690,.F.);
#25412=ADVANCED_FACE('',(#2599),#487,.F.);
#25413=ADVANCED_FACE('',(#2600),#1691,.F.);
#25414=ADVANCED_FACE('',(#2601),#488,.F.);
#25415=ADVANCED_FACE('',(#2602),#525,.T.);
#25416=ADVANCED_FACE('',(#2603),#1692,.F.);
#25417=ADVANCED_FACE('',(#2604),#489,.F.);
#25418=ADVANCED_FACE('',(#2605),#1693,.F.);
#25419=ADVANCED_FACE('',(#2606),#490,.F.);
#25420=ADVANCED_FACE('',(#2607),#526,.T.);
#25421=ADVANCED_FACE('',(#2608),#1694,.F.);
#25422=ADVANCED_FACE('',(#2609),#491,.F.);
#25423=ADVANCED_FACE('',(#2610),#1695,.F.);
#25424=ADVANCED_FACE('',(#2611),#492,.F.);
#25425=ADVANCED_FACE('',(#2612),#527,.T.);
#25426=ADVANCED_FACE('',(#2613),#1696,.F.);
#25427=ADVANCED_FACE('',(#2614),#493,.F.);
#25428=ADVANCED_FACE('',(#2615),#1697,.F.);
#25429=ADVANCED_FACE('',(#2616),#494,.F.);
#25430=ADVANCED_FACE('',(#2617),#528,.T.);
#25431=ADVANCED_FACE('',(#2618),#1698,.F.);
#25432=ADVANCED_FACE('',(#2619),#495,.F.);
#25433=ADVANCED_FACE('',(#2620),#1699,.F.);
#25434=ADVANCED_FACE('',(#2621),#496,.F.);
#25435=ADVANCED_FACE('',(#2622),#529,.T.);
#25436=ADVANCED_FACE('',(#2623),#1700,.F.);
#25437=ADVANCED_FACE('',(#2624),#497,.F.);
#25438=ADVANCED_FACE('',(#2625),#1701,.F.);
#25439=ADVANCED_FACE('',(#2626),#498,.F.);
#25440=ADVANCED_FACE('',(#2627),#530,.T.);
#25441=ADVANCED_FACE('',(#2628),#1702,.F.);
#25442=ADVANCED_FACE('',(#2629),#499,.F.);
#25443=ADVANCED_FACE('',(#2630),#1703,.F.);
#25444=ADVANCED_FACE('',(#2631),#500,.F.);
#25445=ADVANCED_FACE('',(#2632),#531,.T.);
#25446=ADVANCED_FACE('',(#2633),#1704,.F.);
#25447=ADVANCED_FACE('',(#2634),#501,.F.);
#25448=ADVANCED_FACE('',(#2635),#1705,.F.);
#25449=ADVANCED_FACE('',(#2636),#502,.F.);
#25450=ADVANCED_FACE('',(#2637),#532,.T.);
#25451=ADVANCED_FACE('',(#2638),#1706,.F.);
#25452=ADVANCED_FACE('',(#2639),#503,.F.);
#25453=ADVANCED_FACE('',(#2640),#1707,.F.);
#25454=ADVANCED_FACE('',(#2641),#504,.F.);
#25455=ADVANCED_FACE('',(#2642),#533,.T.);
#25456=ADVANCED_FACE('',(#2643),#1708,.F.);
#25457=ADVANCED_FACE('',(#2644),#505,.F.);
#25458=ADVANCED_FACE('',(#2645),#1709,.F.);
#25459=ADVANCED_FACE('',(#2646),#506,.F.);
#25460=ADVANCED_FACE('',(#2647),#534,.T.);
#25461=ADVANCED_FACE('',(#2648),#1710,.F.);
#25462=ADVANCED_FACE('',(#2649),#507,.F.);
#25463=ADVANCED_FACE('',(#2650),#1711,.F.);
#25464=ADVANCED_FACE('',(#2651),#508,.F.);
#25465=ADVANCED_FACE('',(#2652),#535,.T.);
#25466=ADVANCED_FACE('',(#2653),#1712,.F.);
#25467=ADVANCED_FACE('',(#2654),#509,.F.);
#25468=ADVANCED_FACE('',(#2655),#1713,.F.);
#25469=ADVANCED_FACE('',(#2656),#510,.F.);
#25470=ADVANCED_FACE('',(#2657),#536,.T.);
#25471=ADVANCED_FACE('',(#2658),#1714,.F.);
#25472=ADVANCED_FACE('',(#2659),#511,.F.);
#25473=ADVANCED_FACE('',(#2660),#1715,.F.);
#25474=ADVANCED_FACE('',(#2661),#512,.F.);
#25475=ADVANCED_FACE('',(#2662),#537,.T.);
#25476=ADVANCED_FACE('',(#2663),#1716,.F.);
#25477=ADVANCED_FACE('',(#2664),#513,.F.);
#25478=ADVANCED_FACE('',(#2665),#1717,.F.);
#25479=ADVANCED_FACE('',(#2666),#514,.F.);
#25480=ADVANCED_FACE('',(#2667),#538,.T.);
#25481=ADVANCED_FACE('',(#2668),#1718,.F.);
#25482=ADVANCED_FACE('',(#2669),#515,.F.);
#25483=ADVANCED_FACE('',(#2670),#1719,.F.);
#25484=ADVANCED_FACE('',(#2671),#516,.F.);
#25485=ADVANCED_FACE('',(#2672),#539,.T.);
#25486=ADVANCED_FACE('',(#2673),#1720,.F.);
#25487=ADVANCED_FACE('',(#2674),#517,.F.);
#25488=ADVANCED_FACE('',(#2675),#1721,.F.);
#25489=ADVANCED_FACE('',(#2676),#540,.T.);
#25490=ADVANCED_FACE('',(#2677),#541,.T.);
#25491=ADVANCED_FACE('',(#2678),#542,.T.);
#25492=ADVANCED_FACE('',(#2679),#543,.T.);
#25493=ADVANCED_FACE('',(#2680),#544,.T.);
#25494=ADVANCED_FACE('',(#2681),#545,.T.);
#25495=ADVANCED_FACE('',(#2682),#546,.T.);
#25496=ADVANCED_FACE('',(#2683),#547,.T.);
#25497=ADVANCED_FACE('',(#2684),#548,.T.);
#25498=ADVANCED_FACE('',(#2685),#549,.T.);
#25499=ADVANCED_FACE('',(#2686),#550,.T.);
#25500=ADVANCED_FACE('',(#2687),#551,.T.);
#25501=ADVANCED_FACE('',(#2688),#552,.T.);
#25502=ADVANCED_FACE('',(#2689),#553,.T.);
#25503=ADVANCED_FACE('',(#2690),#554,.T.);
#25504=ADVANCED_FACE('',(#2691),#555,.T.);
#25505=ADVANCED_FACE('',(#2692),#556,.T.);
#25506=ADVANCED_FACE('',(#2693),#557,.T.);
#26872=CLOSED_SHELL('',(#25383,#25384,#25385,#25386,#25387,#25388,#25389,
#25390,#25391,#25392,#25393,#25394,#25395,#25396,#25397,#25398,#25399,#25400,
#25401,#25402,#25403,#25404,#25405,#25406,#25407,#25408,#25409,#25410,#25411,
#25412,#25413,#25414,#25415,#25416,#25417,#25418,#25419,#25420,#25421,#25422,
#25423,#25424,#25425,#25426,#25427,#25428,#25429,#25430,#25431,#25432,#25433,
#25434,#25435,#25436,#25437,#25438,#25439,#25440,#25441,#25442,#25443,#25444,
#25445,#25446,#25447,#25448,#25449,#25450,#25451,#25452,#25453,#25454,#25455,
#25456,#25457,#25458,#25459,#25460,#25461,#25462,#25463,#25464,#25465,#25466,
#25467,#25468,#25469,#25470,#25471,#25472,#25473,#25474,#25475,#25476,#25477,
#25478,#25479,#25480,#25481,#25482,#25483,#25484,#25485,#25486,#25487,#25488,
#25489,#25490,#25491,#25492,#25493,#25494,#25495,#25496,#25497,#25498,#25499,
#25500,#25501,#25502,#25503,#25504,#25505,#25506));
#27054=AXIS2_PLACEMENT_3D('',#35347,#28987,#28988);
#27055=AXIS2_PLACEMENT_3D('',#35348,#28989,#28990);
#27056=AXIS2_PLACEMENT_3D('',#35351,#28991,#28992);
#27057=AXIS2_PLACEMENT_3D('',#35352,#28993,#28994);
#27058=AXIS2_PLACEMENT_3D('',#35355,#28996,#28997);
#27059=AXIS2_PLACEMENT_3D('',#35356,#28998,#28999);
#27060=AXIS2_PLACEMENT_3D('',#35368,#29000,#29001);
#27061=AXIS2_PLACEMENT_3D('',#35419,#29003,#29004);
#27062=AXIS2_PLACEMENT_3D('',#35432,#29006,#29007);
#27063=AXIS2_PLACEMENT_3D('',#35483,#29009,#29010);
#27064=AXIS2_PLACEMENT_3D('',#35496,#29012,#29013);
#27065=AXIS2_PLACEMENT_3D('',#35509,#29015,#29016);
#27066=AXIS2_PLACEMENT_3D('',#35522,#29018,#29019);
#27067=AXIS2_PLACEMENT_3D('',#35535,#29021,#29022);
#27068=AXIS2_PLACEMENT_3D('',#35548,#29024,#29025);
#27069=AXIS2_PLACEMENT_3D('',#35599,#29027,#29028);
#27070=AXIS2_PLACEMENT_3D('',#35612,#29030,#29031);
#27071=AXIS2_PLACEMENT_3D('',#35663,#29033,#29034);
#27072=AXIS2_PLACEMENT_3D('',#35676,#29036,#29037);
#27073=AXIS2_PLACEMENT_3D('',#35727,#29039,#29040);
#27074=AXIS2_PLACEMENT_3D('',#35740,#29042,#29043);
#27075=AXIS2_PLACEMENT_3D('',#35791,#29045,#29046);
#27076=AXIS2_PLACEMENT_3D('',#35804,#29048,#29049);
#27077=AXIS2_PLACEMENT_3D('',#35855,#29051,#29052);
#27078=AXIS2_PLACEMENT_3D('',#35868,#29054,#29055);
#27079=AXIS2_PLACEMENT_3D('',#35879,#29057,#29058);
#27080=AXIS2_PLACEMENT_3D('',#35892,#29060,#29061);
#27081=AXIS2_PLACEMENT_3D('',#35905,#29063,#29064);
#27082=AXIS2_PLACEMENT_3D('',#35918,#29066,#29067);
#27083=AXIS2_PLACEMENT_3D('',#35969,#29069,#29070);
#27084=AXIS2_PLACEMENT_3D('',#35982,#29072,#29073);
#27085=AXIS2_PLACEMENT_3D('',#36033,#29075,#29076);
#27086=AXIS2_PLACEMENT_3D('',#36046,#29078,#29079);
#27087=AXIS2_PLACEMENT_3D('',#36097,#29081,#29082);
#27088=AXIS2_PLACEMENT_3D('',#36110,#29084,#29085);
#27089=AXIS2_PLACEMENT_3D('',#36161,#29087,#29088);
#27090=AXIS2_PLACEMENT_3D('',#36174,#29090,#29091);
#27091=AXIS2_PLACEMENT_3D('',#36225,#29093,#29094);
#27092=AXIS2_PLACEMENT_3D('',#36238,#29096,#29097);
#27093=AXIS2_PLACEMENT_3D('',#36289,#29099,#29100);
#27094=AXIS2_PLACEMENT_3D('',#36302,#29102,#29103);
#27095=AXIS2_PLACEMENT_3D('',#36353,#29105,#29106);
#27096=AXIS2_PLACEMENT_3D('',#36355,#29108,#29109);
#27097=AXIS2_PLACEMENT_3D('',#36357,#29110,#29111);
#27098=AXIS2_PLACEMENT_3D('',#36359,#29113,#29114);
#27099=AXIS2_PLACEMENT_3D('',#36361,#29115,#29116);
#27100=AXIS2_PLACEMENT_3D('',#36365,#29118,#29119);
#27101=AXIS2_PLACEMENT_3D('',#36366,#29120,#29121);
#27102=AXIS2_PLACEMENT_3D('',#36367,#29122,#29123);
#27103=AXIS2_PLACEMENT_3D('',#36419,#29125,#29126);
#27104=AXIS2_PLACEMENT_3D('',#36432,#29128,#29129);
#27105=AXIS2_PLACEMENT_3D('',#36483,#29131,#29132);
#27106=AXIS2_PLACEMENT_3D('',#36496,#29134,#29135);
#27107=AXIS2_PLACEMENT_3D('',#36547,#29137,#29138);
#27108=AXIS2_PLACEMENT_3D('',#36560,#29140,#29141);
#27109=AXIS2_PLACEMENT_3D('',#36611,#29143,#29144);
#27110=AXIS2_PLACEMENT_3D('',#36624,#29146,#29147);
#27111=AXIS2_PLACEMENT_3D('',#36637,#29149,#29150);
#27112=AXIS2_PLACEMENT_3D('',#36650,#29152,#29153);
#27113=AXIS2_PLACEMENT_3D('',#36701,#29155,#29156);
#27114=AXIS2_PLACEMENT_3D('',#36714,#29158,#29159);
#27115=AXIS2_PLACEMENT_3D('',#36765,#29161,#29162);
#27116=AXIS2_PLACEMENT_3D('',#36778,#29164,#29165);
#27117=AXIS2_PLACEMENT_3D('',#36829,#29167,#29168);
#27118=AXIS2_PLACEMENT_3D('',#36842,#29170,#29171);
#27119=AXIS2_PLACEMENT_3D('',#36893,#29173,#29174);
#27120=AXIS2_PLACEMENT_3D('',#36906,#29176,#29177);
#27121=AXIS2_PLACEMENT_3D('',#36957,#29179,#29180);
#27122=AXIS2_PLACEMENT_3D('',#36970,#29182,#29183);
#27123=AXIS2_PLACEMENT_3D('',#36983,#29185,#29186);
#27124=AXIS2_PLACEMENT_3D('',#36996,#29188,#29189);
#27125=AXIS2_PLACEMENT_3D('',#37047,#29191,#29192);
#27126=AXIS2_PLACEMENT_3D('',#37060,#29194,#29195);
#27127=AXIS2_PLACEMENT_3D('',#37111,#29197,#29198);
#27128=AXIS2_PLACEMENT_3D('',#37124,#29200,#29201);
#27129=AXIS2_PLACEMENT_3D('',#37175,#29203,#29204);
#27130=AXIS2_PLACEMENT_3D('',#37188,#29206,#29207);
#27131=AXIS2_PLACEMENT_3D('',#37201,#29209,#29210);
#27132=AXIS2_PLACEMENT_3D('',#37214,#29212,#29213);
#27133=AXIS2_PLACEMENT_3D('',#37265,#29215,#29216);
#27134=AXIS2_PLACEMENT_3D('',#37278,#29218,#29219);
#27135=AXIS2_PLACEMENT_3D('',#37329,#29221,#29222);
#27136=AXIS2_PLACEMENT_3D('',#37342,#29224,#29225);
#27137=AXIS2_PLACEMENT_3D('',#37393,#29227,#29228);
#27138=AXIS2_PLACEMENT_3D('',#37405,#29230,#29231);
#27139=AXIS2_PLACEMENT_3D('',#37406,#29232,#29233);
#27140=AXIS2_PLACEMENT_3D('',#37409,#29235,#29236);
#27141=AXIS2_PLACEMENT_3D('',#37410,#29237,#29238);
#27142=AXIS2_PLACEMENT_3D('',#37412,#29239,#29240);
#27143=AXIS2_PLACEMENT_3D('',#37413,#29241,#29242);
#27144=AXIS2_PLACEMENT_3D('',#37415,#29243,#29244);
#27145=AXIS2_PLACEMENT_3D('',#37417,#29246,#29247);
#27146=AXIS2_PLACEMENT_3D('',#37419,#29248,#29249);
#27147=AXIS2_PLACEMENT_3D('',#37421,#29251,#29252);
#27148=AXIS2_PLACEMENT_3D('',#37423,#29253,#29254);
#27149=AXIS2_PLACEMENT_3D('',#37424,#29255,#29256);
#27150=AXIS2_PLACEMENT_3D('',#37426,#29258,#29259);
#27151=AXIS2_PLACEMENT_3D('',#37428,#29260,#29261);
#27152=AXIS2_PLACEMENT_3D('',#37430,#29263,#29264);
#27153=AXIS2_PLACEMENT_3D('',#37432,#29265,#29266);
#27154=AXIS2_PLACEMENT_3D('',#37433,#29267,#29268);
#27155=AXIS2_PLACEMENT_3D('',#37435,#29269,#29270);
#27156=AXIS2_PLACEMENT_3D('',#37437,#29272,#29273);
#27157=AXIS2_PLACEMENT_3D('',#37439,#29274,#29275);
#27158=AXIS2_PLACEMENT_3D('',#37441,#29277,#29278);
#27159=AXIS2_PLACEMENT_3D('',#37519,#29280,#29281);
#27160=AXIS2_PLACEMENT_3D('',#37522,#29284,#29285);
#27161=AXIS2_PLACEMENT_3D('',#37600,#29287,#29288);
#27162=AXIS2_PLACEMENT_3D('',#37678,#29290,#29291);
#27163=AXIS2_PLACEMENT_3D('',#37681,#29294,#29295);
#27164=AXIS2_PLACEMENT_3D('',#37759,#29297,#29298);
#27165=AXIS2_PLACEMENT_3D('',#37837,#29300,#29301);
#27166=AXIS2_PLACEMENT_3D('',#37840,#29304,#29305);
#27167=AXIS2_PLACEMENT_3D('',#37918,#29307,#29308);
#27168=AXIS2_PLACEMENT_3D('',#37996,#29310,#29311);
#27169=AXIS2_PLACEMENT_3D('',#37999,#29314,#29315);
#27170=AXIS2_PLACEMENT_3D('',#38077,#29317,#29318);
#27171=AXIS2_PLACEMENT_3D('',#38155,#29320,#29321);
#27172=AXIS2_PLACEMENT_3D('',#38158,#29324,#29325);
#27173=AXIS2_PLACEMENT_3D('',#38236,#29327,#29328);
#27174=AXIS2_PLACEMENT_3D('',#38314,#29330,#29331);
#27175=AXIS2_PLACEMENT_3D('',#38317,#29334,#29335);
#27176=AXIS2_PLACEMENT_3D('',#38395,#29337,#29338);
#27177=AXIS2_PLACEMENT_3D('',#38473,#29340,#29341);
#27178=AXIS2_PLACEMENT_3D('',#38476,#29344,#29345);
#27179=AXIS2_PLACEMENT_3D('',#38554,#29347,#29348);
#27180=AXIS2_PLACEMENT_3D('',#38632,#29350,#29351);
#27181=AXIS2_PLACEMENT_3D('',#38635,#29354,#29355);
#27182=AXIS2_PLACEMENT_3D('',#38713,#29357,#29358);
#27183=AXIS2_PLACEMENT_3D('',#38791,#29360,#29361);
#27184=AXIS2_PLACEMENT_3D('',#38794,#29364,#29365);
#27185=AXIS2_PLACEMENT_3D('',#38872,#29367,#29368);
#27186=AXIS2_PLACEMENT_3D('',#38950,#29370,#29371);
#27187=AXIS2_PLACEMENT_3D('',#38953,#29374,#29375);
#27188=AXIS2_PLACEMENT_3D('',#39031,#29377,#29378);
#27189=AXIS2_PLACEMENT_3D('',#39109,#29380,#29381);
#27190=AXIS2_PLACEMENT_3D('',#39112,#29384,#29385);
#27191=AXIS2_PLACEMENT_3D('',#39190,#29387,#29388);
#27192=AXIS2_PLACEMENT_3D('',#39268,#29390,#29391);
#27193=AXIS2_PLACEMENT_3D('',#39271,#29394,#29395);
#27194=AXIS2_PLACEMENT_3D('',#39349,#29397,#29398);
#27195=AXIS2_PLACEMENT_3D('',#39427,#29400,#29401);
#27196=AXIS2_PLACEMENT_3D('',#39430,#29404,#29405);
#27197=AXIS2_PLACEMENT_3D('',#39508,#29407,#29408);
#27198=AXIS2_PLACEMENT_3D('',#39586,#29410,#29411);
#27199=AXIS2_PLACEMENT_3D('',#39589,#29414,#29415);
#27200=AXIS2_PLACEMENT_3D('',#39667,#29417,#29418);
#27201=AXIS2_PLACEMENT_3D('',#39745,#29420,#29421);
#27202=AXIS2_PLACEMENT_3D('',#39748,#29424,#29425);
#27203=AXIS2_PLACEMENT_3D('',#39826,#29427,#29428);
#27204=AXIS2_PLACEMENT_3D('',#39904,#29430,#29431);
#27205=AXIS2_PLACEMENT_3D('',#39907,#29434,#29435);
#27206=AXIS2_PLACEMENT_3D('',#39985,#29437,#29438);
#27207=AXIS2_PLACEMENT_3D('',#40063,#29440,#29441);
#27208=AXIS2_PLACEMENT_3D('',#40066,#29444,#29445);
#27209=AXIS2_PLACEMENT_3D('',#40144,#29447,#29448);
#27210=AXIS2_PLACEMENT_3D('',#40222,#29450,#29451);
#27211=AXIS2_PLACEMENT_3D('',#40225,#29454,#29455);
#27212=AXIS2_PLACEMENT_3D('',#40303,#29457,#29458);
#27213=AXIS2_PLACEMENT_3D('',#40304,#29459,#29460);
#27214=AXIS2_PLACEMENT_3D('',#40305,#29461,#29462);
#27215=AXIS2_PLACEMENT_3D('',#40306,#29463,#29464);
#27216=AXIS2_PLACEMENT_3D('',#40307,#29465,#29466);
#27217=AXIS2_PLACEMENT_3D('',#40308,#29467,#29468);
#27218=AXIS2_PLACEMENT_3D('',#40309,#29469,#29470);
#27219=AXIS2_PLACEMENT_3D('',#40310,#29471,#29472);
#27220=AXIS2_PLACEMENT_3D('',#40311,#29473,#29474);
#27221=AXIS2_PLACEMENT_3D('',#40312,#29475,#29476);
#27222=AXIS2_PLACEMENT_3D('',#40313,#29477,#29478);
#27223=AXIS2_PLACEMENT_3D('',#40314,#29479,#29480);
#27224=AXIS2_PLACEMENT_3D('',#40315,#29481,#29482);
#27225=AXIS2_PLACEMENT_3D('',#40316,#29483,#29484);
#27226=AXIS2_PLACEMENT_3D('',#40317,#29485,#29486);
#27227=AXIS2_PLACEMENT_3D('',#40318,#29487,#29488);
#27228=AXIS2_PLACEMENT_3D('',#40319,#29489,#29490);
#27229=AXIS2_PLACEMENT_3D('',#40320,#29491,#29492);
#27230=AXIS2_PLACEMENT_3D('',#40321,#29493,#29494);
#28987=DIRECTION('axis',(0.,0.,1.));
#28988=DIRECTION('refdir',(1.,0.,0.));
#28989=DIRECTION('center_axis',(0.,-1.,0.));
#28990=DIRECTION('ref_axis',(-1.,0.,0.));
#28991=DIRECTION('center_axis',(0.,1.,0.));
#28992=DIRECTION('ref_axis',(-1.,0.,0.));
#28993=DIRECTION('center_axis',(0.,1.,0.));
#28994=DIRECTION('ref_axis',(-1.,0.,0.));
#28995=DIRECTION('',(-0.707106781186545,0.70710678118655,-8.65956056235491E-17));
#28996=DIRECTION('center_axis',(0.,-1.,0.));
#28997=DIRECTION('ref_axis',(-1.,0.,0.));
#28998=DIRECTION('center_axis',(0.,1.,0.));
#28999=DIRECTION('ref_axis',(0.,0.,1.));
#29000=DIRECTION('center_axis',(0.,-1.,0.));
#29001=DIRECTION('ref_axis',(1.,0.,0.));
#29002=DIRECTION('',(0.973234235146997,0.,0.229815411880577));
#29003=DIRECTION('center_axis',(0.,-1.,0.));
#29004=DIRECTION('ref_axis',(-0.966435998091082,0.,-0.256907496180421));
#29005=DIRECTION('',(-0.993142529173694,0.,-0.116909865907365));
#29006=DIRECTION('center_axis',(0.,-1.,0.));
#29007=DIRECTION('ref_axis',(1.,0.,0.));
#29008=DIRECTION('',(0.835939528954007,0.,0.548821559281478));
#29009=DIRECTION('center_axis',(0.,-1.,0.));
#29010=DIRECTION('ref_axis',(-0.820285237202974,0.,-0.571954656967543));
#29011=DIRECTION('',(-0.89326317695935,0.,-0.449534088461031));
#29012=DIRECTION('center_axis',(0.,-1.,0.));
#29013=DIRECTION('ref_axis',(1.,0.,0.));
#29014=DIRECTION('',(0.597818178415661,0.,0.801631726889462));
#29015=DIRECTION('center_axis',(0.,-1.,0.));
#29016=DIRECTION('ref_axis',(-0.575195970587437,0.,-0.818015644972623));
#29017=DIRECTION('',(-0.685643102443273,0.,-0.727937865529719));
#29018=DIRECTION('center_axis',(0.,-1.,0.));
#29019=DIRECTION('ref_axis',(1.,0.,0.));
#29020=DIRECTION('',(0.287591132703732,0.,0.957753277410307));
#29021=DIRECTION('center_axis',(0.,-1.,0.));
#29022=DIRECTION('ref_axis',(-0.260729580930624,0.,-0.965411873568862));
#29023=DIRECTION('',(-0.395324350758037,0.,-0.918541592796829));
#29024=DIRECTION('center_axis',(0.,-1.,0.));
#29025=DIRECTION('ref_axis',(1.,0.,0.));
#29026=DIRECTION('',(-0.0573236480053483,0.,0.998355647742506));
#29027=DIRECTION('center_axis',(0.,-1.,0.));
#29028=DIRECTION('ref_axis',(0.0851846441452059,0.,-0.996365182250893));
#29029=DIRECTION('',(-0.0573236480053483,0.,-0.998355647742506));
#29030=DIRECTION('center_axis',(0.,-1.,0.));
#29031=DIRECTION('ref_axis',(1.,0.,0.));
#29032=DIRECTION('',(-0.395324350758034,0.,0.918541592796831));
#29033=DIRECTION('center_axis',(0.,-1.,0.));
#29034=DIRECTION('ref_axis',(0.420824343945678,0.,-0.907142145169482));
#29035=DIRECTION('',(0.287591132703732,0.,-0.957753277410307));
#29036=DIRECTION('center_axis',(0.,-1.,0.));
#29037=DIRECTION('ref_axis',(1.,0.,0.));
#29038=DIRECTION('',(-0.68564310244327,0.,0.727937865529722));
#29039=DIRECTION('center_axis',(0.,-1.,0.));
#29040=DIRECTION('ref_axis',(0.705706417160429,0.,-0.708504377388447));
#29041=DIRECTION('',(0.597818178415657,0.,-0.801631726889465));
#29042=DIRECTION('center_axis',(0.,-1.,0.));
#29043=DIRECTION('ref_axis',(1.,0.,0.));
#29044=DIRECTION('',(-0.893263176959351,0.,0.449534088461028));
#29045=DIRECTION('center_axis',(0.,-1.,0.));
#29046=DIRECTION('ref_axis',(0.9054698813482,0.,-0.424410525283336));
#29047=DIRECTION('',(0.835939528953991,0.,-0.548821559281502));
#29048=DIRECTION('center_axis',(0.,-1.,0.));
#29049=DIRECTION('ref_axis',(1.,0.,0.));
#29050=DIRECTION('',(-0.993142529173694,0.,0.116909865907364));
#29051=DIRECTION('center_axis',(0.,-1.,0.));
#29052=DIRECTION('ref_axis',(0.996020314533121,0.,-0.0891265001968739));
#29053=DIRECTION('',(0.973234235146997,0.,-0.229815411880577));
#29054=DIRECTION('center_axis',(0.,-1.,0.));
#29055=DIRECTION('ref_axis',(1.,0.,0.));
#29056=DIRECTION('',(-0.973234235146997,0.,-0.229815411880577));
#29057=DIRECTION('center_axis',(0.,-1.,0.));
#29058=DIRECTION('ref_axis',(0.966435998091084,0.,0.256907496180414));
#29059=DIRECTION('',(0.993142529173694,0.,0.116909865907365));
#29060=DIRECTION('center_axis',(0.,-1.,0.));
#29061=DIRECTION('ref_axis',(1.,0.,0.));
#29062=DIRECTION('',(-0.835939528954005,0.,-0.548821559281481));
#29063=DIRECTION('center_axis',(0.,-1.,0.));
#29064=DIRECTION('ref_axis',(0.820285237202979,0.,0.571954656967538));
#29065=DIRECTION('',(0.89326317695935,0.,0.44953408846103));
#29066=DIRECTION('center_axis',(0.,-1.,0.));
#29067=DIRECTION('ref_axis',(1.,0.,0.));
#29068=DIRECTION('',(-0.597818178415659,0.,-0.801631726889463));
#29069=DIRECTION('center_axis',(0.,-1.,0.));
#29070=DIRECTION('ref_axis',(0.575195970587441,0.,0.818015644972621));
#29071=DIRECTION('',(0.685643102443272,0.,0.72793786552972));
#29072=DIRECTION('center_axis',(0.,-1.,0.));
#29073=DIRECTION('ref_axis',(1.,0.,0.));
#29074=DIRECTION('',(-0.287591132703736,0.,-0.957753277410306));
#29075=DIRECTION('center_axis',(0.,-1.,0.));
#29076=DIRECTION('ref_axis',(0.260729580930626,0.,0.965411873568862));
#29077=DIRECTION('',(0.395324350758034,0.,0.918541592796831));
#29078=DIRECTION('center_axis',(0.,-1.,0.));
#29079=DIRECTION('ref_axis',(1.,0.,0.));
#29080=DIRECTION('',(0.0573236480053483,0.,-0.998355647742506));
#29081=DIRECTION('center_axis',(0.,-1.,0.));
#29082=DIRECTION('ref_axis',(-0.0851846441452059,0.,0.996365182250893));
#29083=DIRECTION('',(0.0573236480053525,0.,0.998355647742506));
#29084=DIRECTION('center_axis',(0.,-1.,0.));
#29085=DIRECTION('ref_axis',(1.,0.,0.));
#29086=DIRECTION('',(0.395324350758046,0.,-0.918541592796826));
#29087=DIRECTION('center_axis',(0.,-1.,0.));
#29088=DIRECTION('ref_axis',(-0.420824343945662,0.,0.907142145169489));
#29089=DIRECTION('',(-0.287591132703732,0.,0.957753277410307));
#29090=DIRECTION('center_axis',(0.,-1.,0.));
#29091=DIRECTION('ref_axis',(1.,0.,0.));
#29092=DIRECTION('',(0.685643102443271,0.,-0.727937865529721));
#29093=DIRECTION('center_axis',(0.,-1.,0.));
#29094=DIRECTION('ref_axis',(-0.705706417160429,0.,0.708504377388447));
#29095=DIRECTION('',(-0.597818178415657,0.,0.801631726889465));
#29096=DIRECTION('center_axis',(0.,-1.,0.));
#29097=DIRECTION('ref_axis',(1.,0.,0.));
#29098=DIRECTION('',(0.89326317695935,0.,-0.44953408846103));
#29099=DIRECTION('center_axis',(0.,-1.,0.));
#29100=DIRECTION('ref_axis',(-0.905469881348196,0.,0.424410525283343));
#29101=DIRECTION('',(-0.835939528953991,0.,0.548821559281503));
#29102=DIRECTION('center_axis',(0.,-1.,0.));
#29103=DIRECTION('ref_axis',(1.,0.,0.));
#29104=DIRECTION('',(0.993142529173694,0.,-0.116909865907365));
#29105=DIRECTION('center_axis',(0.,-1.,0.));
#29106=DIRECTION('ref_axis',(-0.996020314533121,0.,0.0891265001968672));
#29107=DIRECTION('',(-0.973234235146997,0.,0.229815411880577));
#29108=DIRECTION('center_axis',(0.,-1.,0.));
#29109=DIRECTION('ref_axis',(1.,0.,0.));
#29110=DIRECTION('center_axis',(0.,-1.,0.));
#29111=DIRECTION('ref_axis',(1.,0.,0.));
#29112=DIRECTION('',(0.,1.,0.));
#29113=DIRECTION('center_axis',(0.,1.,0.));
#29114=DIRECTION('ref_axis',(-1.,0.,0.));
#29115=DIRECTION('center_axis',(0.,1.,0.));
#29116=DIRECTION('ref_axis',(-1.,0.,0.));
#29117=DIRECTION('',(0.707106781186548,0.707106781186548,8.65956056235493E-17));
#29118=DIRECTION('center_axis',(0.,-1.,0.));
#29119=DIRECTION('ref_axis',(-1.,0.,0.));
#29120=DIRECTION('center_axis',(0.,-1.,0.));
#29121=DIRECTION('ref_axis',(-1.,0.,0.));
#29122=DIRECTION('center_axis',(0.,-1.,0.));
#29123=DIRECTION('ref_axis',(0.,0.,-1.));
#29124=DIRECTION('',(0.973234235146997,0.,-0.229815411880577));
#29125=DIRECTION('center_axis',(0.,1.,0.));
#29126=DIRECTION('ref_axis',(-0.996020314533121,0.,0.0891265001968672));
#29127=DIRECTION('',(-0.993142529173694,0.,0.116909865907365));
#29128=DIRECTION('center_axis',(0.,1.,0.));
#29129=DIRECTION('ref_axis',(1.,0.,0.));
#29130=DIRECTION('',(0.835939528953991,0.,-0.548821559281503));
#29131=DIRECTION('center_axis',(0.,1.,0.));
#29132=DIRECTION('ref_axis',(-0.905469881348196,0.,0.424410525283343));
#29133=DIRECTION('',(-0.89326317695935,0.,0.44953408846103));
#29134=DIRECTION('center_axis',(0.,1.,0.));
#29135=DIRECTION('ref_axis',(1.,0.,0.));
#29136=DIRECTION('',(0.597818178415657,0.,-0.801631726889465));
#29137=DIRECTION('center_axis',(0.,1.,0.));
#29138=DIRECTION('ref_axis',(-0.705706417160429,0.,0.708504377388447));
#29139=DIRECTION('',(-0.685643102443271,0.,0.727937865529721));
#29140=DIRECTION('center_axis',(0.,1.,0.));
#29141=DIRECTION('ref_axis',(1.,0.,0.));
#29142=DIRECTION('',(0.287591132703732,0.,-0.957753277410307));
#29143=DIRECTION('center_axis',(0.,1.,0.));
#29144=DIRECTION('ref_axis',(-0.420824343945662,0.,0.907142145169489));
#29145=DIRECTION('',(-0.395324350758046,0.,0.918541592796826));
#29146=DIRECTION('center_axis',(0.,1.,0.));
#29147=DIRECTION('ref_axis',(1.,0.,0.));
#29148=DIRECTION('',(-0.0573236480053525,0.,-0.998355647742506));
#29149=DIRECTION('center_axis',(0.,1.,0.));
#29150=DIRECTION('ref_axis',(-0.0851846441452059,0.,0.996365182250893));
#29151=DIRECTION('',(-0.0573236480053483,0.,0.998355647742506));
#29152=DIRECTION('center_axis',(0.,1.,0.));
#29153=DIRECTION('ref_axis',(1.,0.,0.));
#29154=DIRECTION('',(-0.395324350758034,0.,-0.918541592796831));
#29155=DIRECTION('center_axis',(0.,1.,0.));
#29156=DIRECTION('ref_axis',(0.260729580930626,0.,0.965411873568862));
#29157=DIRECTION('',(0.287591132703736,0.,0.957753277410306));
#29158=DIRECTION('center_axis',(0.,1.,0.));
#29159=DIRECTION('ref_axis',(1.,0.,0.));
#29160=DIRECTION('',(-0.685643102443272,0.,-0.72793786552972));
#29161=DIRECTION('center_axis',(0.,1.,0.));
#29162=DIRECTION('ref_axis',(0.575195970587441,0.,0.818015644972621));
#29163=DIRECTION('',(0.597818178415659,0.,0.801631726889463));
#29164=DIRECTION('center_axis',(0.,1.,0.));
#29165=DIRECTION('ref_axis',(1.,0.,0.));
#29166=DIRECTION('',(-0.89326317695935,0.,-0.44953408846103));
#29167=DIRECTION('center_axis',(0.,1.,0.));
#29168=DIRECTION('ref_axis',(0.820285237202979,0.,0.571954656967538));
#29169=DIRECTION('',(0.835939528954005,0.,0.548821559281481));
#29170=DIRECTION('center_axis',(0.,1.,0.));
#29171=DIRECTION('ref_axis',(1.,0.,0.));
#29172=DIRECTION('',(-0.993142529173694,0.,-0.116909865907365));
#29173=DIRECTION('center_axis',(0.,1.,0.));
#29174=DIRECTION('ref_axis',(0.966435998091084,0.,0.256907496180414));
#29175=DIRECTION('',(0.973234235146997,0.,0.229815411880577));
#29176=DIRECTION('center_axis',(0.,1.,0.));
#29177=DIRECTION('ref_axis',(1.,0.,0.));
#29178=DIRECTION('',(-0.973234235146997,0.,0.229815411880577));
#29179=DIRECTION('center_axis',(0.,1.,0.));
#29180=DIRECTION('ref_axis',(0.996020314533121,0.,-0.0891265001968739));
#29181=DIRECTION('',(0.993142529173694,0.,-0.116909865907364));
#29182=DIRECTION('center_axis',(0.,1.,0.));
#29183=DIRECTION('ref_axis',(1.,0.,0.));
#29184=DIRECTION('',(-0.835939528953991,0.,0.548821559281502));
#29185=DIRECTION('center_axis',(0.,1.,0.));
#29186=DIRECTION('ref_axis',(0.9054698813482,0.,-0.424410525283336));
#29187=DIRECTION('',(0.893263176959351,0.,-0.449534088461028));
#29188=DIRECTION('center_axis',(0.,1.,0.));
#29189=DIRECTION('ref_axis',(1.,0.,0.));
#29190=DIRECTION('',(-0.597818178415657,0.,0.801631726889465));
#29191=DIRECTION('center_axis',(0.,1.,0.));
#29192=DIRECTION('ref_axis',(0.705706417160429,0.,-0.708504377388447));
#29193=DIRECTION('',(0.68564310244327,0.,-0.727937865529722));
#29194=DIRECTION('center_axis',(0.,1.,0.));
#29195=DIRECTION('ref_axis',(1.,0.,0.));
#29196=DIRECTION('',(-0.287591132703732,0.,0.957753277410307));
#29197=DIRECTION('center_axis',(0.,1.,0.));
#29198=DIRECTION('ref_axis',(0.420824343945678,0.,-0.907142145169482));
#29199=DIRECTION('',(0.395324350758034,0.,-0.918541592796831));
#29200=DIRECTION('center_axis',(0.,1.,0.));
#29201=DIRECTION('ref_axis',(1.,0.,0.));
#29202=DIRECTION('',(0.0573236480053483,0.,0.998355647742506));
#29203=DIRECTION('center_axis',(0.,1.,0.));
#29204=DIRECTION('ref_axis',(0.0851846441452059,0.,-0.996365182250893));
#29205=DIRECTION('',(0.0573236480053483,0.,-0.998355647742506));
#29206=DIRECTION('center_axis',(0.,1.,0.));
#29207=DIRECTION('ref_axis',(1.,0.,0.));
#29208=DIRECTION('',(0.395324350758037,0.,0.918541592796829));
#29209=DIRECTION('center_axis',(0.,1.,0.));
#29210=DIRECTION('ref_axis',(-0.260729580930624,0.,-0.965411873568862));
#29211=DIRECTION('',(-0.287591132703732,0.,-0.957753277410307));
#29212=DIRECTION('center_axis',(0.,1.,0.));
#29213=DIRECTION('ref_axis',(1.,0.,0.));
#29214=DIRECTION('',(0.685643102443273,0.,0.727937865529719));
#29215=DIRECTION('center_axis',(0.,1.,0.));
#29216=DIRECTION('ref_axis',(-0.575195970587437,0.,-0.818015644972623));
#29217=DIRECTION('',(-0.597818178415661,0.,-0.801631726889462));
#29218=DIRECTION('center_axis',(0.,1.,0.));
#29219=DIRECTION('ref_axis',(1.,0.,0.));
#29220=DIRECTION('',(0.89326317695935,0.,0.449534088461031));
#29221=DIRECTION('center_axis',(0.,1.,0.));
#29222=DIRECTION('ref_axis',(-0.820285237202974,0.,-0.571954656967543));
#29223=DIRECTION('',(-0.835939528954007,0.,-0.548821559281478));
#29224=DIRECTION('center_axis',(0.,1.,0.));
#29225=DIRECTION('ref_axis',(1.,0.,0.));
#29226=DIRECTION('',(0.993142529173694,0.,0.116909865907365));
#29227=DIRECTION('center_axis',(0.,1.,0.));
#29228=DIRECTION('ref_axis',(-0.966435998091082,0.,-0.256907496180421));
#29229=DIRECTION('',(-0.973234235146997,0.,-0.229815411880577));
#29230=DIRECTION('center_axis',(0.,1.,0.));
#29231=DIRECTION('ref_axis',(1.,0.,0.));
#29232=DIRECTION('center_axis',(0.,-1.,0.));
#29233=DIRECTION('ref_axis',(1.,0.,0.));
#29234=DIRECTION('',(0.,1.,0.));
#29235=DIRECTION('center_axis',(0.,-1.,0.));
#29236=DIRECTION('ref_axis',(1.,0.,0.));
#29237=DIRECTION('center_axis',(0.,1.,0.));
#29238=DIRECTION('ref_axis',(0.,0.,1.));
#29239=DIRECTION('center_axis',(0.,-1.,0.));
#29240=DIRECTION('ref_axis',(1.,0.,0.));
#29241=DIRECTION('center_axis',(0.,-1.,0.));
#29242=DIRECTION('ref_axis',(1.,0.,0.));
#29243=DIRECTION('center_axis',(0.,-1.,0.));
#29244=DIRECTION('ref_axis',(1.,0.,0.));
#29245=DIRECTION('',(0.707106781186541,0.707106781186554,8.65956056235486E-17));
#29246=DIRECTION('center_axis',(0.,-1.,0.));
#29247=DIRECTION('ref_axis',(1.,0.,0.));
#29248=DIRECTION('center_axis',(0.,-1.,0.));
#29249=DIRECTION('ref_axis',(1.,0.,0.));
#29250=DIRECTION('',(0.,1.,0.));
#29251=DIRECTION('center_axis',(0.,1.,0.));
#29252=DIRECTION('ref_axis',(0.,0.,1.));
#29253=DIRECTION('center_axis',(0.,-1.,0.));
#29254=DIRECTION('ref_axis',(1.,0.,0.));
#29255=DIRECTION('center_axis',(0.,-1.,0.));
#29256=DIRECTION('ref_axis',(1.,0.,0.));
#29257=DIRECTION('',(0.707106781186543,0.707106781186552,8.65956056235488E-17));
#29258=DIRECTION('center_axis',(0.,1.,0.));
#29259=DIRECTION('ref_axis',(1.,0.,0.));
#29260=DIRECTION('center_axis',(0.,-1.,0.));
#29261=DIRECTION('ref_axis',(1.,0.,0.));
#29262=DIRECTION('',(-0.707106781186543,0.707106781186552,-8.65956056235488E-17));
#29263=DIRECTION('center_axis',(0.,-1.,0.));
#29264=DIRECTION('ref_axis',(0.,0.,-1.));
#29265=DIRECTION('center_axis',(0.,-1.,0.));
#29266=DIRECTION('ref_axis',(1.,0.,0.));
#29267=DIRECTION('center_axis',(0.,-1.,0.));
#29268=DIRECTION('ref_axis',(1.,0.,0.));
#29269=DIRECTION('center_axis',(0.,-1.,0.));
#29270=DIRECTION('ref_axis',(1.,0.,0.));
#29271=DIRECTION('',(0.,1.,0.));
#29272=DIRECTION('center_axis',(0.,1.,0.));
#29273=DIRECTION('ref_axis',(1.,0.,0.));
#29274=DIRECTION('center_axis',(0.,-1.,0.));
#29275=DIRECTION('ref_axis',(1.,0.,0.));
#29276=DIRECTION('',(-0.707106781186541,0.707106781186554,-8.65956056235486E-17));
#29277=DIRECTION('center_axis',(0.,-1.,0.));
#29278=DIRECTION('ref_axis',(0.,0.,-1.));
#29279=DIRECTION('',(0.,1.,0.));
#29280=DIRECTION('center_axis',(0.,1.,0.));
#29281=DIRECTION('ref_axis',(-0.905469881348196,0.,0.424410525283343));
#29282=DIRECTION('',(0.,-1.,0.));
#29283=DIRECTION('',(0.,1.,0.));
#29284=DIRECTION('center_axis',(0.44953408846103,0.,0.89326317695935));
#29285=DIRECTION('ref_axis',(0.89326317695935,0.,-0.44953408846103));
#29286=DIRECTION('',(0.,1.,0.));
#29287=DIRECTION('center_axis',(-0.548821559281503,0.,-0.835939528953991));
#29288=DIRECTION('ref_axis',(-0.835939528953991,0.,0.548821559281503));
#29289=DIRECTION('',(0.,1.,0.));
#29290=DIRECTION('center_axis',(0.,1.,0.));
#29291=DIRECTION('ref_axis',(-0.420824343945662,0.,0.907142145169489));
#29292=DIRECTION('',(0.,-1.,0.));
#29293=DIRECTION('',(0.,1.,0.));
#29294=DIRECTION('center_axis',(0.918541592796826,0.,0.395324350758046));
#29295=DIRECTION('ref_axis',(0.395324350758046,0.,-0.918541592796826));
#29296=DIRECTION('',(0.,1.,0.));
#29297=DIRECTION('center_axis',(-0.957753277410307,0.,-0.287591132703732));
#29298=DIRECTION('ref_axis',(-0.287591132703732,0.,0.957753277410307));
#29299=DIRECTION('',(0.,1.,0.));
#29300=DIRECTION('center_axis',(0.,1.,0.));
#29301=DIRECTION('ref_axis',(0.260729580930626,0.,0.965411873568862));
#29302=DIRECTION('',(0.,-1.,0.));
#29303=DIRECTION('',(0.,1.,0.));
#29304=DIRECTION('center_axis',(0.957753277410306,0.,-0.287591132703736));
#29305=DIRECTION('ref_axis',(-0.287591132703736,0.,-0.957753277410306));
#29306=DIRECTION('',(0.,1.,0.));
#29307=DIRECTION('center_axis',(-0.918541592796831,0.,0.395324350758034));
#29308=DIRECTION('ref_axis',(0.395324350758034,0.,0.918541592796831));
#29309=DIRECTION('',(0.,1.,0.));
#29310=DIRECTION('center_axis',(0.,1.,0.));
#29311=DIRECTION('ref_axis',(0.820285237202979,0.,0.571954656967538));
#29312=DIRECTION('',(0.,-1.,0.));
#29313=DIRECTION('',(0.,1.,0.));
#29314=DIRECTION('center_axis',(0.548821559281481,0.,-0.835939528954005));
#29315=DIRECTION('ref_axis',(-0.835939528954005,0.,-0.548821559281481));
#29316=DIRECTION('',(0.,1.,0.));
#29317=DIRECTION('center_axis',(-0.44953408846103,0.,0.89326317695935));
#29318=DIRECTION('ref_axis',(0.89326317695935,0.,0.44953408846103));
#29319=DIRECTION('',(0.,1.,0.));
#29320=DIRECTION('center_axis',(0.,1.,0.));
#29321=DIRECTION('ref_axis',(-0.966435998091082,0.,-0.256907496180421));
#29322=DIRECTION('',(0.,-1.,0.));
#29323=DIRECTION('',(0.,1.,0.));
#29324=DIRECTION('center_axis',(-0.229815411880577,0.,0.973234235146997));
#29325=DIRECTION('ref_axis',(0.973234235146997,0.,0.229815411880577));
#29326=DIRECTION('',(0.,1.,0.));
#29327=DIRECTION('center_axis',(0.116909865907365,0.,-0.993142529173694));
#29328=DIRECTION('ref_axis',(-0.993142529173694,0.,-0.116909865907365));
#29329=DIRECTION('',(0.,1.,0.));
#29330=DIRECTION('center_axis',(0.,1.,0.));
#29331=DIRECTION('ref_axis',(0.9054698813482,0.,-0.424410525283336));
#29332=DIRECTION('',(0.,-1.,0.));
#29333=DIRECTION('',(0.,1.,0.));
#29334=DIRECTION('center_axis',(-0.449534088461028,0.,-0.893263176959351));
#29335=DIRECTION('ref_axis',(-0.893263176959351,0.,0.449534088461028));
#29336=DIRECTION('',(0.,1.,0.));
#29337=DIRECTION('center_axis',(0.548821559281502,0.,0.835939528953991));
#29338=DIRECTION('ref_axis',(0.835939528953991,0.,-0.548821559281502));
#29339=DIRECTION('',(0.,1.,0.));
#29340=DIRECTION('center_axis',(0.,1.,0.));
#29341=DIRECTION('ref_axis',(0.420824343945678,0.,-0.907142145169482));
#29342=DIRECTION('',(0.,-1.,0.));
#29343=DIRECTION('',(0.,1.,0.));
#29344=DIRECTION('center_axis',(-0.918541592796831,0.,-0.395324350758034));
#29345=DIRECTION('ref_axis',(-0.395324350758034,0.,0.918541592796831));
#29346=DIRECTION('',(0.,1.,0.));
#29347=DIRECTION('center_axis',(0.957753277410307,0.,0.287591132703732));
#29348=DIRECTION('ref_axis',(0.287591132703732,0.,-0.957753277410307));
#29349=DIRECTION('',(0.,1.,0.));
#29350=DIRECTION('center_axis',(0.,1.,0.));
#29351=DIRECTION('ref_axis',(-0.260729580930624,0.,-0.965411873568862));
#29352=DIRECTION('',(0.,-1.,0.));
#29353=DIRECTION('',(0.,1.,0.));
#29354=DIRECTION('center_axis',(-0.957753277410307,0.,0.287591132703732));
#29355=DIRECTION('ref_axis',(0.287591132703732,0.,0.957753277410307));
#29356=DIRECTION('',(0.,1.,0.));
#29357=DIRECTION('center_axis',(0.918541592796829,0.,-0.395324350758037));
#29358=DIRECTION('ref_axis',(-0.395324350758037,0.,-0.918541592796829));
#29359=DIRECTION('',(0.,1.,0.));
#29360=DIRECTION('center_axis',(0.,1.,0.));
#29361=DIRECTION('ref_axis',(-0.820285237202974,0.,-0.571954656967543));
#29362=DIRECTION('',(0.,-1.,0.));
#29363=DIRECTION('',(0.,1.,0.));
#29364=DIRECTION('center_axis',(-0.548821559281478,0.,0.835939528954007));
#29365=DIRECTION('ref_axis',(0.835939528954007,0.,0.548821559281478));
#29366=DIRECTION('',(0.,1.,0.));
#29367=DIRECTION('center_axis',(0.449534088461031,0.,-0.89326317695935));
#29368=DIRECTION('ref_axis',(-0.89326317695935,0.,-0.449534088461031));
#29369=DIRECTION('',(0.,1.,0.));
#29370=DIRECTION('center_axis',(0.,1.,0.));
#29371=DIRECTION('ref_axis',(-0.575195970587437,0.,-0.818015644972623));
#29372=DIRECTION('',(0.,-1.,0.));
#29373=DIRECTION('',(0.,1.,0.));
#29374=DIRECTION('center_axis',(-0.801631726889462,0.,0.597818178415661));
#29375=DIRECTION('ref_axis',(0.597818178415661,0.,0.801631726889462));
#29376=DIRECTION('',(0.,1.,0.));
#29377=DIRECTION('center_axis',(0.727937865529719,0.,-0.685643102443273));
#29378=DIRECTION('ref_axis',(-0.685643102443273,0.,-0.727937865529719));
#29379=DIRECTION('',(0.,1.,0.));
#29380=DIRECTION('center_axis',(0.,1.,0.));
#29381=DIRECTION('ref_axis',(0.0851846441452059,0.,-0.996365182250893));
#29382=DIRECTION('',(0.,-1.,0.));
#29383=DIRECTION('',(0.,1.,0.));
#29384=DIRECTION('center_axis',(-0.998355647742506,0.,-0.0573236480053483));
#29385=DIRECTION('ref_axis',(-0.0573236480053483,0.,0.998355647742506));
#29386=DIRECTION('',(0.,1.,0.));
#29387=DIRECTION('center_axis',(0.998355647742506,0.,-0.0573236480053483));
#29388=DIRECTION('ref_axis',(-0.0573236480053483,0.,-0.998355647742506));
#29389=DIRECTION('',(0.,1.,0.));
#29390=DIRECTION('center_axis',(0.,1.,0.));
#29391=DIRECTION('ref_axis',(0.705706417160429,0.,-0.708504377388447));
#29392=DIRECTION('',(0.,-1.,0.));
#29393=DIRECTION('',(0.,1.,0.));
#29394=DIRECTION('center_axis',(-0.727937865529722,0.,-0.68564310244327));
#29395=DIRECTION('ref_axis',(-0.68564310244327,0.,0.727937865529722));
#29396=DIRECTION('',(0.,1.,0.));
#29397=DIRECTION('center_axis',(0.801631726889465,0.,0.597818178415657));
#29398=DIRECTION('ref_axis',(0.597818178415657,0.,-0.801631726889465));
#29399=DIRECTION('',(0.,1.,0.));
#29400=DIRECTION('center_axis',(0.,1.,0.));
#29401=DIRECTION('ref_axis',(0.996020314533121,0.,-0.0891265001968739));
#29402=DIRECTION('',(0.,-1.,0.));
#29403=DIRECTION('',(0.,1.,0.));
#29404=DIRECTION('center_axis',(-0.116909865907364,0.,-0.993142529173694));
#29405=DIRECTION('ref_axis',(-0.993142529173694,0.,0.116909865907364));
#29406=DIRECTION('',(0.,1.,0.));
#29407=DIRECTION('center_axis',(0.229815411880577,0.,0.973234235146997));
#29408=DIRECTION('ref_axis',(0.973234235146997,0.,-0.229815411880577));
#29409=DIRECTION('',(0.,1.,0.));
#29410=DIRECTION('center_axis',(0.,1.,0.));
#29411=DIRECTION('ref_axis',(0.966435998091084,0.,0.256907496180414));
#29412=DIRECTION('',(0.,-1.,0.));
#29413=DIRECTION('',(0.,1.,0.));
#29414=DIRECTION('center_axis',(0.229815411880577,0.,-0.973234235146997));
#29415=DIRECTION('ref_axis',(-0.973234235146997,0.,-0.229815411880577));
#29416=DIRECTION('',(0.,1.,0.));
#29417=DIRECTION('center_axis',(-0.116909865907365,0.,0.993142529173694));
#29418=DIRECTION('ref_axis',(0.993142529173694,0.,0.116909865907365));
#29419=DIRECTION('',(0.,1.,0.));
#29420=DIRECTION('center_axis',(0.,1.,0.));
#29421=DIRECTION('ref_axis',(0.575195970587441,0.,0.818015644972621));
#29422=DIRECTION('',(0.,-1.,0.));
#29423=DIRECTION('',(0.,1.,0.));
#29424=DIRECTION('center_axis',(0.801631726889463,0.,-0.597818178415659));
#29425=DIRECTION('ref_axis',(-0.597818178415659,0.,-0.801631726889463));
#29426=DIRECTION('',(0.,1.,0.));
#29427=DIRECTION('center_axis',(-0.72793786552972,0.,0.685643102443272));
#29428=DIRECTION('ref_axis',(0.685643102443272,0.,0.72793786552972));
#29429=DIRECTION('',(0.,1.,0.));
#29430=DIRECTION('center_axis',(0.,1.,0.));
#29431=DIRECTION('ref_axis',(-0.0851846441452059,0.,0.996365182250893));
#29432=DIRECTION('',(0.,-1.,0.));
#29433=DIRECTION('',(0.,1.,0.));
#29434=DIRECTION('center_axis',(0.998355647742506,0.,0.0573236480053483));
#29435=DIRECTION('ref_axis',(0.0573236480053483,0.,-0.998355647742506));
#29436=DIRECTION('',(0.,1.,0.));
#29437=DIRECTION('center_axis',(-0.998355647742506,0.,0.0573236480053525));
#29438=DIRECTION('ref_axis',(0.0573236480053525,0.,0.998355647742506));
#29439=DIRECTION('',(0.,1.,0.));
#29440=DIRECTION('center_axis',(0.,1.,0.));
#29441=DIRECTION('ref_axis',(-0.705706417160429,0.,0.708504377388447));
#29442=DIRECTION('',(0.,-1.,0.));
#29443=DIRECTION('',(0.,1.,0.));
#29444=DIRECTION('center_axis',(0.727937865529721,0.,0.685643102443271));
#29445=DIRECTION('ref_axis',(0.685643102443271,0.,-0.727937865529721));
#29446=DIRECTION('',(0.,1.,0.));
#29447=DIRECTION('center_axis',(-0.801631726889465,0.,-0.597818178415657));
#29448=DIRECTION('ref_axis',(-0.597818178415657,0.,0.801631726889465));
#29449=DIRECTION('',(0.,1.,0.));
#29450=DIRECTION('center_axis',(0.,1.,0.));
#29451=DIRECTION('ref_axis',(-0.996020314533121,0.,0.0891265001968672));
#29452=DIRECTION('',(0.,-1.,0.));
#29453=DIRECTION('',(0.,1.,0.));
#29454=DIRECTION('center_axis',(0.116909865907365,0.,0.993142529173694));
#29455=DIRECTION('ref_axis',(0.993142529173694,0.,-0.116909865907365));
#29456=DIRECTION('',(0.,1.,0.));
#29457=DIRECTION('center_axis',(-0.229815411880577,0.,-0.973234235146997));
#29458=DIRECTION('ref_axis',(-0.973234235146997,0.,0.229815411880577));
#29459=DIRECTION('center_axis',(0.,1.,0.));
#29460=DIRECTION('ref_axis',(1.,0.,0.));
#29461=DIRECTION('center_axis',(0.,1.,0.));
#29462=DIRECTION('ref_axis',(1.,0.,0.));
#29463=DIRECTION('center_axis',(0.,1.,0.));
#29464=DIRECTION('ref_axis',(1.,0.,0.));
#29465=DIRECTION('center_axis',(0.,1.,0.));
#29466=DIRECTION('ref_axis',(1.,0.,0.));
#29467=DIRECTION('center_axis',(0.,1.,0.));
#29468=DIRECTION('ref_axis',(1.,0.,0.));
#29469=DIRECTION('center_axis',(0.,1.,0.));
#29470=DIRECTION('ref_axis',(1.,0.,0.));
#29471=DIRECTION('center_axis',(0.,1.,0.));
#29472=DIRECTION('ref_axis',(1.,0.,0.));
#29473=DIRECTION('center_axis',(0.,1.,0.));
#29474=DIRECTION('ref_axis',(1.,0.,0.));
#29475=DIRECTION('center_axis',(0.,1.,0.));
#29476=DIRECTION('ref_axis',(1.,0.,0.));
#29477=DIRECTION('center_axis',(0.,1.,0.));
#29478=DIRECTION('ref_axis',(-1.,0.,-2.5785718345414E-11));
#29479=DIRECTION('center_axis',(0.,1.,0.));
#29480=DIRECTION('ref_axis',(1.,0.,0.));
#29481=DIRECTION('center_axis',(0.,1.,0.));
#29482=DIRECTION('ref_axis',(1.,0.,0.));
#29483=DIRECTION('center_axis',(0.,1.,0.));
#29484=DIRECTION('ref_axis',(1.,0.,0.));
#29485=DIRECTION('center_axis',(0.,1.,0.));
#29486=DIRECTION('ref_axis',(1.,0.,0.));
#29487=DIRECTION('center_axis',(0.,1.,0.));
#29488=DIRECTION('ref_axis',(1.,0.,0.));
#29489=DIRECTION('center_axis',(0.,1.,0.));
#29490=DIRECTION('ref_axis',(1.,0.,0.));
#29491=DIRECTION('center_axis',(0.,1.,0.));
#29492=DIRECTION('ref_axis',(1.,0.,0.));
#29493=DIRECTION('center_axis',(0.,1.,0.));
#29494=DIRECTION('ref_axis',(1.,0.,0.));
#35347=CARTESIAN_POINT('',(0.,0.,0.));
#35348=CARTESIAN_POINT('Origin',(9.31,-4.875,78.));
#35349=CARTESIAN_POINT('',(15.56,-4.95,78.));
#35350=CARTESIAN_POINT('',(3.06,-4.95,78.));
#35351=CARTESIAN_POINT('Origin',(9.31,-4.95,78.));
#35352=CARTESIAN_POINT('Origin',(9.31,-4.95,78.));
#35353=CARTESIAN_POINT('',(15.41,-4.8,78.));
#35354=CARTESIAN_POINT('',(15.485,-4.875,78.));
#35355=CARTESIAN_POINT('Origin',(9.31,-4.8,78.));
#35356=CARTESIAN_POINT('Origin',(15.56,-4.8,78.));
#35357=CARTESIAN_POINT('',(4.2616449875437,-4.8,78.5128739112901));
#35358=CARTESIAN_POINT('',(3.31329278848646,-4.8,78.1987526588035));
#35359=CARTESIAN_POINT('Ctrl Pts',(4.2616449875437,-4.8,78.5128739112901));
#35360=CARTESIAN_POINT('Ctrl Pts',(4.21748868989439,-4.8,78.5162020803145));
#35361=CARTESIAN_POINT('Ctrl Pts',(4.15767750006772,-4.8,78.5102954843629));
#35362=CARTESIAN_POINT('Ctrl Pts',(3.96449151342978,-4.8,78.4820870104176));
#35363=CARTESIAN_POINT('Ctrl Pts',(3.82580660796765,-4.8,78.4380535018334));
#35364=CARTESIAN_POINT('Ctrl Pts',(3.56890774120608,-4.8,78.3375379190907));
#35365=CARTESIAN_POINT('Ctrl Pts',(3.43851411968528,-4.8,78.2720997066612));
#35366=CARTESIAN_POINT('Ctrl Pts',(3.31329278848645,-4.8,78.1987526588035));
#35367=CARTESIAN_POINT('',(3.31329278849671,-4.8,77.8012473408872));
#35368=CARTESIAN_POINT('Origin',(9.31,-4.8,78.));
#35369=CARTESIAN_POINT('',(4.2616449875437,-4.8,77.4871260887099));
#35370=CARTESIAN_POINT('Ctrl Pts',(3.3132927884967,-4.8,77.8012473408872));
#35371=CARTESIAN_POINT('Ctrl Pts',(3.35889085631205,-4.8,77.774538763147));
#35372=CARTESIAN_POINT('Ctrl Pts',(3.40424018038843,-4.8,77.7494140892238));
#35373=CARTESIAN_POINT('Ctrl Pts',(3.44932023931853,-4.8,77.7259332918199));
#35374=CARTESIAN_POINT('Ctrl Pts',(3.48535154467789,-4.8,77.7071657080717));
#35375=CARTESIAN_POINT('Ctrl Pts',(3.52121323519527,-4.8,77.6894485799316));
#35376=CARTESIAN_POINT('Ctrl Pts',(3.55687519269613,-4.8,77.6727963528265));
#35377=CARTESIAN_POINT('Ctrl Pts',(3.58544218901406,-4.8,77.6594570931859));
#35378=CARTESIAN_POINT('Ctrl Pts',(3.61388191592754,-4.8,77.6468005097403));
#35379=CARTESIAN_POINT('Ctrl Pts',(3.64214093417943,-4.8,77.6348321699585));
#35380=CARTESIAN_POINT('Ctrl Pts',(3.67299487491485,-4.8,77.6217648212262));
#35381=CARTESIAN_POINT('Ctrl Pts',(3.70363431536384,-4.8,77.609517604295));
#35382=CARTESIAN_POINT('Ctrl Pts',(3.73391380774594,-4.8,77.5981023686591));
#35383=CARTESIAN_POINT('Ctrl Pts',(3.76023545579461,-4.8,77.5881792229534));
#35384=CARTESIAN_POINT('Ctrl Pts',(3.78627885577575,-4.8,77.5788849711814));
#35385=CARTESIAN_POINT('Ctrl Pts',(3.81195344757976,-4.8,77.5702305821903));
#35386=CARTESIAN_POINT('Ctrl Pts',(3.83288569746951,-4.8,77.5631747413657));
#35387=CARTESIAN_POINT('Ctrl Pts',(3.85357165256806,-4.8,77.5565443368315));
#35388=CARTESIAN_POINT('Ctrl Pts',(3.87400245730923,-4.8,77.5503456729673));
#35389=CARTESIAN_POINT('Ctrl Pts',(3.89634471953046,-4.8,77.5435670768605));
#35390=CARTESIAN_POINT('Ctrl Pts',(3.91838596197266,-4.8,77.5373047098573));
#35391=CARTESIAN_POINT('Ctrl Pts',(3.94016536091701,-4.8,77.5315664445101));
#35392=CARTESIAN_POINT('Ctrl Pts',(3.95632811812935,-4.8,77.5273080079084));
#35393=CARTESIAN_POINT('Ctrl Pts',(3.97234882666259,-4.8,77.5233381875081));
#35394=CARTESIAN_POINT('Ctrl Pts',(3.98822206424162,-4.8,77.5196608232975));
#35395=CARTESIAN_POINT('Ctrl Pts',(4.0027286437008,-4.8,77.5163000737431));
#35396=CARTESIAN_POINT('Ctrl Pts',(4.01711313080281,-4.8,77.5131835791406));
#35397=CARTESIAN_POINT('Ctrl Pts',(4.03133253269136,-4.8,77.5103150376875));
#35398=CARTESIAN_POINT('Ctrl Pts',(4.04574667531631,-4.8,77.5074072103433));
#35399=CARTESIAN_POINT('Ctrl Pts',(4.05999158764115,-4.8,77.50475418481));
#35400=CARTESIAN_POINT('Ctrl Pts',(4.073966587985,-4.8,77.5023606915013));
#35401=CARTESIAN_POINT('Ctrl Pts',(4.09342501070055,-4.8,77.499028054405));
#35402=CARTESIAN_POINT('Ctrl Pts',(4.11235622185552,-4.8,77.4961988311417));
#35403=CARTESIAN_POINT('Ctrl Pts',(4.130391951486,-4.8,77.4938857626853));
#35404=CARTESIAN_POINT('Ctrl Pts',(4.14391874870886,-4.8,77.492150961343));
#35405=CARTESIAN_POINT('Ctrl Pts',(4.15693803977231,-4.8,77.4907065511493));
#35406=CARTESIAN_POINT('Ctrl Pts',(4.16931232039428,-4.8,77.4895559928397));
#35407=CARTESIAN_POINT('Ctrl Pts',(4.1812650340981,-4.8,77.4884446317437));
#35408=CARTESIAN_POINT('Ctrl Pts',(4.19261487926314,-4.8,77.48760745091));
#35409=CARTESIAN_POINT('Ctrl Pts',(4.20329220748563,-4.8,77.4870447436042));
#35410=CARTESIAN_POINT('Ctrl Pts',(4.21554028423639,-4.8,77.4863992560696));
#35411=CARTESIAN_POINT('Ctrl Pts',(4.22690460313112,-4.8,77.4861147687392));
#35412=CARTESIAN_POINT('Ctrl Pts',(4.23735441716533,-4.8,77.48618908429));
#35413=CARTESIAN_POINT('Ctrl Pts',(4.24608785219741,-4.8,77.4862511935327));
#35414=CARTESIAN_POINT('Ctrl Pts',(4.25418482587244,-4.8,77.4865637978906));
#35415=CARTESIAN_POINT('Ctrl Pts',(4.2616449875437,-4.8,77.4871260887099));
#35416=CARTESIAN_POINT('',(4.67850553742098,-4.8,77.5855617740846));
#35417=CARTESIAN_POINT('',(6.70986352030667,-4.8,78.0652380479502));
#35418=CARTESIAN_POINT('',(4.81607260887647,-4.8,76.805380142761));
#35419=CARTESIAN_POINT('Origin',(9.3100000000004,-4.8,78.0000000000001));
#35420=CARTESIAN_POINT('',(4.39068483903982,-4.8,76.7553047249138));
#35421=CARTESIAN_POINT('',(7.10167754842447,-4.8,77.0744349452193));
#35422=CARTESIAN_POINT('',(3.60696107145242,-4.8,76.1357717469497));
#35423=CARTESIAN_POINT('Ctrl Pts',(4.39068483903982,-4.8,76.7553047249138));
#35424=CARTESIAN_POINT('Ctrl Pts',(4.34805318890719,-4.8,76.743329836952));
#35425=CARTESIAN_POINT('Ctrl Pts',(4.29386922796023,-4.8,76.7173228188007));
#35426=CARTESIAN_POINT('Ctrl Pts',(4.12525248244484,-4.8,76.6265037376292));
#35427=CARTESIAN_POINT('Ctrl Pts',(4.00650765748837,-4.8,76.5376601133753));
#35428=CARTESIAN_POINT('Ctrl Pts',(3.79828001734992,-4.8,76.3505159793066));
#35429=CARTESIAN_POINT('Ctrl Pts',(3.70426215481285,-4.8,76.2532180870415));
#35430=CARTESIAN_POINT('Ctrl Pts',(3.60696107145241,-4.8,76.1357717469497));
#35431=CARTESIAN_POINT('',(3.74291589727828,-4.8,75.7622389329459));
#35432=CARTESIAN_POINT('Origin',(9.31,-4.8,78.));
#35433=CARTESIAN_POINT('',(4.7415112563347,-4.8,75.7914170652479));
#35434=CARTESIAN_POINT('Ctrl Pts',(3.74291589727827,-4.8,75.7622389329459));
#35435=CARTESIAN_POINT('Ctrl Pts',(3.79489893671569,-4.8,75.752736537219));
#35436=CARTESIAN_POINT('Ctrl Pts',(3.8461065065151,-4.8,75.7446374488288));
#35437=CARTESIAN_POINT('Ctrl Pts',(3.89649881094588,-4.8,75.7379910049808));
#35438=CARTESIAN_POINT('Ctrl Pts',(3.93677605596246,-4.8,75.7326786770295));
#35439=CARTESIAN_POINT('Ctrl Pts',(3.97653463813689,-4.8,75.7282954428482));
#35440=CARTESIAN_POINT('Ctrl Pts',(4.0157413150127,-4.8,75.7248445756745));
#35441=CARTESIAN_POINT('Ctrl Pts',(4.04714780575629,-4.8,75.7220802600889));
#35442=CARTESIAN_POINT('Ctrl Pts',(4.0782012133719,-4.8,75.7199139215761));
#35443=CARTESIAN_POINT('Ctrl Pts',(4.1088494172024,-4.8,75.7183325145388));
#35444=CARTESIAN_POINT('Ctrl Pts',(4.14231193316861,-4.8,75.7166058926941));
#35445=CARTESIAN_POINT('Ctrl Pts',(4.17529238322651,-4.8,75.7155765791924));
#35446=CARTESIAN_POINT('Ctrl Pts',(4.20765003841591,-4.8,75.7152059628458));
#35447=CARTESIAN_POINT('Ctrl Pts',(4.23577821253443,-4.8,75.7148837898989));
#35448=CARTESIAN_POINT('Ctrl Pts',(4.26342982460602,-4.8,75.7150574174935));
#35449=CARTESIAN_POINT('Ctrl Pts',(4.29051602439583,-4.8,75.7157061795936));
#35450=CARTESIAN_POINT('Ctrl Pts',(4.31259914472419,-4.8,75.7162351091457));
#35451=CARTESIAN_POINT('Ctrl Pts',(4.33430531587732,-4.8,75.7170795802567));
#35452=CARTESIAN_POINT('Ctrl Pts',(4.3556240601199,-4.8,75.7182424883248));
#35453=CARTESIAN_POINT('Ctrl Pts',(4.37893733544232,-4.8,75.7195141953099));
#35454=CARTESIAN_POINT('Ctrl Pts',(4.40179118394796,-4.8,75.7211680441458));
#35455=CARTESIAN_POINT('Ctrl Pts',(4.42421972672823,-4.8,75.7232248316902));
#35456=CARTESIAN_POINT('Ctrl Pts',(4.44086422150209,-4.8,75.7247511987782));
#35457=CARTESIAN_POINT('Ctrl Pts',(4.45727652162596,-4.8,75.7265001928719));
#35458=CARTESIAN_POINT('Ctrl Pts',(4.47345021847494,-4.8,75.7284735678523));
#35459=CARTESIAN_POINT('Ctrl Pts',(4.48823138815577,-4.8,75.7302770386792));
#35460=CARTESIAN_POINT('Ctrl Pts',(4.502814288437,-4.8,75.732268276036));
#35461=CARTESIAN_POINT('Ctrl Pts',(4.51715725439111,-4.8,75.7344360506685));
#35462=CARTESIAN_POINT('Ctrl Pts',(4.53169665335291,-4.8,75.7366335138949));
#35463=CARTESIAN_POINT('Ctrl Pts',(4.54598988049976,-4.8,75.7390125323308));
#35464=CARTESIAN_POINT('Ctrl Pts',(4.5599407081024,-4.8,75.7415431159479));
#35465=CARTESIAN_POINT('Ctrl Pts',(4.57936547336537,-4.8,75.7450666339885));
#35466=CARTESIAN_POINT('Ctrl Pts',(4.59812264414369,-4.8,75.7488828893195));
#35467=CARTESIAN_POINT('Ctrl Pts',(4.61586180219855,-4.8,75.752877898793));
#35468=CARTESIAN_POINT('Ctrl Pts',(4.62916617073969,-4.8,75.7558741558981));
#35469=CARTESIAN_POINT('Ctrl Pts',(4.64189431986447,-4.8,75.7589697140927));
#35470=CARTESIAN_POINT('Ctrl Pts',(4.65391585417251,-4.8,75.7621207961701));
#35471=CARTESIAN_POINT('Ctrl Pts',(4.66552783887808,-4.8,75.7651645271907));
#35472=CARTESIAN_POINT('Ctrl Pts',(4.67647953729782,-4.8,75.7682597101957));
#35473=CARTESIAN_POINT('Ctrl Pts',(4.68670540103973,-4.8,75.7713827996084));
#35474=CARTESIAN_POINT('Ctrl Pts',(4.69843559818659,-4.8,75.7749653287174));
#35475=CARTESIAN_POINT('Ctrl Pts',(4.70921186524681,-4.8,75.7785848240668));
#35476=CARTESIAN_POINT('Ctrl Pts',(4.71900606101744,-4.8,75.7822287047553));
#35477=CARTESIAN_POINT('Ctrl Pts',(4.72719156284253,-4.8,75.7852740790489));
#35478=CARTESIAN_POINT('Ctrl Pts',(4.7346933122562,-4.8,75.788337159151));
#35479=CARTESIAN_POINT('Ctrl Pts',(4.7415112563347,-4.8,75.7914170652479));
#35480=CARTESIAN_POINT('',(5.09956505173093,-4.8,76.0264910574324));
#35481=CARTESIAN_POINT('',(6.84435821048571,-4.8,77.1720046608023));
#35482=CARTESIAN_POINT('',(5.49567364700612,-4.8,75.340410845101));
#35483=CARTESIAN_POINT('Origin',(9.30999999999911,-4.8,77.9999999999995));
#35484=CARTESIAN_POINT('',(5.11306670030725,-4.8,75.1478641584586));
#35485=CARTESIAN_POINT('',(7.55141758063195,-4.8,76.3749625865681));
#35486=CARTESIAN_POINT('',(4.58850001706627,-4.8,74.2976442754434));
#35487=CARTESIAN_POINT('Ctrl Pts',(5.11306670030725,-4.8,75.1478641584586));
#35488=CARTESIAN_POINT('Ctrl Pts',(5.07710170456016,-4.8,75.122030560416));
#35489=CARTESIAN_POINT('Ctrl Pts',(5.03508035930635,-4.8,75.0790599492463));
#35490=CARTESIAN_POINT('Ctrl Pts',(4.9076944069207,-4.8,74.9360476103334));
#35491=CARTESIAN_POINT('Ctrl Pts',(4.82649707995744,-4.8,74.8119487900272));
#35492=CARTESIAN_POINT('Ctrl Pts',(4.69483416636455,-4.8,74.5648727807342));
#35493=CARTESIAN_POINT('Ctrl Pts',(4.63976411326715,-4.8,74.4412866656976));
#35494=CARTESIAN_POINT('Ctrl Pts',(4.58850001706627,-4.8,74.2976442754434));
#35495=CARTESIAN_POINT('',(4.84401151027683,-4.8,73.9931375354699));
#35496=CARTESIAN_POINT('Origin',(9.31,-4.8,78.));
#35497=CARTESIAN_POINT('',(5.77240469132477,-4.8,74.3620957389297));
#35498=CARTESIAN_POINT('Ctrl Pts',(4.84401151027683,-4.8,73.9931375354699));
#35499=CARTESIAN_POINT('Ctrl Pts',(5.02013219956813,-4.8,74.0230552009928));
#35500=CARTESIAN_POINT('Ctrl Pts',(5.19307522703524,-4.8,74.0670863794806));
#35501=CARTESIAN_POINT('Ctrl Pts',(5.45666781109844,-4.8,74.1681448115599));
#35502=CARTESIAN_POINT('Ctrl Pts',(5.53752890906739,-4.8,74.2065364265515));
#35503=CARTESIAN_POINT('Ctrl Pts',(5.67001324763651,-4.8,74.2823453026591));
#35504=CARTESIAN_POINT('Ctrl Pts',(5.735048362443,-4.8,74.3256280169092));
#35505=CARTESIAN_POINT('Ctrl Pts',(5.77240469132477,-4.8,74.3620957389297));
#35506=CARTESIAN_POINT('',(6.02846516020394,-4.8,74.7054546451438));
#35507=CARTESIAN_POINT('',(7.27624568947745,-4.8,76.3786397314713));
#35508=CARTESIAN_POINT('',(6.63533873676838,-4.8,74.1962272508773));
#35509=CARTESIAN_POINT('Origin',(9.30999999999964,-4.8,77.9999999999996));
#35510=CARTESIAN_POINT('',(6.34166065765632,-4.8,73.8844332675354));
#35511=CARTESIAN_POINT('',(8.21326860652757,-4.8,75.8714937229748));
#35512=CARTESIAN_POINT('',(6.13952154251132,-4.8,72.9060755452598));
#35513=CARTESIAN_POINT('Ctrl Pts',(6.34166065765632,-4.8,73.8844332675354));
#35514=CARTESIAN_POINT('Ctrl Pts',(6.31670022667317,-4.8,73.8478568720211));
#35515=CARTESIAN_POINT('Ctrl Pts',(6.29190989306677,-4.8,73.7931055577262));
#35516=CARTESIAN_POINT('Ctrl Pts',(6.22111935580918,-4.8,73.6151493613585));
#35517=CARTESIAN_POINT('Ctrl Pts',(6.18726312290577,-4.8,73.4707634940155));
#35518=CARTESIAN_POINT('Ctrl Pts',(6.14804542650294,-4.8,73.1935566226426));
#35519=CARTESIAN_POINT('Ctrl Pts',(6.13856544452442,-4.8,73.0585885938589));
#35520=CARTESIAN_POINT('Ctrl Pts',(6.13952154251132,-4.8,72.9060755452598));
#35521=CARTESIAN_POINT('',(6.48377124607659,-4.8,72.7073228862421));
#35522=CARTESIAN_POINT('Origin',(9.31,-4.8,78.));
#35523=CARTESIAN_POINT('',(7.22998432988738,-4.8,73.3715593562453));
#35524=CARTESIAN_POINT('Ctrl Pts',(6.4837712460766,-4.8,72.7073228862421));
#35525=CARTESIAN_POINT('Ctrl Pts',(6.63903811401181,-4.8,72.7956731192056));
#35526=CARTESIAN_POINT('Ctrl Pts',(6.78649185057934,-4.8,72.8961988916076));
#35527=CARTESIAN_POINT('Ctrl Pts',(6.99962383745534,-4.8,73.081316728015));
#35528=CARTESIAN_POINT('Ctrl Pts',(7.06247770883292,-4.8,73.1450491696213));
#35529=CARTESIAN_POINT('Ctrl Pts',(7.16104410153789,-4.8,73.2615985236155));
#35530=CARTESIAN_POINT('Ctrl Pts',(7.20735355880619,-4.8,73.3245142900275));
#35531=CARTESIAN_POINT('Ctrl Pts',(7.22998432988738,-4.8,73.3715593562453));
#35532=CARTESIAN_POINT('',(7.3531668006526,-4.8,73.7817890249619));
#35533=CARTESIAN_POINT('',(7.95343395333514,-4.8,75.7808347792541));
#35534=CARTESIAN_POINT('',(8.09760744867254,-4.8,73.5108347879048));
#35535=CARTESIAN_POINT('Origin',(9.30999999999986,-4.8,77.9999999999997));
#35536=CARTESIAN_POINT('',(7.92828014771504,-4.8,73.1174004638434));
#35537=CARTESIAN_POINT('',(9.00740162450745,-4.8,75.6247541297977));
#35538=CARTESIAN_POINT('',(8.07294956118024,-4.8,72.1289092826106));
#35539=CARTESIAN_POINT('Ctrl Pts',(7.92828014771504,-4.8,73.1174004638434));
#35540=CARTESIAN_POINT('Ctrl Pts',(7.91733487859675,-4.8,73.0744929233038));
#35541=CARTESIAN_POINT('Ctrl Pts',(7.91276563762517,-4.8,73.0145647221345));
#35542=CARTESIAN_POINT('Ctrl Pts',(7.90710889613904,-4.8,72.823128810336));
#35543=CARTESIAN_POINT('Ctrl Pts',(7.92467731891725,-4.8,72.6758709627745));
#35544=CARTESIAN_POINT('Ctrl Pts',(7.98263507276294,-4.8,72.4019684701976));
#35545=CARTESIAN_POINT('Ctrl Pts',(8.0198885882389,-4.8,72.2718976641637));
#35546=CARTESIAN_POINT('Ctrl Pts',(8.07294956118024,-4.8,72.1289092826106));
#35547=CARTESIAN_POINT('',(8.46441588028026,-4.8,72.0598832085154));
#35548=CARTESIAN_POINT('Origin',(9.31,-4.8,78.));
#35549=CARTESIAN_POINT('',(8.93844455602745,-4.8,72.9392812237066));
#35550=CARTESIAN_POINT('Ctrl Pts',(8.46441588028027,-4.8,72.0598832085154));
#35551=CARTESIAN_POINT('Ctrl Pts',(8.49863671609865,-4.8,72.1001506433736));
#35552=CARTESIAN_POINT('Ctrl Pts',(8.5312545173476,-4.8,72.1404481555372));
#35553=CARTESIAN_POINT('Ctrl Pts',(8.56220665880833,-4.8,72.1807659494296));
#35554=CARTESIAN_POINT('Ctrl Pts',(8.58694589561962,-4.8,72.2129909071785));
#35555=CARTESIAN_POINT('Ctrl Pts',(8.61062118189946,-4.8,72.2452312366064));
#35556=CARTESIAN_POINT('Ctrl Pts',(8.63321306170843,-4.8,72.2774597855078));
#35557=CARTESIAN_POINT('Ctrl Pts',(8.65131027380309,-4.8,72.3032764457372));
#35558=CARTESIAN_POINT('Ctrl Pts',(8.66871308103186,-4.8,72.3290863155335));
#35559=CARTESIAN_POINT('Ctrl Pts',(8.68540672089436,-4.8,72.3548377342902));
#35560=CARTESIAN_POINT('Ctrl Pts',(8.70363327657302,-4.8,72.3829538115291));
#35561=CARTESIAN_POINT('Ctrl Pts',(8.72101491260155,-4.8,72.4110010616084));
#35562=CARTESIAN_POINT('Ctrl Pts',(8.73751470277175,-4.8,72.4388383040863));
#35563=CARTESIAN_POINT('Ctrl Pts',(8.75185779942539,-4.8,72.4630369305726));
#35564=CARTESIAN_POINT('Ctrl Pts',(8.76553323921084,-4.8,72.4870707424861));
#35565=CARTESIAN_POINT('Ctrl Pts',(8.77851449432001,-4.8,72.5108524602548));
#35566=CARTESIAN_POINT('Ctrl Pts',(8.7890979878147,-4.8,72.5302414679572));
#35567=CARTESIAN_POINT('Ctrl Pts',(8.79921973972455,-4.8,72.5494617988781));
#35568=CARTESIAN_POINT('Ctrl Pts',(8.80887200369403,-4.8,72.5685058267365));
#35569=CARTESIAN_POINT('Ctrl Pts',(8.81942731012063,-4.8,72.5893315677521));
#35570=CARTESIAN_POINT('Ctrl Pts',(8.82942195864573,-4.8,72.6099505044235));
#35571=CARTESIAN_POINT('Ctrl Pts',(8.83885499921122,-4.8,72.6304025849049));
#35572=CARTESIAN_POINT('Ctrl Pts',(8.84585537382384,-4.8,72.6455803236184));
#35573=CARTESIAN_POINT('Ctrl Pts',(8.85254685047463,-4.8,72.6606682893708));
#35574=CARTESIAN_POINT('Ctrl Pts',(8.85892470594634,-4.8,72.6756618090688));
#35575=CARTESIAN_POINT('Ctrl Pts',(8.86475343918438,-4.8,72.6893644128682));
#35576=CARTESIAN_POINT('Ctrl Pts',(8.87032042714041,-4.8,72.7029891935948));
#35577=CARTESIAN_POINT('Ctrl Pts',(8.87561456216956,-4.8,72.7164944537335));
#35578=CARTESIAN_POINT('Ctrl Pts',(8.88098120268016,-4.8,72.7301846742829));
#35579=CARTESIAN_POINT('Ctrl Pts',(8.88606752585608,-4.8,72.7437524813858));
#35580=CARTESIAN_POINT('Ctrl Pts',(8.89085138995626,-4.8,72.7570995443649));
#35581=CARTESIAN_POINT('Ctrl Pts',(8.8975123163246,-4.8,72.7756836433015));
#35582=CARTESIAN_POINT('Ctrl Pts',(8.90358592752971,-4.8,72.7938359570949));
#35583=CARTESIAN_POINT('Ctrl Pts',(8.90899572675103,-4.8,72.8111960230857));
#35584=CARTESIAN_POINT('Ctrl Pts',(8.91305307616702,-4.8,72.8242160725788));
#35585=CARTESIAN_POINT('Ctrl Pts',(8.91673631861236,-4.8,72.8367867519676));
#35586=CARTESIAN_POINT('Ctrl Pts',(8.92001816856195,-4.8,72.848773246926));
#35587=CARTESIAN_POINT('Ctrl Pts',(8.92318821249884,-4.8,72.8603513861618));
#35588=CARTESIAN_POINT('Ctrl Pts',(8.9259835545623,-4.8,72.8713834266871));
#35589=CARTESIAN_POINT('Ctrl Pts',(8.92839181162883,-4.8,72.8818008291423));
#35590=CARTESIAN_POINT('Ctrl Pts',(8.93115434897723,-4.8,72.8937507425281));
#35591=CARTESIAN_POINT('Ctrl Pts',(8.93340790756747,-4.8,72.9048930113212));
#35592=CARTESIAN_POINT('Ctrl Pts',(8.93514931218717,-4.8,72.9151969740743));
#35593=CARTESIAN_POINT('Ctrl Pts',(8.93660469147692,-4.8,72.9238085131869));
#35594=CARTESIAN_POINT('Ctrl Pts',(8.93770286092992,-4.8,72.9318367583111));
#35595=CARTESIAN_POINT('Ctrl Pts',(8.93844455602745,-4.8,72.9392812237066));
#35596=CARTESIAN_POINT('',(8.91389140472481,-4.8,73.3669019025333));
#35597=CARTESIAN_POINT('',(8.79424410320319,-4.8,75.4506939040492));
#35598=CARTESIAN_POINT('',(9.70610859527519,-4.8,73.3669019025333));
#35599=CARTESIAN_POINT('Origin',(9.31,-4.8,77.9999999999998));
#35600=CARTESIAN_POINT('',(9.68155544397255,-4.8,72.9392812237066));
#35601=CARTESIAN_POINT('',(9.83803247244813,-4.8,75.6645042434626));
#35602=CARTESIAN_POINT('',(10.1555841196959,-4.8,72.059883208512));
#35603=CARTESIAN_POINT('Ctrl Pts',(9.68155544397255,-4.8,72.9392812237066));
#35604=CARTESIAN_POINT('Ctrl Pts',(9.68594549850892,-4.8,72.8952178217337));
#35605=CARTESIAN_POINT('Ctrl Pts',(9.70214846866658,-4.8,72.8373409606809));
#35606=CARTESIAN_POINT('Ctrl Pts',(9.76230780748678,-4.8,72.6555153293997));
#35607=CARTESIAN_POINT('Ctrl Pts',(9.82918187492197,-4.8,72.5231469708476));
#35608=CARTESIAN_POINT('Ctrl Pts',(9.97732451803297,-4.8,72.2855855392203));
#35609=CARTESIAN_POINT('Ctrl Pts',(10.0568182077383,-4.8,72.1761004145255));
#35610=CARTESIAN_POINT('Ctrl Pts',(10.1555841196959,-4.8,72.059883208512));
#35611=CARTESIAN_POINT('',(10.5470504387829,-4.8,72.1289092826028));
#35612=CARTESIAN_POINT('Origin',(9.31,-4.8,78.));
#35613=CARTESIAN_POINT('',(10.691719852285,-4.8,73.1174004638434));
#35614=CARTESIAN_POINT('Ctrl Pts',(10.5470504387829,-4.8,72.1289092826028));
#35615=CARTESIAN_POINT('Ctrl Pts',(10.5654352318417,-4.8,72.1784525091694));
#35616=CARTESIAN_POINT('Ctrl Pts',(10.5823033781278,-4.8,72.2274757290437));
#35617=CARTESIAN_POINT('Ctrl Pts',(10.5975993794282,-4.8,72.2759483183091));
#35618=CARTESIAN_POINT('Ctrl Pts',(10.6098250724357,-4.8,72.3146911886841));
#35619=CARTESIAN_POINT('Ctrl Pts',(10.6210457216483,-4.8,72.3530846112338));
#35620=CARTESIAN_POINT('Ctrl Pts',(10.6312523310667,-4.8,72.3910964169147));
#35621=CARTESIAN_POINT('Ctrl Pts',(10.6394283300246,-4.8,72.4215457533097));
#35622=CARTESIAN_POINT('Ctrl Pts',(10.6469541243075,-4.8,72.4517512083325));
#35623=CARTESIAN_POINT('Ctrl Pts',(10.6538335106752,-4.8,72.4816591878217));
#35624=CARTESIAN_POINT('Ctrl Pts',(10.6613446055808,-4.8,72.5143135061535));
#35625=CARTESIAN_POINT('Ctrl Pts',(10.6680852760586,-4.8,72.5466141686034));
#35626=CARTESIAN_POINT('Ctrl Pts',(10.674069109378,-4.8,72.5784158794642));
#35627=CARTESIAN_POINT('Ctrl Pts',(10.6792707939463,-4.8,72.6060607786114));
#35628=CARTESIAN_POINT('Ctrl Pts',(10.6839014561727,-4.8,72.6333224506243));
#35629=CARTESIAN_POINT('Ctrl Pts',(10.6879660194427,-4.8,72.6601098064801));
#35630=CARTESIAN_POINT('Ctrl Pts',(10.6912798190807,-4.8,72.6819492820257));
#35631=CARTESIAN_POINT('Ctrl Pts',(10.6942174144141,-4.8,72.703472328323));
#35632=CARTESIAN_POINT('Ctrl Pts',(10.6967741345915,-4.8,72.7246691295972));
#35633=CARTESIAN_POINT('Ctrl Pts',(10.6995700554658,-4.8,72.7478490534988));
#35634=CARTESIAN_POINT('Ctrl Pts',(10.7019098614498,-4.8,72.7706428885429));
#35635=CARTESIAN_POINT('Ctrl Pts',(10.7037789967056,-4.8,72.7930878487832));
#35636=CARTESIAN_POINT('Ctrl Pts',(10.7051661047424,-4.8,72.8097445271263));
#35637=CARTESIAN_POINT('Ctrl Pts',(10.7062936478012,-4.8,72.8262111971522));
#35638=CARTESIAN_POINT('Ctrl Pts',(10.7071587858016,-4.8,72.8424818521564));
#35639=CARTESIAN_POINT('Ctrl Pts',(10.7079494369223,-4.8,72.8573516320174));
#35640=CARTESIAN_POINT('Ctrl Pts',(10.708520744992,-4.8,72.8720587599544));
#35641=CARTESIAN_POINT('Ctrl Pts',(10.7088765336285,-4.8,72.8865602540843));
#35642=CARTESIAN_POINT('Ctrl Pts',(10.7092371949417,-4.8,72.901260352345));
#35643=CARTESIAN_POINT('Ctrl Pts',(10.7093763119928,-4.8,72.9157495454271));
#35644=CARTESIAN_POINT('Ctrl Pts',(10.7093067094224,-4.8,72.9299278598028));
#35645=CARTESIAN_POINT('Ctrl Pts',(10.7092097966346,-4.8,72.9496693717271));
#35646=CARTESIAN_POINT('Ctrl Pts',(10.7087086673265,-4.8,72.9688042647236));
#35647=CARTESIAN_POINT('Ctrl Pts',(10.7078547234915,-4.8,72.9869676512239));
#35648=CARTESIAN_POINT('Ctrl Pts',(10.7072142656153,-4.8,73.0005901910992));
#35649=CARTESIAN_POINT('Ctrl Pts',(10.7063759558006,-4.8,73.0136625090764));
#35650=CARTESIAN_POINT('Ctrl Pts',(10.7053602632569,-4.8,73.0260485889224));
#35651=CARTESIAN_POINT('Ctrl Pts',(10.7043791733311,-4.8,73.0380126997465));
#35652=CARTESIAN_POINT('Ctrl Pts',(10.7032327555811,-4.8,73.0493354900672));
#35653=CARTESIAN_POINT('Ctrl Pts',(10.7019328155191,-4.8,73.0599483186778));
#35654=CARTESIAN_POINT('Ctrl Pts',(10.7004416404183,-4.8,73.0721224074963));
#35655=CARTESIAN_POINT('Ctrl Pts',(10.6987484124568,-4.8,73.0833634776816));
#35656=CARTESIAN_POINT('Ctrl Pts',(10.6968606347447,-4.8,73.0936416309137));
#35657=CARTESIAN_POINT('Ctrl Pts',(10.6952829240073,-4.8,73.1022316002785));
#35658=CARTESIAN_POINT('Ctrl Pts',(10.6935690441008,-4.8,73.1101512795537));
#35659=CARTESIAN_POINT('Ctrl Pts',(10.691719852285,-4.8,73.1174004638434));
#35660=CARTESIAN_POINT('',(10.5223925513275,-4.8,73.5108347879048));
#35661=CARTESIAN_POINT('',(9.6972620259713,-4.8,75.428036967767));
#35662=CARTESIAN_POINT('',(11.2668331993474,-4.8,73.7817890249619));
#35663=CARTESIAN_POINT('Origin',(9.31000000000015,-4.8,77.9999999999997));
#35664=CARTESIAN_POINT('',(11.3900156701126,-4.8,73.3715593562453));
#35665=CARTESIAN_POINT('',(10.6049748112822,-4.8,75.9859496136124));
#35666=CARTESIAN_POINT('',(12.1362287539072,-4.8,72.7073228862334));
#35667=CARTESIAN_POINT('Ctrl Pts',(11.3900156701126,-4.8,73.3715593562453));
#35668=CARTESIAN_POINT('Ctrl Pts',(11.4092115433894,-4.8,73.3316547888187));
#35669=CARTESIAN_POINT('Ctrl Pts',(11.4442324080663,-4.8,73.2828100711267));
#35670=CARTESIAN_POINT('Ctrl Pts',(11.5629517209604,-4.8,73.1325255753574));
#35671=CARTESIAN_POINT('Ctrl Pts',(11.6710654337471,-4.8,73.0310122834859));
#35672=CARTESIAN_POINT('Ctrl Pts',(11.8915247771686,-4.8,72.8584453271068));
#35673=CARTESIAN_POINT('Ctrl Pts',(12.0036705291132,-4.8,72.7827514061615));
#35674=CARTESIAN_POINT('Ctrl Pts',(12.1362287539072,-4.8,72.7073228862334));
#35675=CARTESIAN_POINT('',(12.4804784574649,-4.8,72.906075545245));
#35676=CARTESIAN_POINT('Origin',(9.31,-4.8,78.));
#35677=CARTESIAN_POINT('',(12.2783393423437,-4.8,73.8844332675354));
#35678=CARTESIAN_POINT('Ctrl Pts',(12.4804784574649,-4.8,72.906075545245));
#35679=CARTESIAN_POINT('Ctrl Pts',(12.4808097303897,-4.8,72.9589189192183));
#35680=CARTESIAN_POINT('Ctrl Pts',(12.4798936743185,-4.8,73.0107549230007));
#35681=CARTESIAN_POINT('Ctrl Pts',(12.4776886119537,-4.8,73.0615357980059));
#35682=CARTESIAN_POINT('Ctrl Pts',(12.4759261634347,-4.8,73.1021236196345));
#35683=CARTESIAN_POINT('Ctrl Pts',(12.473338800909,-4.8,73.1420393225299));
#35684=CARTESIAN_POINT('Ctrl Pts',(12.4699290733643,-4.8,73.1812496008697));
#35685=CARTESIAN_POINT('Ctrl Pts',(12.467197712867,-4.8,73.2126589741824));
#35686=CARTESIAN_POINT('Ctrl Pts',(12.4639387721653,-4.8,73.2436167908666));
#35687=CARTESIAN_POINT('Ctrl Pts',(12.4601741493332,-4.8,73.2740739874536));
#35688=CARTESIAN_POINT('Ctrl Pts',(12.4560638351902,-4.8,73.3073279551069));
#35689=CARTESIAN_POINT('Ctrl Pts',(12.4513505163371,-4.8,73.3399860942704));
#35690=CARTESIAN_POINT('Ctrl Pts',(12.4460966546888,-4.8,73.3719165187634));
#35691=CARTESIAN_POINT('Ctrl Pts',(12.4415295269319,-4.8,73.399673307532));
#35692=CARTESIAN_POINT('Ctrl Pts',(12.4365568850902,-4.8,73.4268746794466));
#35693=CARTESIAN_POINT('Ctrl Pts',(12.4312145099132,-4.8,73.4534367227204));
#35694=CARTESIAN_POINT('Ctrl Pts',(12.4268589224052,-4.8,73.4750925031618));
#35695=CARTESIAN_POINT('Ctrl Pts',(12.4222580436605,-4.8,73.4963222679185));
#35696=CARTESIAN_POINT('Ctrl Pts',(12.4174108417078,-4.8,73.5171151956521));
#35697=CARTESIAN_POINT('Ctrl Pts',(12.4121101469542,-4.8,73.5398534607422));
#35698=CARTESIAN_POINT('Ctrl Pts',(12.4065128945608,-4.8,73.5620729204852));
#35699=CARTESIAN_POINT('Ctrl Pts',(12.4005926785574,-4.8,73.5838035662621));
#35700=CARTESIAN_POINT('Ctrl Pts',(12.3961992142276,-4.8,73.5999301428989));
#35701=CARTESIAN_POINT('Ctrl Pts',(12.3916268252751,-4.8,73.6157893936696));
#35702=CARTESIAN_POINT('Ctrl Pts',(12.3868748973112,-4.8,73.6313747027535));
#35703=CARTESIAN_POINT('Ctrl Pts',(12.3825321020783,-4.8,73.6456181438387));
#35704=CARTESIAN_POINT('Ctrl Pts',(12.3780388220321,-4.8,73.6596337223663));
#35705=CARTESIAN_POINT('Ctrl Pts',(12.3734133508682,-4.8,73.6733823563325));
#35706=CARTESIAN_POINT('Ctrl Pts',(12.3687245319211,-4.8,73.6873192836534));
#35707=CARTESIAN_POINT('Ctrl Pts',(12.3638996632849,-4.8,73.7009822523324));
#35708=CARTESIAN_POINT('Ctrl Pts',(12.3589849891398,-4.8,73.7142817042695));
#35709=CARTESIAN_POINT('Ctrl Pts',(12.3521419261712,-4.8,73.7327995112222));
#35710=CARTESIAN_POINT('Ctrl Pts',(12.3451264998134,-4.8,73.750609032654));
#35711=CARTESIAN_POINT('Ctrl Pts',(12.3381118110373,-4.8,73.7673849669295));
#35712=CARTESIAN_POINT('Ctrl Pts',(12.3328507944552,-4.8,73.7799669176362));
#35713=CARTESIAN_POINT('Ctrl Pts',(12.3275920448378,-4.8,73.7919641595396));
#35714=CARTESIAN_POINT('Ctrl Pts',(12.322401317242,-4.8,73.8032558800705));
#35715=CARTESIAN_POINT('Ctrl Pts',(12.317387427334,-4.8,73.8141629143099));
#35716=CARTESIAN_POINT('Ctrl Pts',(12.3124375246201,-4.8,73.824410758949));
#35717=CARTESIAN_POINT('Ctrl Pts',(12.3075861793309,-4.8,73.833938950071));
#35718=CARTESIAN_POINT('Ctrl Pts',(12.3020211495231,-4.8,73.8448688395031));
#35719=CARTESIAN_POINT('Ctrl Pts',(12.2965853632991,-4.8,73.8548528720717));
#35720=CARTESIAN_POINT('Ctrl Pts',(12.2912960971058,-4.8,73.8638655187556));
#35721=CARTESIAN_POINT('Ctrl Pts',(12.2868755914205,-4.8,73.8713978407167));
#35722=CARTESIAN_POINT('Ctrl Pts',(12.2825563812865,-4.8,73.8782537234236));
#35723=CARTESIAN_POINT('Ctrl Pts',(12.2783393423437,-4.8,73.8844332675354));
#35724=CARTESIAN_POINT('',(11.9846612632316,-4.8,74.1962272508773));
#35725=CARTESIAN_POINT('',(10.5535704330285,-4.8,75.7155967313038));
#35726=CARTESIAN_POINT('',(12.5915348397961,-4.8,74.7054546451438));
#35727=CARTESIAN_POINT('Origin',(9.3099999999996,-4.8,78.0000000000005));
#35728=CARTESIAN_POINT('',(12.8475953086752,-4.8,74.3620957389297));
#35729=CARTESIAN_POINT('',(11.215724076083,-4.8,76.5503191845784));
#35730=CARTESIAN_POINT('',(13.7759884897161,-4.8,73.993137535462));
#35731=CARTESIAN_POINT('Ctrl Pts',(12.8475953086752,-4.8,74.3620957389297));
#35732=CARTESIAN_POINT('Ctrl Pts',(12.879281694861,-4.8,74.3311630868456));
#35733=CARTESIAN_POINT('Ctrl Pts',(12.9288964200912,-4.8,74.2972419073571));
#35734=CARTESIAN_POINT('Ctrl Pts',(13.0918564069193,-4.8,74.1966250720879));
#35735=CARTESIAN_POINT('Ctrl Pts',(13.2281696557251,-4.8,74.1382108482666));
#35736=CARTESIAN_POINT('Ctrl Pts',(13.4943550490169,-4.8,74.0514524889784));
#35737=CARTESIAN_POINT('Ctrl Pts',(13.6256264304604,-4.8,74.0186795760604));
#35738=CARTESIAN_POINT('Ctrl Pts',(13.7759884897161,-4.8,73.993137535462));
#35739=CARTESIAN_POINT('',(14.0314999829165,-4.8,74.2976442754215));
#35740=CARTESIAN_POINT('Origin',(9.31,-4.8,78.));
#35741=CARTESIAN_POINT('',(13.5069332996928,-4.8,75.1478641584586));
#35742=CARTESIAN_POINT('Ctrl Pts',(14.0314999829165,-4.8,74.2976442754215));
#35743=CARTESIAN_POINT('Ctrl Pts',(14.0137377793038,-4.8,74.3474141060163));
#35744=CARTESIAN_POINT('Ctrl Pts',(13.9951480107643,-4.8,74.3958107066136));
#35745=CARTESIAN_POINT('Ctrl Pts',(13.9757078478022,-4.8,74.4427749443781));
#35746=CARTESIAN_POINT('Ctrl Pts',(13.9601698370925,-4.8,74.4803122238127));
#35747=CARTESIAN_POINT('Ctrl Pts',(13.9440865390346,-4.8,74.5169357812344));
#35748=CARTESIAN_POINT('Ctrl Pts',(13.9274717401505,-4.8,74.5526151912231));
#35749=CARTESIAN_POINT('Ctrl Pts',(13.9141624622321,-4.8,74.5811961681471));
#35750=CARTESIAN_POINT('Ctrl Pts',(13.9005118625272,-4.8,74.6091723775572));
#35751=CARTESIAN_POINT('Ctrl Pts',(13.8865572991921,-4.8,74.6365052044542));
#35752=CARTESIAN_POINT('Ctrl Pts',(13.8713213407319,-4.8,74.6663479021583));
#35753=CARTESIAN_POINT('Ctrl Pts',(13.8557225285405,-4.8,74.6954244644896));
#35754=CARTESIAN_POINT('Ctrl Pts',(13.8398646653426,-4.8,74.7236323222161));
#35755=CARTESIAN_POINT('Ctrl Pts',(13.826079588047,-4.8,74.7481531226702));
#35756=CARTESIAN_POINT('Ctrl Pts',(13.8121034158961,-4.8,74.7720133080073));
#35757=CARTESIAN_POINT('Ctrl Pts',(13.797998471323,-4.8,74.7951462646713));
#35758=CARTESIAN_POINT('Ctrl Pts',(13.7864988446753,-4.8,74.8140063433844));
#35759=CARTESIAN_POINT('Ctrl Pts',(13.7749144256038,-4.8,74.8323822037526));
#35760=CARTESIAN_POINT('Ctrl Pts',(13.7632479454926,-4.8,74.8502633240851));
#35761=CARTESIAN_POINT('Ctrl Pts',(13.7504899762601,-4.8,74.8698173610244));
#35762=CARTESIAN_POINT('Ctrl Pts',(13.7376307758707,-4.8,74.8887824516424));
#35763=CARTESIAN_POINT('Ctrl Pts',(13.7246352731669,-4.8,74.9071777472498));
#35764=CARTESIAN_POINT('Ctrl Pts',(13.7149911530288,-4.8,74.9208291191789));
#35765=CARTESIAN_POINT('Ctrl Pts',(13.7052703295732,-4.8,74.934168091134));
#35766=CARTESIAN_POINT('Ctrl Pts',(13.6954744882065,-4.8,74.9471882361456));
#35767=CARTESIAN_POINT('Ctrl Pts',(13.6865220518115,-4.8,74.9590873692274));
#35768=CARTESIAN_POINT('Ctrl Pts',(13.6775061395318,-4.8,74.9707209127091));
#35769=CARTESIAN_POINT('Ctrl Pts',(13.6684573086483,-4.8,74.9820583983343));
#35770=CARTESIAN_POINT('Ctrl Pts',(13.6592845502886,-4.8,74.9935511555076));
#35771=CARTESIAN_POINT('Ctrl Pts',(13.6500776464114,-4.8,75.0047399440415));
#35772=CARTESIAN_POINT('Ctrl Pts',(13.6409106830007,-4.8,75.0155564232949));
#35773=CARTESIAN_POINT('Ctrl Pts',(13.6281468440578,-4.8,75.0306170047475));
#35774=CARTESIAN_POINT('Ctrl Pts',(13.6154632844137,-4.8,75.0449530637636));
#35775=CARTESIAN_POINT('Ctrl Pts',(13.6031339254938,-4.8,75.0583181208055));
#35776=CARTESIAN_POINT('Ctrl Pts',(13.5938869063039,-4.8,75.0683419135868));
#35777=CARTESIAN_POINT('Ctrl Pts',(13.5848419995513,-4.8,75.0778170351574));
#35778=CARTESIAN_POINT('Ctrl Pts',(13.5761023151156,-4.8,75.0866524483868));
#35779=CARTESIAN_POINT('Ctrl Pts',(13.5676603743603,-4.8,75.095186856646));
#35780=CARTESIAN_POINT('Ctrl Pts',(13.5595040180152,-4.8,75.1031237142177));
#35781=CARTESIAN_POINT('Ctrl Pts',(13.5516864113499,-4.8,75.1104180273209));
#35782=CARTESIAN_POINT('Ctrl Pts',(13.5427187516189,-4.8,75.1187854114427));
#35783=CARTESIAN_POINT('Ctrl Pts',(13.5341960432185,-4.8,75.1263081847801));
#35784=CARTESIAN_POINT('Ctrl Pts',(13.5261432521403,-4.8,75.1329682667954));
#35785=CARTESIAN_POINT('Ctrl Pts',(13.5194131292823,-4.8,75.1385344325844));
#35786=CARTESIAN_POINT('Ctrl Pts',(13.513009548998,-4.8,75.1434995984469));
#35787=CARTESIAN_POINT('Ctrl Pts',(13.5069332996928,-4.8,75.1478641584586));
#35788=CARTESIAN_POINT('',(13.1243263529939,-4.8,75.340410845101));
#35789=CARTESIAN_POINT('',(11.2598858927175,-4.8,76.278689243247));
#35790=CARTESIAN_POINT('',(13.5204349482691,-4.8,76.0264910574324));
#35791=CARTESIAN_POINT('Origin',(9.31000000000134,-4.8,77.9999999999992));
#35792=CARTESIAN_POINT('',(13.8784887436653,-4.8,75.7914170652479));
#35793=CARTESIAN_POINT('',(11.5966148918162,-4.8,77.2895416568946));
#35794=CARTESIAN_POINT('',(14.8770841027247,-4.8,75.7622389329533));
#35795=CARTESIAN_POINT('Ctrl Pts',(13.8784887436653,-4.8,75.7914170652479));
#35796=CARTESIAN_POINT('Ctrl Pts',(13.9188438003731,-4.8,75.7731872611009));
#35797=CARTESIAN_POINT('Ctrl Pts',(13.9770681225745,-4.8,75.7582810146635));
#35798=CARTESIAN_POINT('Ctrl Pts',(14.1646133920406,-4.8,75.7194677169264));
#35799=CARTESIAN_POINT('Ctrl Pts',(14.3126847875687,-4.8,75.7111981783716));
#35800=CARTESIAN_POINT('Ctrl Pts',(14.5924903467623,-4.8,75.7207127544627));
#35801=CARTESIAN_POINT('Ctrl Pts',(14.7270540920481,-4.8,75.7348137468176));
#35802=CARTESIAN_POINT('Ctrl Pts',(14.8770841027247,-4.8,75.7622389329533));
#35803=CARTESIAN_POINT('',(15.0130389285309,-4.8,76.1357717468986));
#35804=CARTESIAN_POINT('Origin',(9.31,-4.8,78.));
#35805=CARTESIAN_POINT('',(14.2293151609602,-4.8,76.7553047249138));
#35806=CARTESIAN_POINT('Ctrl Pts',(15.0130389285309,-4.8,76.1357717468986));
#35807=CARTESIAN_POINT('Ctrl Pts',(14.9793256322769,-4.8,76.1764650580252));
#35808=CARTESIAN_POINT('Ctrl Pts',(14.9453043517147,-4.8,76.2155849111935));
#35809=CARTESIAN_POINT('Ctrl Pts',(14.9109738587163,-4.8,76.2530679315487));
#35810=CARTESIAN_POINT('Ctrl Pts',(14.8835344011301,-4.8,76.2830271211033));
#35811=CARTESIAN_POINT('Ctrl Pts',(14.8558950524031,-4.8,76.3119411937235));
#35812=CARTESIAN_POINT('Ctrl Pts',(14.8280791737289,-4.8,76.3397862741419));
#35813=CARTESIAN_POINT('Ctrl Pts',(14.8057972733803,-4.8,76.362091566538));
#35814=CARTESIAN_POINT('Ctrl Pts',(14.7834014781299,-4.8,76.3837118244195));
#35815=CARTESIAN_POINT('Ctrl Pts',(14.7609401002719,-4.8,76.4046235388012));
#35816=CARTESIAN_POINT('Ctrl Pts',(14.7364161792257,-4.8,76.4274554966482));
#35817=CARTESIAN_POINT('Ctrl Pts',(14.7118133209326,-4.8,76.4494434194877));
#35818=CARTESIAN_POINT('Ctrl Pts',(14.6872641487802,-4.8,76.4705264263976));
#35819=CARTESIAN_POINT('Ctrl Pts',(14.6659238053871,-4.8,76.4888536679202));
#35820=CARTESIAN_POINT('Ctrl Pts',(14.6446298352381,-4.8,76.5064947759896));
#35821=CARTESIAN_POINT('Ctrl Pts',(14.6234635854471,-4.8,76.5234084698624));
#35822=CARTESIAN_POINT('Ctrl Pts',(14.6062069441493,-4.8,76.537198042936));
#35823=CARTESIAN_POINT('Ctrl Pts',(14.5890362364622,-4.8,76.5505035988803));
#35824=CARTESIAN_POINT('Ctrl Pts',(14.5719576276826,-4.8,76.5633161847262));
#35825=CARTESIAN_POINT('Ctrl Pts',(14.5532811825371,-4.8,76.5773274873921));
#35826=CARTESIAN_POINT('Ctrl Pts',(14.5347110427406,-4.8,76.5907507383831));
#35827=CARTESIAN_POINT('Ctrl Pts',(14.5162077020452,-4.8,76.6035919390039));
#35828=CARTESIAN_POINT('Ctrl Pts',(14.5024761492368,-4.8,76.613121549216));
#35829=CARTESIAN_POINT('Ctrl Pts',(14.4887793659718,-4.8,76.622331365394));
#35830=CARTESIAN_POINT('Ctrl Pts',(14.475121134166,-4.8,76.6312159246056));
#35831=CARTESIAN_POINT('Ctrl Pts',(14.4626388525233,-4.8,76.6393355386176));
#35832=CARTESIAN_POINT('Ctrl Pts',(14.4501877600528,-4.8,76.647183870011));
#35833=CARTESIAN_POINT('Ctrl Pts',(14.437806991961,-4.8,76.6547427391965));
#35834=CARTESIAN_POINT('Ctrl Pts',(14.4252566642583,-4.8,76.6624051301431));
#35835=CARTESIAN_POINT('Ctrl Pts',(14.4127782136582,-4.8,76.6697702055542));
#35836=CARTESIAN_POINT('Ctrl Pts',(14.4004646320838,-4.8,76.676799085134));
#35837=CARTESIAN_POINT('Ctrl Pts',(14.3833195243853,-4.8,76.6865859125219));
#35838=CARTESIAN_POINT('Ctrl Pts',(14.3664976558123,-4.8,76.6957193686518));
#35839=CARTESIAN_POINT('Ctrl Pts',(14.3503407292824,-4.8,76.7040615251609));
#35840=CARTESIAN_POINT('Ctrl Pts',(14.3382230343849,-4.8,76.7103181425427));
#35841=CARTESIAN_POINT('Ctrl Pts',(14.3264829196606,-4.8,76.7161283041536));
#35842=CARTESIAN_POINT('Ctrl Pts',(14.3152484132406,-4.8,76.7214417287278));
#35843=CARTESIAN_POINT('Ctrl Pts',(14.3043966442584,-4.8,76.7265741354244));
#35844=CARTESIAN_POINT('Ctrl Pts',(14.2940176112058,-4.8,76.7312427037723));
#35845=CARTESIAN_POINT('Ctrl Pts',(14.284176661876,-4.8,76.7354233370412));
#35846=CARTESIAN_POINT('Ctrl Pts',(14.2728880043614,-4.8,76.740218985874));
#35847=CARTESIAN_POINT('Ctrl Pts',(14.262306338214,-4.8,76.7443731425178));
#35848=CARTESIAN_POINT('Ctrl Pts',(14.252461307702,-4.8,76.7478773556981));
#35849=CARTESIAN_POINT('Ctrl Pts',(14.2442333196509,-4.8,76.7508060032163));
#35850=CARTESIAN_POINT('Ctrl Pts',(14.2365177353778,-4.8,76.7532815796345));
#35851=CARTESIAN_POINT('Ctrl Pts',(14.2293151609602,-4.8,76.7553047249138));
#35852=CARTESIAN_POINT('',(13.8039273911235,-4.8,76.805380142761));
#35853=CARTESIAN_POINT('',(11.7310163364939,-4.8,77.0493972362957));
#35854=CARTESIAN_POINT('',(13.941494462579,-4.8,77.5855617740846));
#35855=CARTESIAN_POINT('Origin',(9.30999999999972,-4.8,78.0000000000001));
#35856=CARTESIAN_POINT('',(14.3583550124563,-4.8,77.4871260887099));
#35857=CARTESIAN_POINT('',(11.7017062047547,-4.8,78.1144558906375));
#35858=CARTESIAN_POINT('',(15.3067072115039,-4.8,77.8012473409061));
#35859=CARTESIAN_POINT('Ctrl Pts',(14.3583550124563,-4.8,77.4871260887099));
#35860=CARTESIAN_POINT('Ctrl Pts',(14.4025113203035,-4.8,77.4837979186678));
#35861=CARTESIAN_POINT('Ctrl Pts',(14.4623225212488,-4.8,77.4897045193554));
#35862=CARTESIAN_POINT('Ctrl Pts',(14.6555084752939,-4.8,77.5179129863291));
#35863=CARTESIAN_POINT('Ctrl Pts',(14.7941933832081,-4.8,77.5619464951834));
#35864=CARTESIAN_POINT('Ctrl Pts',(15.0510922509005,-4.8,77.6624620772393));
#35865=CARTESIAN_POINT('Ctrl Pts',(15.1814858790588,-4.8,77.7279002923833));
#35866=CARTESIAN_POINT('Ctrl Pts',(15.3067072115039,-4.8,77.8012473409061));
#35867=CARTESIAN_POINT('',(15.306707211514,-4.8,78.1987526587886));
#35868=CARTESIAN_POINT('Origin',(9.31,-4.8,78.));
#35869=CARTESIAN_POINT('',(14.3583550124563,-4.8,78.5128739112901));
#35870=CARTESIAN_POINT('Ctrl Pts',(15.306707211514,-4.8,78.1987526587886));
#35871=CARTESIAN_POINT('Ctrl Pts',(15.1815741357754,-4.8,78.2720480119657));
#35872=CARTESIAN_POINT('Ctrl Pts',(14.9949210075704,-4.8,78.369958518309));
#35873=CARTESIAN_POINT('Ctrl Pts',(14.5626620354579,-4.8,78.5088509137435));
#35874=CARTESIAN_POINT('Ctrl Pts',(14.4186035570618,-4.8,78.5174149926455));
#35875=CARTESIAN_POINT('Ctrl Pts',(14.3583550124563,-4.8,78.5128739112901));
#35876=CARTESIAN_POINT('',(13.941494462579,-4.8,78.4144382259154));
#35877=CARTESIAN_POINT('',(11.9101364796933,-4.8,77.9347619520498));
#35878=CARTESIAN_POINT('',(13.8039273911235,-4.8,79.194619857239));
#35879=CARTESIAN_POINT('Origin',(9.30999999999925,-4.8,77.9999999999999));
#35880=CARTESIAN_POINT('',(14.2293151609602,-4.8,79.2446952750862));
#35881=CARTESIAN_POINT('',(11.5183224515755,-4.8,78.9255650547807));
#35882=CARTESIAN_POINT('',(15.0130389285914,-4.8,79.8642282529162));
#35883=CARTESIAN_POINT('Ctrl Pts',(14.2293151609602,-4.8,79.2446952750862));
#35884=CARTESIAN_POINT('Ctrl Pts',(14.2719468183276,-4.8,79.2566701648679));
#35885=CARTESIAN_POINT('Ctrl Pts',(14.3261307856426,-4.8,79.2826771890912));
#35886=CARTESIAN_POINT('Ctrl Pts',(14.4947475082523,-4.8,79.37349625589));
#35887=CARTESIAN_POINT('Ctrl Pts',(14.6134923348285,-4.8,79.462339880326));
#35888=CARTESIAN_POINT('Ctrl Pts',(14.8217199770457,-4.8,79.649484015153));
#35889=CARTESIAN_POINT('Ctrl Pts',(14.9157378424995,-4.8,79.7467819095626));
#35890=CARTESIAN_POINT('Ctrl Pts',(15.0130389285914,-4.8,79.8642282529162));
#35891=CARTESIAN_POINT('',(14.877084102819,-4.8,80.237761066812));
#35892=CARTESIAN_POINT('Origin',(9.31,-4.8,78.));
#35893=CARTESIAN_POINT('',(13.8784887436653,-4.8,80.2085829347521));
#35894=CARTESIAN_POINT('Ctrl Pts',(14.877084102819,-4.8,80.237761066812));
#35895=CARTESIAN_POINT('Ctrl Pts',(14.7013523439929,-4.8,80.2698844812177));
#35896=CARTESIAN_POINT('Ctrl Pts',(14.5237795116491,-4.8,80.28765870646));
#35897=CARTESIAN_POINT('Ctrl Pts',(14.2415194834978,-4.8,80.2828488169659));
#35898=CARTESIAN_POINT('Ctrl Pts',(14.152404201208,-4.8,80.2744286239328));
#35899=CARTESIAN_POINT('Ctrl Pts',(14.0019814789273,-4.8,80.2485038942336));
#35900=CARTESIAN_POINT('Ctrl Pts',(13.9260649040323,-4.8,80.2300747661684));
#35901=CARTESIAN_POINT('Ctrl Pts',(13.8784887436653,-4.8,80.2085829347521));
#35902=CARTESIAN_POINT('',(13.5204349482691,-4.8,79.9735089425676));
#35903=CARTESIAN_POINT('',(11.7756417895143,-4.8,78.8279953391977));
#35904=CARTESIAN_POINT('',(13.1243263529939,-4.8,80.659589154899));
#35905=CARTESIAN_POINT('Origin',(9.31000000000061,-4.8,78.0000000000004));
#35906=CARTESIAN_POINT('',(13.5069332996928,-4.8,80.8521358415414));
#35907=CARTESIAN_POINT('',(11.0685824193681,-4.8,79.6250374134319));
#35908=CARTESIAN_POINT('',(14.0314999829639,-4.8,81.7023557245181));
#35909=CARTESIAN_POINT('Ctrl Pts',(13.5069332996928,-4.8,80.8521358415414));
#35910=CARTESIAN_POINT('Ctrl Pts',(13.5428982988443,-4.8,80.8779694418353));
#35911=CARTESIAN_POINT('Ctrl Pts',(13.5849196460621,-4.8,80.9209400573754));
#35912=CARTESIAN_POINT('Ctrl Pts',(13.7123055878643,-4.8,81.0639523822528));
#35913=CARTESIAN_POINT('Ctrl Pts',(13.7935029159474,-4.8,81.1880512030957));
#35914=CARTESIAN_POINT('Ctrl Pts',(13.925165831458,-4.8,81.4351272145176));
#35915=CARTESIAN_POINT('Ctrl Pts',(13.980235885705,-4.8,81.5587133313075));
#35916=CARTESIAN_POINT('Ctrl Pts',(14.0314999829639,-4.8,81.7023557245181));
#35917=CARTESIAN_POINT('',(13.7759884899248,-4.8,82.0068624643054));
#35918=CARTESIAN_POINT('Origin',(9.31,-4.8,78.));
#35919=CARTESIAN_POINT('',(12.8475953086752,-4.8,81.6379042610703));
#35920=CARTESIAN_POINT('Ctrl Pts',(13.7759884899248,-4.8,82.0068624643054));
#35921=CARTESIAN_POINT('Ctrl Pts',(13.7238904006001,-4.8,81.998012548872));
#35922=CARTESIAN_POINT('Ctrl Pts',(13.6730009737443,-4.8,81.9881091822482));
#35923=CARTESIAN_POINT('Ctrl Pts',(13.6233744794367,-4.8,81.9771196133808));
#35924=CARTESIAN_POINT('Ctrl Pts',(13.5837093382832,-4.8,81.9683359423513));
#35925=CARTESIAN_POINT('Ctrl Pts',(13.5448493490778,-4.8,81.9588566022824));
#35926=CARTESIAN_POINT('Ctrl Pts',(13.5068268689897,-4.8,81.94868988692));
#35927=CARTESIAN_POINT('Ctrl Pts',(13.476368967432,-4.8,81.9405458412145));
#35928=CARTESIAN_POINT('Ctrl Pts',(13.446447375747,-4.8,81.9319606423288));
#35929=CARTESIAN_POINT('Ctrl Pts',(13.417106609469,-4.8,81.9229643754468));
#35930=CARTESIAN_POINT('Ctrl Pts',(13.3850715928299,-4.8,81.9131420157808));
#35931=CARTESIAN_POINT('Ctrl Pts',(13.3537280633307,-4.8,81.9028292769294));
#35932=CARTESIAN_POINT('Ctrl Pts',(13.3231950570889,-4.8,81.8921105736537));
#35933=CARTESIAN_POINT('Ctrl Pts',(13.2966530278779,-4.8,81.8827929148161));
#35934=CARTESIAN_POINT('Ctrl Pts',(13.2707283943044,-4.8,81.8731723496375));
#35935=CARTESIAN_POINT('Ctrl Pts',(13.2454975801038,-4.8,81.8632986864201));
#35936=CARTESIAN_POINT('Ctrl Pts',(13.2249271382615,-4.8,81.8552487831007));
#35937=CARTESIAN_POINT('Ctrl Pts',(13.2048188343683,-4.8,81.8470312918966));
#35938=CARTESIAN_POINT('Ctrl Pts',(13.1851835045775,-4.8,81.8386470756315));
#35939=CARTESIAN_POINT('Ctrl Pts',(13.1637111360262,-4.8,81.8294784503231));
#35940=CARTESIAN_POINT('Ctrl Pts',(13.1428011879323,-4.8,81.8201078622799));
#35941=CARTESIAN_POINT('Ctrl Pts',(13.1224287098858,-4.8,81.8105040987335));
#35942=CARTESIAN_POINT('Ctrl Pts',(13.1073100487301,-4.8,81.8033770302175));
#35943=CARTESIAN_POINT('Ctrl Pts',(13.0924857221107,-4.8,81.7961201759903));
#35944=CARTESIAN_POINT('Ctrl Pts',(13.0779623520226,-4.8,81.7887340798196));
#35945=CARTESIAN_POINT('Ctrl Pts',(13.0646894190553,-4.8,81.7819839137929));
#35946=CARTESIAN_POINT('Ctrl Pts',(13.0516670183166,-4.8,81.7751251170702));
#35947=CARTESIAN_POINT('Ctrl Pts',(13.038930461394,-4.8,81.7681824919383));
#35948=CARTESIAN_POINT('Ctrl Pts',(13.0260194723549,-4.8,81.7611447848463));
#35949=CARTESIAN_POINT('Ctrl Pts',(13.0134019046673,-4.8,81.7540206673816));
#35950=CARTESIAN_POINT('Ctrl Pts',(13.0011579256109,-4.8,81.7468712327598));
#35951=CARTESIAN_POINT('Ctrl Pts',(12.9841097302923,-4.8,81.7369165474986));
#35952=CARTESIAN_POINT('Ctrl Pts',(12.9677889906484,-4.8,81.7269151098885));
#35953=CARTESIAN_POINT('Ctrl Pts',(12.9524860076116,-4.8,81.7170938791618));
#35954=CARTESIAN_POINT('Ctrl Pts',(12.941008770334,-4.8,81.7097279561167));
#35955=CARTESIAN_POINT('Ctrl Pts',(12.9301069651891,-4.8,81.7024657992042));
#35956=CARTESIAN_POINT('Ctrl Pts',(12.9198881511031,-4.8,81.6953931434104));
#35957=CARTESIAN_POINT('Ctrl Pts',(12.910017471913,-4.8,81.6885614390878));
#35958=CARTESIAN_POINT('Ctrl Pts',(12.9007848564824,-4.8,81.6819072169133));
#35959=CARTESIAN_POINT('Ctrl Pts',(12.8922438470947,-4.8,81.6754750213747));
#35960=CARTESIAN_POINT('Ctrl Pts',(12.8824463647866,-4.8,81.6680965817627));
#35961=CARTESIAN_POINT('Ctrl Pts',(12.8735579266505,-4.8,81.6610096685258));
#35962=CARTESIAN_POINT('Ctrl Pts',(12.8656006738454,-4.8,81.6542357287195));
#35963=CARTESIAN_POINT('Ctrl Pts',(12.8589503961148,-4.8,81.6485744053777));
#35964=CARTESIAN_POINT('Ctrl Pts',(12.8529486914522,-4.8,81.6431303012078));
#35965=CARTESIAN_POINT('Ctrl Pts',(12.8475953086752,-4.8,81.6379042610703));
#35966=CARTESIAN_POINT('',(12.5915348397961,-4.8,81.2945453548562));
#35967=CARTESIAN_POINT('',(11.3437543105226,-4.8,79.6213602685287));
#35968=CARTESIAN_POINT('',(11.9846612632316,-4.8,81.8037727491227));
#35969=CARTESIAN_POINT('Origin',(9.31000000000031,-4.8,78.0000000000004));
#35970=CARTESIAN_POINT('',(12.2783393423437,-4.8,82.1155667324646));
#35971=CARTESIAN_POINT('',(10.4067313934724,-4.8,80.1285062770252));
#35972=CARTESIAN_POINT('',(12.4804784574569,-4.8,83.09392445476));
#35973=CARTESIAN_POINT('Ctrl Pts',(12.2783393423437,-4.8,82.1155667324646));
#35974=CARTESIAN_POINT('Ctrl Pts',(12.3032997740142,-4.8,82.1521431288428));
#35975=CARTESIAN_POINT('Ctrl Pts',(12.3280901075719,-4.8,82.2068944444417));
#35976=CARTESIAN_POINT('Ctrl Pts',(12.3988806429637,-4.8,82.3848506340573));
#35977=CARTESIAN_POINT('Ctrl Pts',(12.4327368762941,-4.8,82.5292365018844));
#35978=CARTESIAN_POINT('Ctrl Pts',(12.4719545734303,-4.8,82.8064433756322));
#35979=CARTESIAN_POINT('Ctrl Pts',(12.4814345554706,-4.8,82.9414114045802));
#35980=CARTESIAN_POINT('Ctrl Pts',(12.4804784574569,-4.8,83.0939244547599));
#35981=CARTESIAN_POINT('',(12.1362287541399,-4.8,83.2926771136423));
#35982=CARTESIAN_POINT('Origin',(9.31,-4.8,78.));
#35983=CARTESIAN_POINT('',(11.3900156701126,-4.8,82.6284406437547));
#35984=CARTESIAN_POINT('Ctrl Pts',(12.1362287541399,-4.8,83.2926771136423));
#35985=CARTESIAN_POINT('Ctrl Pts',(12.0902994133922,-4.8,83.2665423174371));
#35986=CARTESIAN_POINT('Ctrl Pts',(12.0458661453988,-4.8,83.2398309878294));
#35987=CARTESIAN_POINT('Ctrl Pts',(12.0029911488357,-4.8,83.2125309103598));
#35988=CARTESIAN_POINT('Ctrl Pts',(11.9687223008297,-4.8,83.1907106822467));
#35989=CARTESIAN_POINT('Ctrl Pts',(11.9354479809844,-4.8,83.1685121172559));
#35990=CARTESIAN_POINT('Ctrl Pts',(11.9031957584663,-4.8,83.1459540757644));
#35991=CARTESIAN_POINT('Ctrl Pts',(11.8773601205811,-4.8,83.1278839600987));
#35992=CARTESIAN_POINT('Ctrl Pts',(11.8521793324076,-4.8,83.1095827248216));
#35993=CARTESIAN_POINT('Ctrl Pts',(11.8276849351316,-4.8,83.0910938659688));
#35994=CARTESIAN_POINT('Ctrl Pts',(11.800941310303,-4.8,83.0709072453674));
#35995=CARTESIAN_POINT('Ctrl Pts',(11.775015190457,-4.8,83.0504963215801));
#35996=CARTESIAN_POINT('Ctrl Pts',(11.7499895614165,-4.8,83.0299811312968));
#35997=CARTESIAN_POINT('Ctrl Pts',(11.7282350396413,-4.8,83.0121474875143));
#35998=CARTESIAN_POINT('Ctrl Pts',(11.707164280057,-4.8,82.9942403666271));
#35999=CARTESIAN_POINT('Ctrl Pts',(11.6868320620375,-4.8,82.9763327115825));
#36000=CARTESIAN_POINT('Ctrl Pts',(11.6702553987293,-4.8,82.9617327713285));
#36001=CARTESIAN_POINT('Ctrl Pts',(11.6541703214774,-4.8,82.9471334104638));
#36002=CARTESIAN_POINT('Ctrl Pts',(11.6385867178304,-4.8,82.9325391459589));
#36003=CARTESIAN_POINT('Ctrl Pts',(11.6215451465656,-4.8,82.9165794742263));
#36004=CARTESIAN_POINT('Ctrl Pts',(11.6051011529476,-4.8,82.9006223787257));
#36005=CARTESIAN_POINT('Ctrl Pts',(11.5892419666579,-4.8,82.8846299955104));
#36006=CARTESIAN_POINT('Ctrl Pts',(11.5774726734063,-4.8,82.8727618552153));
#36007=CARTESIAN_POINT('Ctrl Pts',(11.5660243534712,-4.8,82.8608724245862));
#36008=CARTESIAN_POINT('Ctrl Pts',(11.554903043514,-4.8,82.848964479454));
#36009=CARTESIAN_POINT('Ctrl Pts',(11.5447392590945,-4.8,82.8380817877867));
#36010=CARTESIAN_POINT('Ctrl Pts',(11.5348480518501,-4.8,82.8271827037259));
#36011=CARTESIAN_POINT('Ctrl Pts',(11.5252541209383,-4.8,82.816302611073));
#36012=CARTESIAN_POINT('Ctrl Pts',(11.5155287973603,-4.8,82.8052735112617));
#36013=CARTESIAN_POINT('Ctrl Pts',(11.5061087537551,-4.8,82.7942635682762));
#36014=CARTESIAN_POINT('Ctrl Pts',(11.4970484276151,-4.8,82.7833576097878));
#36015=CARTESIAN_POINT('Ctrl Pts',(11.4844330673021,-4.8,82.7681724394347));
#36016=CARTESIAN_POINT('Ctrl Pts',(11.472517281958,-4.8,82.7531921407433));
#36017=CARTESIAN_POINT('Ctrl Pts',(11.4614962405913,-4.8,82.7387292743878));
#36018=CARTESIAN_POINT('Ctrl Pts',(11.4532304595662,-4.8,82.7278821246212));
#36019=CARTESIAN_POINT('Ctrl Pts',(11.4454699177556,-4.8,82.7173292925021));
#36020=CARTESIAN_POINT('Ctrl Pts',(11.4382863643943,-4.8,82.7071881298805));
#36021=CARTESIAN_POINT('Ctrl Pts',(11.4313475404717,-4.8,82.6973924565885));
#36022=CARTESIAN_POINT('Ctrl Pts',(11.4249475978921,-4.8,82.6879817926255));
#36023=CARTESIAN_POINT('Ctrl Pts',(11.4191216148336,-4.8,82.6790163086589));
#36024=CARTESIAN_POINT('Ctrl Pts',(11.412438568019,-4.8,82.6687319071316));
#36025=CARTESIAN_POINT('Ctrl Pts',(11.4065100354132,-4.8,82.6590323622077));
#36026=CARTESIAN_POINT('Ctrl Pts',(11.4013494875778,-4.8,82.6499454002511));
#36027=CARTESIAN_POINT('Ctrl Pts',(11.3970365574561,-4.8,82.6423509678021));
#36028=CARTESIAN_POINT('Ctrl Pts',(11.3932587932986,-4.8,82.6351824796365));
#36029=CARTESIAN_POINT('Ctrl Pts',(11.3900156701126,-4.8,82.6284406437547));
#36030=CARTESIAN_POINT('',(11.2668331993474,-4.8,82.2182109750381));
#36031=CARTESIAN_POINT('',(10.6665660466648,-4.8,80.2191652207459));
#36032=CARTESIAN_POINT('',(10.5223925513275,-4.8,82.4891652120952));
#36033=CARTESIAN_POINT('Origin',(9.31000000000013,-4.8,78.0000000000003));
#36034=CARTESIAN_POINT('',(10.691719852285,-4.8,82.8825995361566));
#36035=CARTESIAN_POINT('',(9.61259837549256,-4.8,80.3752458702023));
#36036=CARTESIAN_POINT('',(10.5470504386678,-4.8,83.8710907174214));
#36037=CARTESIAN_POINT('Ctrl Pts',(10.691719852285,-4.8,82.8825995361566));
#36038=CARTESIAN_POINT('Ctrl Pts',(10.7026651208567,-4.8,82.9255070744082));
#36039=CARTESIAN_POINT('Ctrl Pts',(10.7072343621118,-4.8,82.9854352727938));
#36040=CARTESIAN_POINT('Ctrl Pts',(10.7128911041171,-4.8,83.1768711873215));
#36041=CARTESIAN_POINT('Ctrl Pts',(10.6953226813375,-4.8,83.3241290352659));
#36042=CARTESIAN_POINT('Ctrl Pts',(10.6373649270984,-4.8,83.5980315310389));
#36043=CARTESIAN_POINT('Ctrl Pts',(10.6001114118967,-4.8,83.7281023352314));
#36044=CARTESIAN_POINT('Ctrl Pts',(10.5470504386678,-4.8,83.8710907174214));
#36045=CARTESIAN_POINT('',(10.1555841198781,-4.8,83.9401167914621));
#36046=CARTESIAN_POINT('Origin',(9.31,-4.8,78.));
#36047=CARTESIAN_POINT('',(9.68155544397255,-4.8,83.0607187762934));
#36048=CARTESIAN_POINT('Ctrl Pts',(10.1555841198781,-4.8,83.9401167914621));
#36049=CARTESIAN_POINT('Ctrl Pts',(10.1213632840485,-4.8,83.8998493566156));
#36050=CARTESIAN_POINT('Ctrl Pts',(10.0887454828079,-4.8,83.8595518445941));
#36051=CARTESIAN_POINT('Ctrl Pts',(10.0577933413463,-4.8,83.8192340507748));
#36052=CARTESIAN_POINT('Ctrl Pts',(10.0330541147877,-4.8,83.78700910644));
#36053=CARTESIAN_POINT('Ctrl Pts',(10.0093788378727,-4.8,83.7547687903993));
#36054=CARTESIAN_POINT('Ctrl Pts',(9.98678696651789,-4.8,83.7225402548213));
#36055=CARTESIAN_POINT('Ctrl Pts',(9.96868975187523,-4.8,83.6967235919687));
#36056=CARTESIAN_POINT('Ctrl Pts',(9.95128694223038,-4.8,83.6709137195168));
#36057=CARTESIAN_POINT('Ctrl Pts',(9.93459330008706,-4.8,83.6451622980894));
#36058=CARTESIAN_POINT('Ctrl Pts',(9.9163667435806,-4.8,83.6170462204991));
#36059=CARTESIAN_POINT('Ctrl Pts',(9.89898510673091,-4.8,83.588998970037));
#36060=CARTESIAN_POINT('Ctrl Pts',(9.88248531574176,-4.8,83.5611617271314));
#36061=CARTESIAN_POINT('Ctrl Pts',(9.86814221774207,-4.8,83.5369630992034));
#36062=CARTESIAN_POINT('Ctrl Pts',(9.85446677667117,-4.8,83.5129292858282));
#36063=CARTESIAN_POINT('Ctrl Pts',(9.84148552034242,-4.8,83.4891475666002));
#36064=CARTESIAN_POINT('Ctrl Pts',(9.83090202589081,-4.8,83.4697585577767));
#36065=CARTESIAN_POINT('Ctrl Pts',(9.8207802730647,-4.8,83.4505382257358));
#36066=CARTESIAN_POINT('Ctrl Pts',(9.81112800822446,-4.8,83.431494196779));
#36067=CARTESIAN_POINT('Ctrl Pts',(9.8005726990786,-4.8,83.4106684510759));
#36068=CARTESIAN_POINT('Ctrl Pts',(9.79057804807715,-4.8,83.3900495098162));
#36069=CARTESIAN_POINT('Ctrl Pts',(9.78114500527958,-4.8,83.3695974248259));
#36070=CARTESIAN_POINT('Ctrl Pts',(9.77414463034711,-4.8,83.3544196856643));
#36071=CARTESIAN_POINT('Ctrl Pts',(9.76745315339273,-4.8,83.3393317194716));
#36072=CARTESIAN_POINT('Ctrl Pts',(9.7610752976329,-4.8,83.3243381993367));
#36073=CARTESIAN_POINT('Ctrl Pts',(9.75524656418418,-4.8,83.3106355952616));
#36074=CARTESIAN_POINT('Ctrl Pts',(9.74967957602566,-4.8,83.2970108142608));
#36075=CARTESIAN_POINT('Ctrl Pts',(9.74438544080102,-4.8,83.2835055538423));
#36076=CARTESIAN_POINT('Ctrl Pts',(9.73901880027901,-4.8,83.2698153334857));
#36077=CARTESIAN_POINT('Ctrl Pts',(9.73393247707929,-4.8,83.2562475265611));
#36078=CARTESIAN_POINT('Ctrl Pts',(9.72914861293952,-4.8,83.2429004637275));
#36079=CARTESIAN_POINT('Ctrl Pts',(9.7224876861611,-4.8,83.224316364003));
#36080=CARTESIAN_POINT('Ctrl Pts',(9.71641407457747,-4.8,83.2061640494016));
#36081=CARTESIAN_POINT('Ctrl Pts',(9.71100427501583,-4.8,83.1888039826073));
#36082=CARTESIAN_POINT('Ctrl Pts',(9.7069469253446,-4.8,83.1757839325116));
#36083=CARTESIAN_POINT('Ctrl Pts',(9.70326368266569,-4.8,83.1632132525234));
#36084=CARTESIAN_POINT('Ctrl Pts',(9.69998183250857,-4.8,83.1512267569901));
#36085=CARTESIAN_POINT('Ctrl Pts',(9.69681178844634,-4.8,83.1396486174734));
#36086=CARTESIAN_POINT('Ctrl Pts',(9.69401644626419,-4.8,83.1286165766646));
#36087=CARTESIAN_POINT('Ctrl Pts',(9.69160818908845,-4.8,83.1181991739405));
#36088=CARTESIAN_POINT('Ctrl Pts',(9.68884565180793,-4.8,83.1062492610819));
#36089=CARTESIAN_POINT('Ctrl Pts',(9.68659209322686,-4.8,83.0951069927227));
#36090=CARTESIAN_POINT('Ctrl Pts',(9.68485068856013,-4.8,83.0848030303271));
#36091=CARTESIAN_POINT('Ctrl Pts',(9.68339530889577,-4.8,83.0761914895294));
#36092=CARTESIAN_POINT('Ctrl Pts',(9.68229713919365,-4.8,83.0681632429366));
#36093=CARTESIAN_POINT('Ctrl Pts',(9.68155544397255,-4.8,83.0607187762934));
#36094=CARTESIAN_POINT('',(9.70610859527519,-4.8,82.6330980974667));
#36095=CARTESIAN_POINT('',(9.82575589679681,-4.8,80.5493060959508));
#36096=CARTESIAN_POINT('',(8.91389140472481,-4.8,82.6330980974667));
#36097=CARTESIAN_POINT('Origin',(9.31,-4.8,78.0000000000002));
#36098=CARTESIAN_POINT('',(8.93844455602746,-4.8,83.0607187762934));
#36099=CARTESIAN_POINT('',(8.78196752755185,-4.8,80.3354957565374));
#36100=CARTESIAN_POINT('',(8.46441588009367,-4.8,83.9401167914581));
#36101=CARTESIAN_POINT('Ctrl Pts',(8.93844455602746,-4.8,83.0607187762934));
#36102=CARTESIAN_POINT('Ctrl Pts',(8.93405450203344,-4.8,83.1047821724661));
#36103=CARTESIAN_POINT('Ctrl Pts',(8.91785153528776,-4.8,83.1626590275444));
#36104=CARTESIAN_POINT('Ctrl Pts',(8.85769219190737,-4.8,83.3444846720947));
#36105=CARTESIAN_POINT('Ctrl Pts',(8.79081812423295,-4.8,83.476853030494));
#36106=CARTESIAN_POINT('Ctrl Pts',(8.64267547983925,-4.8,83.7144144641847));
#36107=CARTESIAN_POINT('Ctrl Pts',(8.56318179159508,-4.8,83.823899586071));
#36108=CARTESIAN_POINT('Ctrl Pts',(8.46441588009366,-4.8,83.9401167914581));
#36109=CARTESIAN_POINT('',(8.07294956130202,-4.8,83.871090717415));
#36110=CARTESIAN_POINT('Origin',(9.31,-4.8,78.));
#36111=CARTESIAN_POINT('',(7.92828014771505,-4.8,82.8825995361566));
#36112=CARTESIAN_POINT('Ctrl Pts',(8.07294956130203,-4.8,83.871090717415));
#36113=CARTESIAN_POINT('Ctrl Pts',(8.05456476823445,-4.8,83.8215474908588));
#36114=CARTESIAN_POINT('Ctrl Pts',(8.03769662195923,-4.8,83.772524271155));
#36115=CARTESIAN_POINT('Ctrl Pts',(8.02240062066062,-4.8,83.7240516819751));
#36116=CARTESIAN_POINT('Ctrl Pts',(8.01017493288046,-4.8,83.6853088282291));
#36117=CARTESIAN_POINT('Ctrl Pts',(7.99895428802889,-4.8,83.6469154219601));
#36118=CARTESIAN_POINT('Ctrl Pts',(7.9887476820989,-4.8,83.6089036321699));
#36119=CARTESIAN_POINT('Ctrl Pts',(7.98057168151374,-4.8,83.5784542920367));
#36120=CARTESIAN_POINT('Ctrl Pts',(7.97304588574899,-4.8,83.548248833292));
#36121=CARTESIAN_POINT('Ctrl Pts',(7.96616649805019,-4.8,83.5183408501214));
#36122=CARTESIAN_POINT('Ctrl Pts',(7.95865540215379,-4.8,83.4856865297811));
#36123=CARTESIAN_POINT('Ctrl Pts',(7.95191473077081,-4.8,83.4533858653268));
#36124=CARTESIAN_POINT('Ctrl Pts',(7.94593089663239,-4.8,83.4215841524714));
#36125=CARTESIAN_POINT('Ctrl Pts',(7.94072921137237,-4.8,83.3939392516977));
#36126=CARTESIAN_POINT('Ctrl Pts',(7.93609854851438,-4.8,83.366677578063));
#36127=CARTESIAN_POINT('Ctrl Pts',(7.93203398466726,-4.8,83.3398902206079));
#36128=CARTESIAN_POINT('Ctrl Pts',(7.92872018455444,-4.8,83.3180507437302));
#36129=CARTESIAN_POINT('Ctrl Pts',(7.92578258878329,-4.8,83.2965276961172));
#36130=CARTESIAN_POINT('Ctrl Pts',(7.92322586820198,-4.8,83.2753308935615));
#36131=CARTESIAN_POINT('Ctrl Pts',(7.92042994648818,-4.8,83.2521509649602));
#36132=CARTESIAN_POINT('Ctrl Pts',(7.91809013983445,-4.8,83.2293571253706));
#36133=CARTESIAN_POINT('Ctrl Pts',(7.91622100408708,-4.8,83.2069121607238));
#36134=CARTESIAN_POINT('Ctrl Pts',(7.91483389591844,-4.8,83.1902554819084));
#36135=CARTESIAN_POINT('Ctrl Pts',(7.91370635273902,-4.8,83.1737888114215));
#36136=CARTESIAN_POINT('Ctrl Pts',(7.91284121463069,-4.8,83.1575181559638));
#36137=CARTESIAN_POINT('Ctrl Pts',(7.91205056341829,-4.8,83.1426483758209));
#36138=CARTESIAN_POINT('Ctrl Pts',(7.91147925526362,-4.8,83.1279412476054));
#36139=CARTESIAN_POINT('Ctrl Pts',(7.91112346655007,-4.8,83.1134397531939));
#36140=CARTESIAN_POINT('Ctrl Pts',(7.91076280516985,-4.8,83.0987396551006));
#36141=CARTESIAN_POINT('Ctrl Pts',(7.91062368804623,-4.8,83.0842504621696));
#36142=CARTESIAN_POINT('Ctrl Pts',(7.91069329054054,-4.8,83.0700721479122));
#36143=CARTESIAN_POINT('Ctrl Pts',(7.91079020322715,-4.8,83.0503306351971));
#36144=CARTESIAN_POINT('Ctrl Pts',(7.91129133246646,-4.8,83.0311957414029));
#36145=CARTESIAN_POINT('Ctrl Pts',(7.91214527626044,-4.8,83.0130323541204));
#36146=CARTESIAN_POINT('Ctrl Pts',(7.91278573410593,-4.8,82.9994098136585));
#36147=CARTESIAN_POINT('Ctrl Pts',(7.91362404390535,-4.8,82.9863374951043));
#36148=CARTESIAN_POINT('Ctrl Pts',(7.91463973644661,-4.8,82.9739514147098));
#36149=CARTESIAN_POINT('Ctrl Pts',(7.91562082635049,-4.8,82.9619873035935));
#36150=CARTESIAN_POINT('Ctrl Pts',(7.91676724408405,-4.8,82.9506645129822));
#36151=CARTESIAN_POINT('Ctrl Pts',(7.91806718413429,-4.8,82.9400516840982));
#36152=CARTESIAN_POINT('Ctrl Pts',(7.91955835913016,-4.8,82.9278775957128));
#36153=CARTESIAN_POINT('Ctrl Pts',(7.9212515869683,-4.8,82.9166365258692));
#36154=CARTESIAN_POINT('Ctrl Pts',(7.92313936453975,-4.8,82.9063583729027));
#36155=CARTESIAN_POINT('Ctrl Pts',(7.92471707547372,-4.8,82.8977684020495));
#36156=CARTESIAN_POINT('Ctrl Pts',(7.92643095561883,-4.8,82.8898487215006));
#36157=CARTESIAN_POINT('Ctrl Pts',(7.92828014771505,-4.8,82.8825995361566));
#36158=CARTESIAN_POINT('',(8.09760744867255,-4.8,82.4891652120952));
#36159=CARTESIAN_POINT('',(8.92273797402872,-4.8,80.571963032233));
#36160=CARTESIAN_POINT('',(7.3531668006526,-4.8,82.2182109750381));
#36161=CARTESIAN_POINT('Origin',(9.31000000000056,-4.8,77.9999999999986));
#36162=CARTESIAN_POINT('',(7.22998432988738,-4.8,82.6284406437547));
#36163=CARTESIAN_POINT('',(8.01502518871776,-4.8,80.0140503863876));
#36164=CARTESIAN_POINT('',(6.48377124583839,-4.8,83.2926771136307));
#36165=CARTESIAN_POINT('Ctrl Pts',(7.22998432988738,-4.8,82.6284406437547));
#36166=CARTESIAN_POINT('Ctrl Pts',(7.21078845977609,-4.8,82.6683452043475));
#36167=CARTESIAN_POINT('Ctrl Pts',(7.17576760202974,-4.8,82.7171899164891));
#36168=CARTESIAN_POINT('Ctrl Pts',(7.0570482750219,-4.8,82.867474428743));
#36169=CARTESIAN_POINT('Ctrl Pts',(6.94893456238546,-4.8,82.9689877197435));
#36170=CARTESIAN_POINT('Ctrl Pts',(6.72847521688295,-4.8,83.1415546773667));
#36171=CARTESIAN_POINT('Ctrl Pts',(6.61632946835478,-4.8,83.21724859508));
#36172=CARTESIAN_POINT('Ctrl Pts',(6.48377124583839,-4.8,83.2926771136307));
#36173=CARTESIAN_POINT('',(6.13952154251532,-4.8,83.0939244547427));
#36174=CARTESIAN_POINT('Origin',(9.31,-4.8,78.));
#36175=CARTESIAN_POINT('',(6.34166065765632,-4.8,82.1155667324646));
#36176=CARTESIAN_POINT('Ctrl Pts',(6.13952154251532,-4.8,83.0939244547427));
#36177=CARTESIAN_POINT('Ctrl Pts',(6.13919026958859,-4.8,83.0410810807779));
#36178=CARTESIAN_POINT('Ctrl Pts',(6.14010632566913,-4.8,82.9892450771334));
#36179=CARTESIAN_POINT('Ctrl Pts',(6.14231138803794,-4.8,82.9384642021974));
#36180=CARTESIAN_POINT('Ctrl Pts',(6.144073836074,-4.8,82.8978763918177));
#36181=CARTESIAN_POINT('Ctrl Pts',(6.14666119765675,-4.8,82.8579606997597));
#36182=CARTESIAN_POINT('Ctrl Pts',(6.15007092380639,-4.8,82.8187504318208));
#36183=CARTESIAN_POINT('Ctrl Pts',(6.15280228412168,-4.8,82.7873410560821));
#36184=CARTESIAN_POINT('Ctrl Pts',(6.15606122471426,-4.8,82.7563832370041));
#36185=CARTESIAN_POINT('Ctrl Pts',(6.15982584751516,-4.8,82.7259260380751));
#36186=CARTESIAN_POINT('Ctrl Pts',(6.16393616160808,-4.8,82.6926720679937));
#36187=CARTESIAN_POINT('Ctrl Pts',(6.16864948050054,-4.8,82.6600139264594));
#36188=CARTESIAN_POINT('Ctrl Pts',(6.17390334227212,-4.8,82.62808349967));
#36189=CARTESIAN_POINT('Ctrl Pts',(6.17847046997489,-4.8,82.6003267098853));
#36190=CARTESIAN_POINT('Ctrl Pts',(6.18344311179598,-4.8,82.5731253369718));
#36191=CARTESIAN_POINT('Ctrl Pts',(6.18878548697729,-4.8,82.5465632927227));
#36192=CARTESIAN_POINT('Ctrl Pts',(6.19314107449476,-4.8,82.5249075114561));
#36193=CARTESIAN_POINT('Ctrl Pts',(6.19774195326573,-4.8,82.5036777458914));
#36194=CARTESIAN_POINT('Ctrl Pts',(6.20258915525585,-4.8,82.4828848173746));
#36195=CARTESIAN_POINT('Ctrl Pts',(6.20788985046534,-4.8,82.4601465496472));
#36196=CARTESIAN_POINT('Ctrl Pts',(6.21348710337351,-4.8,82.4379270873797));
#36197=CARTESIAN_POINT('Ctrl Pts',(6.21940731995865,-4.8,82.4161964391848));
#36198=CARTESIAN_POINT('Ctrl Pts',(6.22380078431013,-4.8,82.4000698622588));
#36199=CARTESIAN_POINT('Ctrl Pts',(6.22837317328842,-4.8,82.3842106112069));
#36200=CARTESIAN_POINT('Ctrl Pts',(6.23312510128403,-4.8,82.3686253018486));
#36201=CARTESIAN_POINT('Ctrl Pts',(6.23746789652353,-4.8,82.3543818605864));
#36202=CARTESIAN_POINT('Ctrl Pts',(6.24196117657975,-4.8,82.3403662818851));
#36203=CARTESIAN_POINT('Ctrl Pts',(6.24658664775933,-4.8,82.3266176477455));
#36204=CARTESIAN_POINT('Ctrl Pts',(6.25127546664344,-4.8,82.312680720483));
#36205=CARTESIAN_POINT('Ctrl Pts',(6.25610033521784,-4.8,82.2990177518533));
#36206=CARTESIAN_POINT('Ctrl Pts',(6.2610150093059,-4.8,82.2857182999482));
#36207=CARTESIAN_POINT('Ctrl Pts',(6.26785807237896,-4.8,82.2672004925425));
#36208=CARTESIAN_POINT('Ctrl Pts',(6.27487349885991,-4.8,82.2493909706609));
#36209=CARTESIAN_POINT('Ctrl Pts',(6.28188818776893,-4.8,82.232615035949));
#36210=CARTESIAN_POINT('Ctrl Pts',(6.28714920445069,-4.8,82.220033084915));
#36211=CARTESIAN_POINT('Ctrl Pts',(6.29240795417291,-4.8,82.2080358426923));
#36212=CARTESIAN_POINT('Ctrl Pts',(6.29759868187373,-4.8,82.19674412186));
#36213=CARTESIAN_POINT('Ctrl Pts',(6.30261257180666,-4.8,82.185837087496));
#36214=CARTESIAN_POINT('Ctrl Pts',(6.30756247454736,-4.8,82.1755892427291));
#36215=CARTESIAN_POINT('Ctrl Pts',(6.3124138198641,-4.8,82.1660610514844));
#36216=CARTESIAN_POINT('Ctrl Pts',(6.31797884951121,-4.8,82.1551311622892));
#36217=CARTESIAN_POINT('Ctrl Pts',(6.32341463558439,-4.8,82.1451471298991));
#36218=CARTESIAN_POINT('Ctrl Pts',(6.32870390163747,-4.8,82.1361344833445));
#36219=CARTESIAN_POINT('Ctrl Pts',(6.33312440775988,-4.8,82.128602160547));
#36220=CARTESIAN_POINT('Ctrl Pts',(6.33744361831287,-4.8,82.1217462771392));
#36221=CARTESIAN_POINT('Ctrl Pts',(6.34166065765632,-4.8,82.1155667324646));
#36222=CARTESIAN_POINT('',(6.63533873676839,-4.8,81.8037727491227));
#36223=CARTESIAN_POINT('',(8.06642956697154,-4.8,80.2844032686962));
#36224=CARTESIAN_POINT('',(6.02846516020393,-4.8,81.2945453548562));
#36225=CARTESIAN_POINT('Origin',(9.3100000000004,-4.8,77.9999999999995));
#36226=CARTESIAN_POINT('',(5.77240469132478,-4.8,81.6379042610703));
#36227=CARTESIAN_POINT('',(7.40427592391703,-4.8,79.4496808154216));
#36228=CARTESIAN_POINT('',(4.8440115100785,-4.8,82.006862464309));
#36229=CARTESIAN_POINT('Ctrl Pts',(5.77240469132478,-4.8,81.6379042610703));
#36230=CARTESIAN_POINT('Ctrl Pts',(5.74071830812517,-4.8,81.6688369101196));
#36231=CARTESIAN_POINT('Ctrl Pts',(5.69110358768174,-4.8,81.7027580880799));
#36232=CARTESIAN_POINT('Ctrl Pts',(5.52814358921249,-4.8,81.8033749296924));
#36233=CARTESIAN_POINT('Ctrl Pts',(5.39183034107398,-4.8,81.8617891528896));
#36234=CARTESIAN_POINT('Ctrl Pts',(5.12564494391121,-4.8,81.9485475132162));
#36235=CARTESIAN_POINT('Ctrl Pts',(4.99437356661556,-4.8,81.9813204242451));
#36236=CARTESIAN_POINT('Ctrl Pts',(4.8440115100785,-4.8,82.006862464309));
#36237=CARTESIAN_POINT('',(4.58850001701745,-4.8,81.7023557244943));
#36238=CARTESIAN_POINT('Origin',(9.31,-4.8,78.));
#36239=CARTESIAN_POINT('',(5.11306670030725,-4.8,80.8521358415414));
#36240=CARTESIAN_POINT('Ctrl Pts',(4.58850001701745,-4.8,81.7023557244943));
#36241=CARTESIAN_POINT('Ctrl Pts',(4.60626222063291,-4.8,81.6525858939099));
#36242=CARTESIAN_POINT('Ctrl Pts',(4.62485198918894,-4.8,81.6041892934237));
#36243=CARTESIAN_POINT('Ctrl Pts',(4.6442921521603,-4.8,81.5572250557159));
#36244=CARTESIAN_POINT('Ctrl Pts',(4.65983016136228,-4.8,81.5196877799871));
#36245=CARTESIAN_POINT('Ctrl Pts',(4.67591345780073,-4.8,81.4830642260602));
#36246=CARTESIAN_POINT('Ctrl Pts',(4.69252825496127,-4.8,81.4473848193518));
#36247=CARTESIAN_POINT('Ctrl Pts',(4.70583753319529,-4.8,81.4188038414128));
#36248=CARTESIAN_POINT('Ctrl Pts',(4.71948813323713,-4.8,81.3908276310071));
#36249=CARTESIAN_POINT('Ctrl Pts',(4.73344269693336,-4.8,81.3634948031522));
#36250=CARTESIAN_POINT('Ctrl Pts',(4.74867865634235,-4.8,81.3336521033162));
#36251=CARTESIAN_POINT('Ctrl Pts',(4.76427746953913,-4.8,81.3045755389547));
#36252=CARTESIAN_POINT('Ctrl Pts',(4.78013533378095,-4.8,81.2763676793213));
#36253=CARTESIAN_POINT('Ctrl Pts',(4.79392041110474,-4.8,81.2518468787736));
#36254=CARTESIAN_POINT('Ctrl Pts',(4.8078965832873,-4.8,81.2279866933517));
#36255=CARTESIAN_POINT('Ctrl Pts',(4.82200152789346,-4.8,81.2048537366049));
#36256=CARTESIAN_POINT('Ctrl Pts',(4.8335011546974,-4.8,81.1859936576122));
#36257=CARTESIAN_POINT('Ctrl Pts',(4.84508557392789,-4.8,81.1676177969763));
#36258=CARTESIAN_POINT('Ctrl Pts',(4.85675205419961,-4.8,81.1497366763869));
#36259=CARTESIAN_POINT('Ctrl Pts',(4.86951002346223,-4.8,81.1301826393895));
#36260=CARTESIAN_POINT('Ctrl Pts',(4.88236922388144,-4.8,81.1112175487126));
#36261=CARTESIAN_POINT('Ctrl Pts',(4.89536472661568,-4.8,81.0928222530497));
#36262=CARTESIAN_POINT('Ctrl Pts',(4.90500884676139,-4.8,81.0791708811008));
#36263=CARTESIAN_POINT('Ctrl Pts',(4.91472967022465,-4.8,81.0658319091268));
#36264=CARTESIAN_POINT('Ctrl Pts',(4.92452551159968,-4.8,81.0528117640994));
#36265=CARTESIAN_POINT('Ctrl Pts',(4.93347794805258,-4.8,81.0409126309364));
#36266=CARTESIAN_POINT('Ctrl Pts',(4.94249386039137,-4.8,81.0292790873789));
#36267=CARTESIAN_POINT('Ctrl Pts',(4.95154269133482,-4.8,81.0179416016839));
#36268=CARTESIAN_POINT('Ctrl Pts',(4.96071544974391,-4.8,81.0064488444541));
#36269=CARTESIAN_POINT('Ctrl Pts',(4.96992235367127,-4.8,80.9952600558691));
#36270=CARTESIAN_POINT('Ctrl Pts',(4.97908931713115,-4.8,80.9844435765684));
#36271=CARTESIAN_POINT('Ctrl Pts',(4.99185315606398,-4.8,80.9693829951428));
#36272=CARTESIAN_POINT('Ctrl Pts',(5.00453671569697,-4.8,80.9550469361515));
#36273=CARTESIAN_POINT('Ctrl Pts',(5.01686607460425,-4.8,80.9416818791236));
#36274=CARTESIAN_POINT('Ctrl Pts',(5.02611309378471,-4.8,80.9316580863527));
#36275=CARTESIAN_POINT('Ctrl Pts',(5.03515800052709,-4.8,80.9221829647861));
#36276=CARTESIAN_POINT('Ctrl Pts',(5.04389768495218,-4.8,80.913347551555));
#36277=CARTESIAN_POINT('Ctrl Pts',(5.05233962579543,-4.8,80.9048131431948));
#36278=CARTESIAN_POINT('Ctrl Pts',(5.06049598222156,-4.8,80.8968762855306));
#36279=CARTESIAN_POINT('Ctrl Pts',(5.06831358896028,-4.8,80.8895819723517));
#36280=CARTESIAN_POINT('Ctrl Pts',(5.07728124855712,-4.8,80.8812145883469));
#36281=CARTESIAN_POINT('Ctrl Pts',(5.08580395683557,-4.8,80.8736918151081));
#36282=CARTESIAN_POINT('Ctrl Pts',(5.09385674780709,-4.8,80.8670317331858));
#36283=CARTESIAN_POINT('Ctrl Pts',(5.10058687068216,-4.8,80.8614655673864));
#36284=CARTESIAN_POINT('Ctrl Pts',(5.10699045098391,-4.8,80.8565004015291));
#36285=CARTESIAN_POINT('Ctrl Pts',(5.11306670030725,-4.8,80.8521358415414));
#36286=CARTESIAN_POINT('',(5.49567364700612,-4.8,80.659589154899));
#36287=CARTESIAN_POINT('',(7.36011410728251,-4.8,79.721310756753));
#36288=CARTESIAN_POINT('',(5.09956505173093,-4.8,79.9735089425676));
#36289=CARTESIAN_POINT('Origin',(9.30999999999911,-4.8,78.0000000000005));
#36290=CARTESIAN_POINT('',(4.7415112563347,-4.8,80.2085829347521));
#36291=CARTESIAN_POINT('',(7.02338510818378,-4.8,78.7104583431054));
#36292=CARTESIAN_POINT('',(3.74291589718234,-4.8,80.2377610668154));
#36293=CARTESIAN_POINT('Ctrl Pts',(4.7415112563347,-4.8,80.2085829347521));
#36294=CARTESIAN_POINT('Ctrl Pts',(4.7011562116549,-4.8,80.2268127331602));
#36295=CARTESIAN_POINT('Ctrl Pts',(4.6429319051249,-4.8,80.2417189802796));
#36296=CARTESIAN_POINT('Ctrl Pts',(4.45538659248291,-4.8,80.2805322845508));
#36297=CARTESIAN_POINT('Ctrl Pts',(4.30731519855239,-4.8,80.2888018217475));
#36298=CARTESIAN_POINT('Ctrl Pts',(4.02750964186796,-4.8,80.2792872446601));
#36299=CARTESIAN_POINT('Ctrl Pts',(3.89294590272478,-4.8,80.2651862520695));
#36300=CARTESIAN_POINT('Ctrl Pts',(3.74291589718234,-4.8,80.2377610668154));
#36301=CARTESIAN_POINT('',(3.60696107140887,-4.8,79.8642282529171));
#36302=CARTESIAN_POINT('Origin',(9.31,-4.8,78.));
#36303=CARTESIAN_POINT('',(4.39068483903982,-4.8,79.2446952750862));
#36304=CARTESIAN_POINT('Ctrl Pts',(3.60696107140887,-4.8,79.8642282529171));
#36305=CARTESIAN_POINT('Ctrl Pts',(3.64067436766681,-4.8,79.8235349418069));
#36306=CARTESIAN_POINT('Ctrl Pts',(3.67469564825235,-4.8,79.7844150887646));
#36307=CARTESIAN_POINT('Ctrl Pts',(3.70902614126382,-4.8,79.7469320684765));
#36308=CARTESIAN_POINT('Ctrl Pts',(3.73646559938461,-4.8,79.7169728784033));
#36309=CARTESIAN_POINT('Ctrl Pts',(3.76410494864752,-4.8,79.6880588052678));
#36310=CARTESIAN_POINT('Ctrl Pts',(3.79192082785855,-4.8,79.6602137243463));
#36311=CARTESIAN_POINT('Ctrl Pts',(3.81420272833821,-4.8,79.6379084318465));
#36312=CARTESIAN_POINT('Ctrl Pts',(3.83659852371768,-4.8,79.6162881738544));
#36313=CARTESIAN_POINT('Ctrl Pts',(3.85905990170427,-4.8,79.5953764593762));
#36314=CARTESIAN_POINT('Ctrl Pts',(3.88358382496445,-4.8,79.5725444994933));
#36315=CARTESIAN_POINT('Ctrl Pts',(3.90818668548508,-4.8,79.5505565747794));
#36316=CARTESIAN_POINT('Ctrl Pts',(3.93273585983976,-4.8,79.5294735661781));
#36317=CARTESIAN_POINT('Ctrl Pts',(3.95407620286161,-4.8,79.5111463251481));
#36318=CARTESIAN_POINT('Ctrl Pts',(3.97537017262871,-4.8,79.4935052175616));
#36319=CARTESIAN_POINT('Ctrl Pts',(3.99653642203519,-4.8,79.47659152415));
#36320=CARTESIAN_POINT('Ctrl Pts',(4.01379306328134,-4.8,79.4628019512433));
#36321=CARTESIAN_POINT('Ctrl Pts',(4.03096377091259,-4.8,79.4494963954657));
#36322=CARTESIAN_POINT('Ctrl Pts',(4.04804237963872,-4.8,79.4366838097816));
#36323=CARTESIAN_POINT('Ctrl Pts',(4.0667188232732,-4.8,79.4226725083823));
#36324=CARTESIAN_POINT('Ctrl Pts',(4.08528896157969,-4.8,79.4092492585601));
#36325=CARTESIAN_POINT('Ctrl Pts',(4.10379230079774,-4.8,79.3964080590159));
#36326=CARTESIAN_POINT('Ctrl Pts',(4.11752385348229,-4.8,79.3868784489279));
#36327=CARTESIAN_POINT('Ctrl Pts',(4.13122063662477,-4.8,79.377668632869));
#36328=CARTESIAN_POINT('Ctrl Pts',(4.14487886830775,-4.8,79.3687840737741));
#36329=CARTESIAN_POINT('Ctrl Pts',(4.15736114997002,-4.8,79.3606644597829));
#36330=CARTESIAN_POINT('Ctrl Pts',(4.1698122424592,-4.8,79.3528161284141));
#36331=CARTESIAN_POINT('Ctrl Pts',(4.18219301056543,-4.8,79.3452572592584));
#36332=CARTESIAN_POINT('Ctrl Pts',(4.19474333843089,-4.8,79.3375948682515));
#36333=CARTESIAN_POINT('Ctrl Pts',(4.20722178918766,-4.8,79.3302297927924));
#36334=CARTESIAN_POINT('Ctrl Pts',(4.21953537090469,-4.8,79.3232009131774));
#36335=CARTESIAN_POINT('Ctrl Pts',(4.2366804783172,-4.8,79.3134140860169));
#36336=CARTESIAN_POINT('Ctrl Pts',(4.25350234659464,-4.8,79.3042806301018));
#36337=CARTESIAN_POINT('Ctrl Pts',(4.26965927283183,-4.8,79.2959384737804));
#36338=CARTESIAN_POINT('Ctrl Pts',(4.28177696750972,-4.8,79.2896818565394));
#36339=CARTESIAN_POINT('Ctrl Pts',(4.29351708201629,-4.8,79.2838716950536));
#36340=CARTESIAN_POINT('Ctrl Pts',(4.30475158822826,-4.8,79.2785582705871));
#36341=CARTESIAN_POINT('Ctrl Pts',(4.31560335725497,-4.8,79.2734258638783));
#36342=CARTESIAN_POINT('Ctrl Pts',(4.32598239033975,-4.8,79.2687572955227));
#36343=CARTESIAN_POINT('Ctrl Pts',(4.33582333969107,-4.8,79.2645766622574));
#36344=CARTESIAN_POINT('Ctrl Pts',(4.34711199719151,-4.8,79.2597810134453));
#36345=CARTESIAN_POINT('Ctrl Pts',(4.35769366331604,-4.8,79.2556268568332));
#36346=CARTESIAN_POINT('Ctrl Pts',(4.36753869379978,-4.8,79.2521226437087));
#36347=CARTESIAN_POINT('Ctrl Pts',(4.3757666812864,-4.8,79.2491939964296));
#36348=CARTESIAN_POINT('Ctrl Pts',(4.38348226505871,-4.8,79.246718420208));
#36349=CARTESIAN_POINT('Ctrl Pts',(4.39068483903982,-4.8,79.2446952750862));
#36350=CARTESIAN_POINT('',(4.81607260887647,-4.8,79.194619857239));
#36351=CARTESIAN_POINT('',(6.88898366350615,-4.8,78.9506027637043));
#36352=CARTESIAN_POINT('',(4.67850553742098,-4.8,78.4144382259154));
#36353=CARTESIAN_POINT('Origin',(9.31000000000016,-4.8,78.));
#36354=CARTESIAN_POINT('',(6.91829379524532,-4.8,77.8855441093625));
#36355=CARTESIAN_POINT('Origin',(9.31,-9.325,78.));
#36356=CARTESIAN_POINT('',(3.06,-13.85,78.));
#36357=CARTESIAN_POINT('Origin',(9.31,-13.85,78.));
#36358=CARTESIAN_POINT('',(3.06,-9.325,78.));
#36359=CARTESIAN_POINT('Origin',(9.31,4.875,78.));
#36360=CARTESIAN_POINT('',(15.41,4.8,78.));
#36361=CARTESIAN_POINT('Origin',(9.31,4.8,78.));
#36362=CARTESIAN_POINT('',(15.56,4.95,78.));
#36363=CARTESIAN_POINT('',(15.485,4.875,78.));
#36364=CARTESIAN_POINT('',(3.06,4.95,78.));
#36365=CARTESIAN_POINT('Origin',(9.31,4.95,78.));
#36366=CARTESIAN_POINT('Origin',(9.31,4.95,78.));
#36367=CARTESIAN_POINT('Origin',(9.31,4.8,78.));
#36368=CARTESIAN_POINT('',(3.31329278848646,4.8,78.1987526588035));
#36369=CARTESIAN_POINT('',(4.2616449875437,4.8,78.5128739112901));
#36370=CARTESIAN_POINT('Ctrl Pts',(3.31329278848646,4.8,78.1987526588035));
#36371=CARTESIAN_POINT('Ctrl Pts',(3.35889085630227,4.8,78.2254612365697));
#36372=CARTESIAN_POINT('Ctrl Pts',(3.40424018037907,4.8,78.2505859106759));
#36373=CARTESIAN_POINT('Ctrl Pts',(3.44932023930959,4.8,78.2740667081797));
#36374=CARTESIAN_POINT('Ctrl Pts',(3.48535154078234,4.8,78.2928342899832));
#36375=CARTESIAN_POINT('Ctrl Pts',(3.52121322744871,4.8,78.3105514163533));
#36376=CARTESIAN_POINT('Ctrl Pts',(3.55687518114691,4.8,78.3272036418769));
#36377=CARTESIAN_POINT('Ctrl Pts',(3.58544217793619,4.8,78.3405429018931));
#36378=CARTESIAN_POINT('Ctrl Pts',(3.61388190532127,4.8,78.3531994856718));
#36379=CARTESIAN_POINT('Ctrl Pts',(3.64214092404874,4.8,78.3651678257731));
#36380=CARTESIAN_POINT('Ctrl Pts',(3.67299486093853,4.8,78.3782351730056));
#36381=CARTESIAN_POINT('Ctrl Pts',(3.70363429760745,4.8,78.3904823886558));
#36382=CARTESIAN_POINT('Ctrl Pts',(3.73391378633966,4.8,78.4018976232415));
#36383=CARTESIAN_POINT('Ctrl Pts',(3.7602354354294,4.8,78.4118207696229));
#36384=CARTESIAN_POINT('Ctrl Pts',(3.7862788364629,4.8,78.4211150220416));
#36385=CARTESIAN_POINT('Ctrl Pts',(3.81195342930972,4.8,78.4297694116381));
#36386=CARTESIAN_POINT('Ctrl Pts',(3.83288567961382,4.8,78.4368252528094));
#36387=CARTESIAN_POINT('Ctrl Pts',(3.85357163513014,4.8,78.4434556576798));
#36388=CARTESIAN_POINT('Ctrl Pts',(3.87400244027753,4.8,78.449654321866));
#36389=CARTESIAN_POINT('Ctrl Pts',(3.89634470605425,4.8,78.4564329192688));
#36390=CARTESIAN_POINT('Ctrl Pts',(3.91838595195131,4.8,78.4626952874073));
#36391=CARTESIAN_POINT('Ctrl Pts',(3.94016535426666,4.8,78.468433553731));
#36392=CARTESIAN_POINT('Ctrl Pts',(3.95632811179584,4.8,78.4726919904816));
#36393=CARTESIAN_POINT('Ctrl Pts',(3.97234882063946,4.8,78.4766618110219));
#36394=CARTESIAN_POINT('Ctrl Pts',(3.98822205852683,4.8,78.4803391753661));
#36395=CARTESIAN_POINT('Ctrl Pts',(4.00272863804244,4.8,78.4836999249904));
#36396=CARTESIAN_POINT('Ctrl Pts',(4.01711312520302,4.8,78.4868164196652));
#36397=CARTESIAN_POINT('Ctrl Pts',(4.03133252715836,4.8,78.4896849611932));
#36398=CARTESIAN_POINT('Ctrl Pts',(4.04574666952095,4.8,78.4925927885468));
#36399=CARTESIAN_POINT('Ctrl Pts',(4.05999158159986,4.8,78.4952458141038));
#36400=CARTESIAN_POINT('Ctrl Pts',(4.073966581728,4.8,78.4976393074474));
#36401=CARTESIAN_POINT('Ctrl Pts',(4.09342500507885,4.8,78.5009719447526));
#36402=CARTESIAN_POINT('Ctrl Pts',(4.11235621687838,4.8,78.5038011681971));
#36403=CARTESIAN_POINT('Ctrl Pts',(4.13039194713631,4.8,78.5061142367954));
#36404=CARTESIAN_POINT('Ctrl Pts',(4.14391874482975,4.8,78.5078490382441));
#36405=CARTESIAN_POINT('Ctrl Pts',(4.15693803635337,4.8,78.5092934485219));
#36406=CARTESIAN_POINT('Ctrl Pts',(4.16931231741,4.8,78.510444006894));
#36407=CARTESIAN_POINT('Ctrl Pts',(4.1812650311382,4.8,78.5115553680136));
#36408=CARTESIAN_POINT('Ctrl Pts',(4.19261487634346,4.8,78.512392548869));
#36409=CARTESIAN_POINT('Ctrl Pts',(4.20329220461838,4.8,78.5129552562033));
#36410=CARTESIAN_POINT('Ctrl Pts',(4.21554028124679,4.8,78.513600743761));
#36411=CARTESIAN_POINT('Ctrl Pts',(4.22690460006138,4.8,78.513885231135));
#36412=CARTESIAN_POINT('Ctrl Pts',(4.23735441405482,4.8,78.5138109156641));
#36413=CARTESIAN_POINT('Ctrl Pts',(4.24608785027474,4.8,78.5137488064796));
#36414=CARTESIAN_POINT('Ctrl Pts',(4.25418482498679,4.8,78.5134362021356));
#36415=CARTESIAN_POINT('Ctrl Pts',(4.2616449875437,4.8,78.5128739112901));
#36416=CARTESIAN_POINT('',(4.67850553742098,4.8,78.4144382259154));
#36417=CARTESIAN_POINT('',(6.91829379524532,4.8,77.8855441093625));
#36418=CARTESIAN_POINT('',(4.81607260887647,4.8,79.194619857239));
#36419=CARTESIAN_POINT('Origin',(9.31000000000016,4.8,78.));
#36420=CARTESIAN_POINT('',(4.39068483903982,4.8,79.2446952750862));
#36421=CARTESIAN_POINT('',(6.88898366350615,4.8,78.9506027637043));
#36422=CARTESIAN_POINT('',(3.60696107140888,4.8,79.8642282529171));
#36423=CARTESIAN_POINT('Ctrl Pts',(4.39068483903982,4.8,79.2446952750862));
#36424=CARTESIAN_POINT('Ctrl Pts',(4.34805318204033,4.8,79.256670164774));
#36425=CARTESIAN_POINT('Ctrl Pts',(4.29386921508062,4.8,79.2826771886758));
#36426=CARTESIAN_POINT('Ctrl Pts',(4.12525249151527,4.8,79.3734962560852));
#36427=CARTESIAN_POINT('Ctrl Pts',(4.00650766503333,4.8,79.4623398804252));
#36428=CARTESIAN_POINT('Ctrl Pts',(3.79828002278047,4.8,79.6494840153308));
#36429=CARTESIAN_POINT('Ctrl Pts',(3.70426215728068,4.8,79.7467819098348));
#36430=CARTESIAN_POINT('Ctrl Pts',(3.60696107140887,4.8,79.8642282529171));
#36431=CARTESIAN_POINT('',(3.74291589718233,4.8,80.2377610668154));
#36432=CARTESIAN_POINT('Origin',(9.31,4.8,78.));
#36433=CARTESIAN_POINT('',(4.7415112563347,4.8,80.2085829347521));
#36434=CARTESIAN_POINT('Ctrl Pts',(3.74291589718233,4.8,80.2377610668154));
#36435=CARTESIAN_POINT('Ctrl Pts',(3.79489893662468,4.8,80.2472634625638));
#36436=CARTESIAN_POINT('Ctrl Pts',(3.8461065064291,4.8,80.2553625510896));
#36437=CARTESIAN_POINT('Ctrl Pts',(3.89649881086473,4.8,80.2620089950116));
#36438=CARTESIAN_POINT('Ctrl Pts',(3.93677604781892,4.8,80.2673213219581));
#36439=CARTESIAN_POINT('Ctrl Pts',(3.97653462213701,4.8,80.271704555469));
#36440=CARTESIAN_POINT('Ctrl Pts',(4.01574129138727,4.8,80.275155422314));
#36441=CARTESIAN_POINT('Ctrl Pts',(4.04714778360346,4.8,80.2779197383036));
#36442=CARTESIAN_POINT('Ctrl Pts',(4.07820119267025,4.8,80.280086077154));
#36443=CARTESIAN_POINT('Ctrl Pts',(4.10884939793472,4.8,80.281667484482));
#36444=CARTESIAN_POINT('Ctrl Pts',(4.14231191142195,4.8,80.2833941064353));
#36445=CARTESIAN_POINT('Ctrl Pts',(4.17529235909806,4.8,80.2844234201605));
#36446=CARTESIAN_POINT('Ctrl Pts',(4.20765001204969,4.8,80.2847940368353));
#36447=CARTESIAN_POINT('Ctrl Pts',(4.23577818756272,4.8,80.2851162101058));
#36448=CARTESIAN_POINT('Ctrl Pts',(4.26342980102536,4.8,80.2849425827943));
#36449=CARTESIAN_POINT('Ctrl Pts',(4.29051600217998,4.8,80.2842938209344));
#36450=CARTESIAN_POINT('Ctrl Pts',(4.3125991233526,4.8,80.2837648915846));
#36451=CARTESIAN_POINT('Ctrl Pts',(4.33430529534107,4.8,80.2829204206548));
#36452=CARTESIAN_POINT('Ctrl Pts',(4.3556240403936,4.8,80.2817575127505));
#36453=CARTESIAN_POINT('Ctrl Pts',(4.3789373199094,4.8,80.2804858057641));
#36454=CARTESIAN_POINT('Ctrl Pts',(4.40179117244473,4.8,80.2788319567986));
#36455=CARTESIAN_POINT('Ctrl Pts',(4.42421971910711,4.8,80.2767751689934));
#36456=CARTESIAN_POINT('Ctrl Pts',(4.44086421427025,4.8,80.2752488019402));
#36457=CARTESIAN_POINT('Ctrl Pts',(4.457276514773,4.8,80.2734998078755));
#36458=CARTESIAN_POINT('Ctrl Pts',(4.47345021199511,4.8,80.271526432919));
#36459=CARTESIAN_POINT('Ctrl Pts',(4.48823138184513,4.8,80.2697229621349));
#36460=CARTESIAN_POINT('Ctrl Pts',(4.50281428229542,4.8,80.267731724821));
#36461=CARTESIAN_POINT('Ctrl Pts',(4.51715724842402,4.8,80.2655639502292));
#36462=CARTESIAN_POINT('Ctrl Pts',(4.53169664720218,4.8,80.2633664870985));
#36463=CARTESIAN_POINT('Ctrl Pts',(4.54598987418342,4.8,80.2609874687648));
#36464=CARTESIAN_POINT('Ctrl Pts',(4.5599407016508,4.8,80.2584568852483));
#36465=CARTESIAN_POINT('Ctrl Pts',(4.57936546759993,4.8,80.254933367189));
#36466=CARTESIAN_POINT('Ctrl Pts',(4.59812263906443,4.8,80.2511171118083));
#36467=CARTESIAN_POINT('Ctrl Pts',(4.61586179777949,4.8,80.2471221022498));
#36468=CARTESIAN_POINT('Ctrl Pts',(4.62916616681578,4.8,80.2441258450809));
#36469=CARTESIAN_POINT('Ctrl Pts',(4.64189431642035,4.8,80.2410302868029));
#36470=CARTESIAN_POINT('Ctrl Pts',(4.65391585117796,4.8,80.2378792046286));
#36471=CARTESIAN_POINT('Ctrl Pts',(4.66552783602353,4.8,80.2348354735915));
#36472=CARTESIAN_POINT('Ctrl Pts',(4.67647953458823,4.8,80.2317402905604));
#36473=CARTESIAN_POINT('Ctrl Pts',(4.68670539847485,4.8,80.228617201124));
#36474=CARTESIAN_POINT('Ctrl Pts',(4.69843559535106,4.8,80.2250346721214));
#36475=CARTESIAN_POINT('Ctrl Pts',(4.70921186221142,4.8,80.2214151768855));
#36476=CARTESIAN_POINT('Ctrl Pts',(4.71900605785115,4.8,80.2177712963384));
#36477=CARTESIAN_POINT('Ctrl Pts',(4.72719156090807,4.8,80.2147259216641));
#36478=CARTESIAN_POINT('Ctrl Pts',(4.73469331137732,4.8,80.2116628411954));
#36479=CARTESIAN_POINT('Ctrl Pts',(4.7415112563347,4.8,80.2085829347521));
#36480=CARTESIAN_POINT('',(5.09956505173093,4.8,79.9735089425676));
#36481=CARTESIAN_POINT('',(7.02338510818378,4.8,78.7104583431054));
#36482=CARTESIAN_POINT('',(5.49567364700612,4.8,80.659589154899));
#36483=CARTESIAN_POINT('Origin',(9.30999999999911,4.8,78.0000000000005));
#36484=CARTESIAN_POINT('',(5.11306670030725,4.8,80.8521358415414));
#36485=CARTESIAN_POINT('',(7.36011410728251,4.8,79.721310756753));
#36486=CARTESIAN_POINT('',(4.58850001701745,4.8,81.7023557244943));
#36487=CARTESIAN_POINT('Ctrl Pts',(5.11306670030725,4.8,80.8521358415414));
#36488=CARTESIAN_POINT('Ctrl Pts',(5.07710170065269,4.8,80.8779694421884));
#36489=CARTESIAN_POINT('Ctrl Pts',(5.03508035307228,4.8,80.9209400583674));
#36490=CARTESIAN_POINT('Ctrl Pts',(4.90769441223799,4.8,81.0639523820827));
#36491=CARTESIAN_POINT('Ctrl Pts',(4.82649708410344,4.8,81.1880512030074));
#36492=CARTESIAN_POINT('Ctrl Pts',(4.69483416885232,4.8,81.4351272139253));
#36493=CARTESIAN_POINT('Ctrl Pts',(4.63976411435854,4.8,81.5587133310751));
#36494=CARTESIAN_POINT('Ctrl Pts',(4.58850001701746,4.8,81.7023557244943));
#36495=CARTESIAN_POINT('',(4.8440115100785,4.8,82.006862464309));
#36496=CARTESIAN_POINT('Origin',(9.31,4.8,78.));
#36497=CARTESIAN_POINT('',(5.77240469132478,4.8,81.6379042610703));
#36498=CARTESIAN_POINT('Ctrl Pts',(4.84401151007851,4.8,82.0068624643091));
#36499=CARTESIAN_POINT('Ctrl Pts',(4.89610959940387,4.8,81.9980125488754));
#36500=CARTESIAN_POINT('Ctrl Pts',(4.94699902627575,4.8,81.988109182246));
#36501=CARTESIAN_POINT('Ctrl Pts',(4.99662552059134,4.8,81.9771196133745));
#36502=CARTESIAN_POINT('Ctrl Pts',(5.03629066414916,4.8,81.9683359418108));
#36503=CARTESIAN_POINT('Ctrl Pts',(5.07515065565679,4.8,81.9588566011248));
#36504=CARTESIAN_POINT('Ctrl Pts',(5.11317313793904,4.8,81.9486898850655));
#36505=CARTESIAN_POINT('Ctrl Pts',(5.14363103907588,4.8,81.9405458393843));
#36506=CARTESIAN_POINT('Ctrl Pts',(5.17355263034768,4.8,81.931960640535));
#36507=CARTESIAN_POINT('Ctrl Pts',(5.20289339622169,4.8,81.9229643737014));
#36508=CARTESIAN_POINT('Ctrl Pts',(5.23492841319329,4.8,81.9131420138512));
#36509=CARTESIAN_POINT('Ctrl Pts',(5.26627194300247,4.8,81.9028292748064));
#36510=CARTESIAN_POINT('Ctrl Pts',(5.29680494952465,4.8,81.8921105713328));
#36511=CARTESIAN_POINT('Ctrl Pts',(5.32334697835746,4.8,81.8827929125414));
#36512=CARTESIAN_POINT('Ctrl Pts',(5.34927161155919,4.8,81.8731723474198));
#36513=CARTESIAN_POINT('Ctrl Pts',(5.37450242539821,4.8,81.863298684267));
#36514=CARTESIAN_POINT('Ctrl Pts',(5.39507286694955,4.8,81.8552487809988));
#36515=CARTESIAN_POINT('Ctrl Pts',(5.41518117055855,4.8,81.847031289851));
#36516=CARTESIAN_POINT('Ctrl Pts',(5.4348165000751,4.8,81.838647073645));
#36517=CARTESIAN_POINT('Ctrl Pts',(5.45628886765119,4.8,81.8294784486897));
#36518=CARTESIAN_POINT('Ctrl Pts',(5.47719881481788,4.8,81.8201078610154));
#36519=CARTESIAN_POINT('Ctrl Pts',(5.49757129198245,4.8,81.810504097856));
#36520=CARTESIAN_POINT('Ctrl Pts',(5.5126899530357,4.8,81.803377029367));
#36521=CARTESIAN_POINT('Ctrl Pts',(5.52751427955579,4.8,81.7961201751675));
#36522=CARTESIAN_POINT('Ctrl Pts',(5.54203764954719,4.8,81.7887340790253));
#36523=CARTESIAN_POINT('Ctrl Pts',(5.55531058243868,4.8,81.7819839130181));
#36524=CARTESIAN_POINT('Ctrl Pts',(5.56833298310324,4.8,81.7751251163156));
#36525=CARTESIAN_POINT('Ctrl Pts',(5.58106953995245,4.8,81.7681824912052));
#36526=CARTESIAN_POINT('Ctrl Pts',(5.59398052898341,4.8,81.761144784099));
#36527=CARTESIAN_POINT('Ctrl Pts',(5.60659809666052,4.8,81.7540206666206));
#36528=CARTESIAN_POINT('Ctrl Pts',(5.6188420757021,4.8,81.7468712319881));
#36529=CARTESIAN_POINT('Ctrl Pts',(5.63589027087475,4.8,81.7369165467854));
#36530=CARTESIAN_POINT('Ctrl Pts',(5.65221101037482,4.8,81.7269151092405));
#36531=CARTESIAN_POINT('Ctrl Pts',(5.6675139932742,4.8,81.7170938785846));
#36532=CARTESIAN_POINT('Ctrl Pts',(5.67899123044873,4.8,81.7097279555928));
#36533=CARTESIAN_POINT('Ctrl Pts',(5.68989303549415,4.8,81.7024657987365));
#36534=CARTESIAN_POINT('Ctrl Pts',(5.70011184948736,4.8,81.6953931429993));
#36535=CARTESIAN_POINT('Ctrl Pts',(5.70998252861731,4.8,81.6885614387111));
#36536=CARTESIAN_POINT('Ctrl Pts',(5.71921514399013,4.8,81.6819072165723));
#36537=CARTESIAN_POINT('Ctrl Pts',(5.72775615332453,4.8,81.6754750210674));
#36538=CARTESIAN_POINT('Ctrl Pts',(5.7375536356891,4.8,81.6680965814056));
#36539=CARTESIAN_POINT('Ctrl Pts',(5.74644207386582,4.8,81.6610096681232));
#36540=CARTESIAN_POINT('Ctrl Pts',(5.75439932669715,4.8,81.6542357282713));
#36541=CARTESIAN_POINT('Ctrl Pts',(5.76104960421005,4.8,81.6485744050953));
#36542=CARTESIAN_POINT('Ctrl Pts',(5.7670513086917,4.8,81.6431303010753));
#36543=CARTESIAN_POINT('Ctrl Pts',(5.77240469132478,4.8,81.6379042610703));
#36544=CARTESIAN_POINT('',(6.02846516020393,4.8,81.2945453548562));
#36545=CARTESIAN_POINT('',(7.40427592391703,4.8,79.4496808154216));
#36546=CARTESIAN_POINT('',(6.63533873676839,4.8,81.8037727491227));
#36547=CARTESIAN_POINT('Origin',(9.3100000000004,4.8,77.9999999999995));
#36548=CARTESIAN_POINT('',(6.34166065765632,4.8,82.1155667324646));
#36549=CARTESIAN_POINT('',(8.06642956697154,4.8,80.2844032686962));
#36550=CARTESIAN_POINT('',(6.13952154251532,4.8,83.0939244547427));
#36551=CARTESIAN_POINT('Ctrl Pts',(6.34166065765632,4.8,82.1155667324646));
#36552=CARTESIAN_POINT('Ctrl Pts',(6.31670022593569,4.8,82.1521431289251));
#36553=CARTESIAN_POINT('Ctrl Pts',(6.29190989233962,4.8,82.2068944446312));
#36554=CARTESIAN_POINT('Ctrl Pts',(6.22111935694833,4.8,82.3848506343714));
#36555=CARTESIAN_POINT('Ctrl Pts',(6.18726312363742,4.8,82.5292365021937));
#36556=CARTESIAN_POINT('Ctrl Pts',(6.14804542664426,4.8,82.8064433752316));
#36557=CARTESIAN_POINT('Ctrl Pts',(6.13856544450829,4.8,82.9414114044585));
#36558=CARTESIAN_POINT('Ctrl Pts',(6.13952154251532,4.8,83.0939244547427));
#36559=CARTESIAN_POINT('',(6.48377124583838,4.8,83.2926771136307));
#36560=CARTESIAN_POINT('Origin',(9.31,4.8,78.));
#36561=CARTESIAN_POINT('',(7.22998432988738,4.8,82.6284406437547));
#36562=CARTESIAN_POINT('Ctrl Pts',(6.48377124583838,4.8,83.2926771136307));
#36563=CARTESIAN_POINT('Ctrl Pts',(6.52970058658809,4.8,83.2665423174258));
#36564=CARTESIAN_POINT('Ctrl Pts',(6.57413385459844,4.8,83.2398309878224));
#36565=CARTESIAN_POINT('Ctrl Pts',(6.61700885117049,4.8,83.2125309103563));
#36566=CARTESIAN_POINT('Ctrl Pts',(6.65127769902839,4.8,83.1907106823448));
#36567=CARTESIAN_POINT('Ctrl Pts',(6.68455201872959,4.8,83.1685121174579));
#36568=CARTESIAN_POINT('Ctrl Pts',(6.71680424110902,4.8,83.1459540760717));
#36569=CARTESIAN_POINT('Ctrl Pts',(6.74263987891727,4.8,83.1278839604665));
#36570=CARTESIAN_POINT('Ctrl Pts',(6.767820667016,4.8,83.1095827252503));
#36571=CARTESIAN_POINT('Ctrl Pts',(6.79231506422289,4.8,83.0910938664587));
#36572=CARTESIAN_POINT('Ctrl Pts',(6.81905868866002,4.8,83.0709072461628));
#36573=CARTESIAN_POINT('Ctrl Pts',(6.84498480814072,4.8,83.0504963226871));
#36574=CARTESIAN_POINT('Ctrl Pts',(6.87001043684679,4.8,83.0299811327162));
#36575=CARTESIAN_POINT('Ctrl Pts',(6.89176495873056,4.8,83.0121474888779));
#36576=CARTESIAN_POINT('Ctrl Pts',(6.91283571842148,4.8,82.9942403679326));
#36577=CARTESIAN_POINT('Ctrl Pts',(6.9331679365434,4.8,82.9763327128294));
#36578=CARTESIAN_POINT('Ctrl Pts',(6.94974459985959,4.8,82.9617327725942));
#36579=CARTESIAN_POINT('Ctrl Pts',(6.96582967712102,4.8,82.9471334117481));
#36580=CARTESIAN_POINT('Ctrl Pts',(6.98141328077829,4.8,82.9325391472623));
#36581=CARTESIAN_POINT('Ctrl Pts',(6.9984548522823,4.8,82.9165794753371));
#36582=CARTESIAN_POINT('Ctrl Pts',(7.01489884612417,4.8,82.9006223796449));
#36583=CARTESIAN_POINT('Ctrl Pts',(7.03075803262354,4.8,82.8846299962369));
#36584=CARTESIAN_POINT('Ctrl Pts',(7.04252732591772,4.8,82.8727618559127));
#36585=CARTESIAN_POINT('Ctrl Pts',(7.05397564589378,4.8,82.8608724252541));
#36586=CARTESIAN_POINT('Ctrl Pts',(7.06509695589111,4.8,82.8489644800917));
#36587=CARTESIAN_POINT('Ctrl Pts',(7.07526074030863,4.8,82.838081788438));
#36588=CARTESIAN_POINT('Ctrl Pts',(7.08515194755247,4.8,82.8271827043902));
#36589=CARTESIAN_POINT('Ctrl Pts',(7.09474587846554,4.8,82.816302611749));
#36590=CARTESIAN_POINT('Ctrl Pts',(7.10447120202654,4.8,82.8052735119704));
#36591=CARTESIAN_POINT('Ctrl Pts',(7.11389124561773,4.8,82.7942635690162));
#36592=CARTESIAN_POINT('Ctrl Pts',(7.12295157174751,4.8,82.7833576105563));
#36593=CARTESIAN_POINT('Ctrl Pts',(7.13556693213933,4.8,82.7681724401309));
#36594=CARTESIAN_POINT('Ctrl Pts',(7.14748271755908,4.8,82.7531921413648));
#36595=CARTESIAN_POINT('Ctrl Pts',(7.15850375899473,4.8,82.7387292749356));
#36596=CARTESIAN_POINT('Ctrl Pts',(7.16676954007146,4.8,82.7278821251137));
#36597=CARTESIAN_POINT('Ctrl Pts',(7.17453008192975,4.8,82.71732929294));
#36598=CARTESIAN_POINT('Ctrl Pts',(7.18171363533377,4.8,82.707188130266));
#36599=CARTESIAN_POINT('Ctrl Pts',(7.18865245925014,4.8,82.6973924569906));
#36600=CARTESIAN_POINT('Ctrl Pts',(7.19505240182619,4.8,82.6879817930411));
#36601=CARTESIAN_POINT('Ctrl Pts',(7.20087838488489,4.8,82.6790163090847));
#36602=CARTESIAN_POINT('Ctrl Pts',(7.20756143170267,4.8,82.6687319075646));
#36603=CARTESIAN_POINT('Ctrl Pts',(7.21348996431612,4.8,82.6590323626442));
#36604=CARTESIAN_POINT('Ctrl Pts',(7.21865051216571,4.8,82.6499454006877));
#36605=CARTESIAN_POINT('Ctrl Pts',(7.2229634423908,4.8,82.6423509680773));
#36606=CARTESIAN_POINT('Ctrl Pts',(7.22674120663366,4.8,82.6351824797662));
#36607=CARTESIAN_POINT('Ctrl Pts',(7.22998432988738,4.8,82.6284406437547));
#36608=CARTESIAN_POINT('',(7.3531668006526,4.8,82.2182109750381));
#36609=CARTESIAN_POINT('',(8.01502518871776,4.8,80.0140503863876));
#36610=CARTESIAN_POINT('',(8.09760744867255,4.8,82.4891652120952));
#36611=CARTESIAN_POINT('Origin',(9.31000000000056,4.8,77.9999999999986));
#36612=CARTESIAN_POINT('',(7.92828014771505,4.8,82.8825995361566));
#36613=CARTESIAN_POINT('',(8.92273797402872,4.8,80.571963032233));
#36614=CARTESIAN_POINT('',(8.07294956130202,4.8,83.871090717415));
#36615=CARTESIAN_POINT('Ctrl Pts',(7.92828014771505,4.8,82.8825995361566));
#36616=CARTESIAN_POINT('Ctrl Pts',(7.9173348789892,4.8,82.9255070749658));
#36617=CARTESIAN_POINT('Ctrl Pts',(7.91276563787875,4.8,82.9854352740174));
#36618=CARTESIAN_POINT('Ctrl Pts',(7.90710889583203,4.8,83.1768711867349));
#36619=CARTESIAN_POINT('Ctrl Pts',(7.92467731857551,4.8,83.324129034775));
#36620=CARTESIAN_POINT('Ctrl Pts',(7.9826350727204,4.8,83.5980315302565));
#36621=CARTESIAN_POINT('Ctrl Pts',(8.01988858795822,4.8,83.7281023348967));
#36622=CARTESIAN_POINT('Ctrl Pts',(8.07294956130202,4.8,83.8710907174151));
#36623=CARTESIAN_POINT('',(8.46441588009367,4.8,83.9401167914581));
#36624=CARTESIAN_POINT('Origin',(9.31,4.8,78.));
#36625=CARTESIAN_POINT('',(8.93844455602746,4.8,83.0607187762934));
#36626=CARTESIAN_POINT('Ctrl Pts',(8.46441588009367,4.8,83.9401167914581));
#36627=CARTESIAN_POINT('Ctrl Pts',(8.58010145233928,4.8,83.8039903313703));
#36628=CARTESIAN_POINT('Ctrl Pts',(8.68428079930222,4.8,83.6590948598213));
#36629=CARTESIAN_POINT('Ctrl Pts',(8.82124532673101,4.8,83.4122455604697));
#36630=CARTESIAN_POINT('Ctrl Pts',(8.85851086683854,4.8,83.3308593655485));
#36631=CARTESIAN_POINT('Ctrl Pts',(8.91127075343445,4.8,83.1876271019925));
#36632=CARTESIAN_POINT('Ctrl Pts',(8.93326894789525,4.8,83.1126668552635));
#36633=CARTESIAN_POINT('Ctrl Pts',(8.93844455602746,4.8,83.0607187762934));
#36634=CARTESIAN_POINT('',(8.91389140472481,4.8,82.6330980974667));
#36635=CARTESIAN_POINT('',(8.78196752755185,4.8,80.3354957565374));
#36636=CARTESIAN_POINT('',(9.70610859527519,4.8,82.6330980974667));
#36637=CARTESIAN_POINT('Origin',(9.31,4.8,78.0000000000002));
#36638=CARTESIAN_POINT('',(9.68155544397255,4.8,83.0607187762934));
#36639=CARTESIAN_POINT('',(9.82575589679681,4.8,80.5493060959508));
#36640=CARTESIAN_POINT('',(10.1555841198781,4.8,83.9401167914621));
#36641=CARTESIAN_POINT('Ctrl Pts',(9.68155544397255,4.8,83.0607187762934));
#36642=CARTESIAN_POINT('Ctrl Pts',(9.68594549803534,4.8,83.1047821733634));
#36643=CARTESIAN_POINT('Ctrl Pts',(9.70214846535674,4.8,83.1626590293364));
#36644=CARTESIAN_POINT('Ctrl Pts',(9.76230780763636,4.8,83.344484671119));
#36645=CARTESIAN_POINT('Ctrl Pts',(9.82918187530145,4.8,83.4768530296735));
#36646=CARTESIAN_POINT('Ctrl Pts',(9.9773245196029,4.8,83.7144144633533));
#36647=CARTESIAN_POINT('Ctrl Pts',(10.0568182080785,4.8,83.8238995857148));
#36648=CARTESIAN_POINT('Ctrl Pts',(10.1555841198781,4.8,83.9401167914621));
#36649=CARTESIAN_POINT('',(10.5470504386678,4.8,83.8710907174214));
#36650=CARTESIAN_POINT('Origin',(9.31,4.8,78.));
#36651=CARTESIAN_POINT('',(10.691719852285,4.8,82.8825995361566));
#36652=CARTESIAN_POINT('Ctrl Pts',(10.5470504386678,4.8,83.8710907174214));
#36653=CARTESIAN_POINT('Ctrl Pts',(10.565435231738,4.8,83.8215474908647));
#36654=CARTESIAN_POINT('Ctrl Pts',(10.5823033780305,4.8,83.7725242711596));
#36655=CARTESIAN_POINT('Ctrl Pts',(10.5975993793386,4.8,83.7240516819789));
#36656=CARTESIAN_POINT('Ctrl Pts',(10.6098250669771,4.8,83.6853088287051));
#36657=CARTESIAN_POINT('Ctrl Pts',(10.6210457117067,4.8,83.6469154229001));
#36658=CARTESIAN_POINT('Ctrl Pts',(10.6312523175355,4.8,83.6089036335644));
#36659=CARTESIAN_POINT('Ctrl Pts',(10.6394283181237,4.8,83.5784542934822));
#36660=CARTESIAN_POINT('Ctrl Pts',(10.6469541138919,4.8,83.5482488347871));
#36661=CARTESIAN_POINT('Ctrl Pts',(10.6538335015972,4.8,83.5183408516636));
#36662=CARTESIAN_POINT('Ctrl Pts',(10.6613445974944,4.8,83.4856865314016));
#36663=CARTESIAN_POINT('Ctrl Pts',(10.6680852688832,4.8,83.4533858670217));
#36664=CARTESIAN_POINT('Ctrl Pts',(10.674069103033,4.8,83.421584154235));
#36665=CARTESIAN_POINT('Ctrl Pts',(10.6792707883309,4.8,83.3939392533715));
#36666=CARTESIAN_POINT('Ctrl Pts',(10.6839014512246,4.8,83.3666775796467));
#36667=CARTESIAN_POINT('Ctrl Pts',(10.6879660151044,4.8,83.339890222103));
#36668=CARTESIAN_POINT('Ctrl Pts',(10.6912798152377,4.8,83.3180507451939));
#36669=CARTESIAN_POINT('Ctrl Pts',(10.6942174110287,4.8,83.2965276975492));
#36670=CARTESIAN_POINT('Ctrl Pts',(10.6967741316292,4.8,83.2753308949627));
#36671=CARTESIAN_POINT('Ctrl Pts',(10.6995700533865,4.8,83.2521509661404));
#36672=CARTESIAN_POINT('Ctrl Pts',(10.7019098600755,4.8,83.2293571263374));
#36673=CARTESIAN_POINT('Ctrl Pts',(10.7037789958498,4.8,83.2069121614836));
#36674=CARTESIAN_POINT('Ctrl Pts',(10.7051661040288,4.8,83.1902554826306));
#36675=CARTESIAN_POINT('Ctrl Pts',(10.7062936472176,4.8,83.1737888121069));
#36676=CARTESIAN_POINT('Ctrl Pts',(10.7071587853345,4.8,83.1575181566129));
#36677=CARTESIAN_POINT('Ctrl Pts',(10.7079494365539,4.8,83.1426483764518));
#36678=CARTESIAN_POINT('Ctrl Pts',(10.7085207447153,4.8,83.1279412482181));
#36679=CARTESIAN_POINT('Ctrl Pts',(10.7088765334352,4.8,83.113439753788));
#36680=CARTESIAN_POINT('Ctrl Pts',(10.7092371948217,4.8,83.098739655688));
#36681=CARTESIAN_POINT('Ctrl Pts',(10.7093763119515,4.8,83.0842504627495));
#36682=CARTESIAN_POINT('Ctrl Pts',(10.7093067094632,4.8,83.070072148483));
#36683=CARTESIAN_POINT('Ctrl Pts',(10.7092097967847,4.8,83.0503306357088));
#36684=CARTESIAN_POINT('Ctrl Pts',(10.7087086675511,4.8,83.031195741855));
#36685=CARTESIAN_POINT('Ctrl Pts',(10.70785472376,4.8,83.0130323545146));
#36686=CARTESIAN_POINT('Ctrl Pts',(10.7072142659167,4.8,82.9994098140094));
#36687=CARTESIAN_POINT('Ctrl Pts',(10.7063759561179,4.8,82.9863374954128));
#36688=CARTESIAN_POINT('Ctrl Pts',(10.705360263576,4.8,82.9739514149783));
#36689=CARTESIAN_POINT('Ctrl Pts',(10.7043791736755,4.8,82.9619873038731));
#36690=CARTESIAN_POINT('Ctrl Pts',(10.7032327559455,4.8,82.9506645132699));
#36691=CARTESIAN_POINT('Ctrl Pts',(10.7019328158995,4.8,82.9400516843912));
#36692=CARTESIAN_POINT('Ctrl Pts',(10.7004416409093,4.8,82.9278775960186));
#36693=CARTESIAN_POINT('Ctrl Pts',(10.6987484130779,4.8,82.916636526183));
#36694=CARTESIAN_POINT('Ctrl Pts',(10.6968606355152,4.8,82.9063583732204));
#36695=CARTESIAN_POINT('Ctrl Pts',(10.6952829245654,4.8,82.8977684022446));
#36696=CARTESIAN_POINT('Ctrl Pts',(10.6935690444019,4.8,82.8898487215898));
#36697=CARTESIAN_POINT('Ctrl Pts',(10.691719852285,4.8,82.8825995361566));
#36698=CARTESIAN_POINT('',(10.5223925513275,4.8,82.4891652120952));
#36699=CARTESIAN_POINT('',(9.61259837549256,4.8,80.3752458702023));
#36700=CARTESIAN_POINT('',(11.2668331993474,4.8,82.2182109750381));
#36701=CARTESIAN_POINT('Origin',(9.31000000000013,4.8,78.0000000000003));
#36702=CARTESIAN_POINT('',(11.3900156701126,4.8,82.6284406437547));
#36703=CARTESIAN_POINT('',(10.6665660466648,4.8,80.2191652207459));
#36704=CARTESIAN_POINT('',(12.1362287541399,4.8,83.2926771136423));
#36705=CARTESIAN_POINT('Ctrl Pts',(11.3900156701126,4.8,82.6284406437547));
#36706=CARTESIAN_POINT('Ctrl Pts',(11.4092115405355,4.8,82.6683452050612));
#36707=CARTESIAN_POINT('Ctrl Pts',(11.4442323990395,4.8,82.7171899177271));
#36708=CARTESIAN_POINT('Ctrl Pts',(11.5629517238869,4.8,82.8674744276728));
#36709=CARTESIAN_POINT('Ctrl Pts',(11.6710654366442,4.8,82.9689877189041));
#36710=CARTESIAN_POINT('Ctrl Pts',(11.8915247821159,4.8,83.1415546766503));
#36711=CARTESIAN_POINT('Ctrl Pts',(12.0036705310799,4.8,83.2172485947785));
#36712=CARTESIAN_POINT('Ctrl Pts',(12.1362287541399,4.8,83.2926771136423));
#36713=CARTESIAN_POINT('',(12.4804784574569,4.8,83.09392445476));
#36714=CARTESIAN_POINT('Origin',(9.31,4.8,78.));
#36715=CARTESIAN_POINT('',(12.2783393423437,4.8,82.1155667324646));
#36716=CARTESIAN_POINT('Ctrl Pts',(12.4804784574569,4.8,83.09392445476));
#36717=CARTESIAN_POINT('Ctrl Pts',(12.4808097303862,4.8,83.0410810807943));
#36718=CARTESIAN_POINT('Ctrl Pts',(12.4798936743225,4.8,82.9892450771466));
#36719=CARTESIAN_POINT('Ctrl Pts',(12.4776886119629,4.8,82.9384642022077));
#36720=CARTESIAN_POINT('Ctrl Pts',(12.4759261639599,4.8,82.8978763924165));
#36721=CARTESIAN_POINT('Ctrl Pts',(12.4733388024296,4.8,82.857960700928));
#36722=CARTESIAN_POINT('Ctrl Pts',(12.4699290763522,4.8,82.8187504335389));
#36723=CARTESIAN_POINT('Ctrl Pts',(12.4671977160268,4.8,82.7873410574586));
#36724=CARTESIAN_POINT('Ctrl Pts',(12.4639387754109,4.8,82.7563832380486));
#36725=CARTESIAN_POINT('Ctrl Pts',(12.4601741525764,4.8,82.7259260387977));
#36726=CARTESIAN_POINT('Ctrl Pts',(12.4560638384958,4.8,82.6926720687609));
#36727=CARTESIAN_POINT('Ctrl Pts',(12.451350519618,4.8,82.6600139272687));
#36728=CARTESIAN_POINT('Ctrl Pts',(12.4460966578638,4.8,82.6280835005169));
#36729=CARTESIAN_POINT('Ctrl Pts',(12.4415295301632,4.8,82.6003267106864));
#36730=CARTESIAN_POINT('Ctrl Pts',(12.4365568883439,4.8,82.5731253377266));
#36731=CARTESIAN_POINT('Ctrl Pts',(12.4312145131633,4.8,82.5465632934318));
#36732=CARTESIAN_POINT('Ctrl Pts',(12.4268589256494,4.8,82.524907512143));
#36733=CARTESIAN_POINT('Ctrl Pts',(12.4222580468816,4.8,82.5036777465558));
#36734=CARTESIAN_POINT('Ctrl Pts',(12.4174108448943,4.8,82.4828848180173));
#36735=CARTESIAN_POINT('Ctrl Pts',(12.4121101496759,4.8,82.4601465502152));
#36736=CARTESIAN_POINT('Ctrl Pts',(12.4065128967569,4.8,82.4379270878765));
#36737=CARTESIAN_POINT('Ctrl Pts',(12.4005926801591,4.8,82.4161964396135));
#36738=CARTESIAN_POINT('Ctrl Pts',(12.3961992158058,4.8,82.4000698626646));
#36739=CARTESIAN_POINT('Ctrl Pts',(12.3916268268252,4.8,82.3842106115907));
#36740=CARTESIAN_POINT('Ctrl Pts',(12.386874898827,4.8,82.368625302211));
#36741=CARTESIAN_POINT('Ctrl Pts',(12.3825321035846,4.8,82.3543818609281));
#36742=CARTESIAN_POINT('Ctrl Pts',(12.3780388235253,4.8,82.3403662822065));
#36743=CARTESIAN_POINT('Ctrl Pts',(12.3734133523422,4.8,82.326617648047));
#36744=CARTESIAN_POINT('Ctrl Pts',(12.3687245334624,4.8,82.3126807207881));
#36745=CARTESIAN_POINT('Ctrl Pts',(12.3638996648925,4.8,82.2990177521613));
#36746=CARTESIAN_POINT('Ctrl Pts',(12.3589849908085,4.8,82.2857183002578));
#36747=CARTESIAN_POINT('Ctrl Pts',(12.3521419277283,4.8,82.2672004928195));
#36748=CARTESIAN_POINT('Ctrl Pts',(12.3451265012387,4.8,82.2493909709054));
#36749=CARTESIAN_POINT('Ctrl Pts',(12.3381118123199,4.8,82.2326150361613));
#36750=CARTESIAN_POINT('Ctrl Pts',(12.3328507956308,4.8,82.2200330851033));
#36751=CARTESIAN_POINT('Ctrl Pts',(12.3275920459005,4.8,82.2080358428568));
#36752=CARTESIAN_POINT('Ctrl Pts',(12.3224013181914,4.8,82.1967441220017));
#36753=CARTESIAN_POINT('Ctrl Pts',(12.3173874282394,4.8,82.1858370875918));
#36754=CARTESIAN_POINT('Ctrl Pts',(12.3124375254797,4.8,82.1755892427828));
#36755=CARTESIAN_POINT('Ctrl Pts',(12.3075861801448,4.8,82.1660610515014));
#36756=CARTESIAN_POINT('Ctrl Pts',(12.3020211505258,4.8,82.15513116236));
#36757=CARTESIAN_POINT('Ctrl Pts',(12.2965853644795,4.8,82.1451471300143));
#36758=CARTESIAN_POINT('Ctrl Pts',(12.2912960984526,4.8,82.136134483496));
#36759=CARTESIAN_POINT('Ctrl Pts',(12.2868755922982,4.8,82.1286021606371));
#36760=CARTESIAN_POINT('Ctrl Pts',(12.2825563817151,4.8,82.1217462771787));
#36761=CARTESIAN_POINT('Ctrl Pts',(12.2783393423437,4.8,82.1155667324646));
#36762=CARTESIAN_POINT('',(11.9846612632316,4.8,81.8037727491227));
#36763=CARTESIAN_POINT('',(10.4067313934724,4.8,80.1285062770252));
#36764=CARTESIAN_POINT('',(12.5915348397961,4.8,81.2945453548562));
#36765=CARTESIAN_POINT('Origin',(9.31000000000031,4.8,78.0000000000004));
#36766=CARTESIAN_POINT('',(12.8475953086752,4.8,81.6379042610703));
#36767=CARTESIAN_POINT('',(11.3437543105226,4.8,79.6213602685287));
#36768=CARTESIAN_POINT('',(13.7759884899248,4.8,82.0068624643054));
#36769=CARTESIAN_POINT('Ctrl Pts',(12.8475953086752,4.8,81.6379042610703));
#36770=CARTESIAN_POINT('Ctrl Pts',(12.8792816901564,4.8,81.668836908395));
#36771=CARTESIAN_POINT('Ctrl Pts',(12.9288964078831,4.8,81.7027580854298));
#36772=CARTESIAN_POINT('Ctrl Pts',(13.0918564124497,4.8,81.8033749305029));
#36773=CARTESIAN_POINT('Ctrl Pts',(13.2281696606021,4.8,81.8617891535078));
#36774=CARTESIAN_POINT('Ctrl Pts',(13.4943550569333,4.8,81.9485475134328));
#36775=CARTESIAN_POINT('Ctrl Pts',(13.6256264337655,4.8,81.9813204243067));
#36776=CARTESIAN_POINT('Ctrl Pts',(13.7759884899248,4.8,82.0068624643054));
#36777=CARTESIAN_POINT('',(14.0314999829639,4.8,81.7023557245181));
#36778=CARTESIAN_POINT('Origin',(9.31,4.8,78.));
#36779=CARTESIAN_POINT('',(13.5069332996928,4.8,80.8521358415414));
#36780=CARTESIAN_POINT('Ctrl Pts',(14.0314999829639,4.8,81.7023557245181));
#36781=CARTESIAN_POINT('Ctrl Pts',(14.0137377793507,4.8,81.6525858939324));
#36782=CARTESIAN_POINT('Ctrl Pts',(13.9951480108104,4.8,81.6041892934436));
#36783=CARTESIAN_POINT('Ctrl Pts',(13.9757078478474,4.8,81.5572250557336));
#36784=CARTESIAN_POINT('Ctrl Pts',(13.9601698393049,4.8,81.5196877815801));
#36785=CARTESIAN_POINT('Ctrl Pts',(13.9440865435676,4.8,81.483064229152));
#36786=CARTESIAN_POINT('Ctrl Pts',(13.9274717471481,4.8,81.4473848238621));
#36787=CARTESIAN_POINT('Ctrl Pts',(13.9141624688315,4.8,81.4188038456076));
#36788=CARTESIAN_POINT('Ctrl Pts',(13.9005118686982,4.8,81.3908276348962));
#36789=CARTESIAN_POINT('Ctrl Pts',(13.8865573049032,4.8,81.3634948067451));
#36790=CARTESIAN_POINT('Ctrl Pts',(13.8713213455486,4.8,81.3336521069032));
#36791=CARTESIAN_POINT('Ctrl Pts',(13.8557225324051,4.8,81.3045755425303));
#36792=CARTESIAN_POINT('Ctrl Pts',(13.8398646682139,4.8,81.2763676828765));
#36793=CARTESIAN_POINT('Ctrl Pts',(13.8260795908255,4.8,81.2518468821179));
#36794=CARTESIAN_POINT('Ctrl Pts',(13.812103418573,4.8,81.2279866964885));
#36795=CARTESIAN_POINT('Ctrl Pts',(13.7979984738936,4.8,81.2048537395401));
#36796=CARTESIAN_POINT('Ctrl Pts',(13.786498847035,4.8,81.1859936603912));
#36797=CARTESIAN_POINT('Ctrl Pts',(13.7749144277477,4.8,81.1676177996027));
#36798=CARTESIAN_POINT('Ctrl Pts',(13.7632479474187,4.8,81.1497366788665));
#36799=CARTESIAN_POINT('Ctrl Pts',(13.750489977824,4.8,81.1301826412959));
#36800=CARTESIAN_POINT('Ctrl Pts',(13.7376307770682,4.8,81.1112175500781));
#36801=CARTESIAN_POINT('Ctrl Pts',(13.7246352739907,4.8,81.0928222539058));
#36802=CARTESIAN_POINT('Ctrl Pts',(13.7149911538226,4.8,81.0791708819076));
#36803=CARTESIAN_POINT('Ctrl Pts',(13.7052703303368,4.8,81.0658319098867));
#36804=CARTESIAN_POINT('Ctrl Pts',(13.6954744889387,4.8,81.0528117648138));
#36805=CARTESIAN_POINT('Ctrl Pts',(13.6865220524789,4.8,81.040912631628));
#36806=CARTESIAN_POINT('Ctrl Pts',(13.6775061401329,4.8,81.0292790880483));
#36807=CARTESIAN_POINT('Ctrl Pts',(13.6684573091815,4.8,81.0179416023308));
#36808=CARTESIAN_POINT('Ctrl Pts',(13.6592845507989,4.8,81.0064488451214));
#36809=CARTESIAN_POINT('Ctrl Pts',(13.6500776468974,4.8,80.9952600565541));
#36810=CARTESIAN_POINT('Ctrl Pts',(13.6409106834611,4.8,80.9844435772673));
#36811=CARTESIAN_POINT('Ctrl Pts',(13.6281468444773,4.8,80.9693829957619));
#36812=CARTESIAN_POINT('Ctrl Pts',(13.6154632847898,4.8,80.9550469366923));
#36813=CARTESIAN_POINT('Ctrl Pts',(13.6031339258266,4.8,80.9416818795899));
#36814=CARTESIAN_POINT('Ctrl Pts',(13.5938869066041,4.8,80.9316580867631));
#36815=CARTESIAN_POINT('Ctrl Pts',(13.584841999819,4.8,80.9221829651429));
#36816=CARTESIAN_POINT('Ctrl Pts',(13.5761023153521,4.8,80.9133475518622));
#36817=CARTESIAN_POINT('Ctrl Pts',(13.5676603744987,4.8,80.9048131434847));
#36818=CARTESIAN_POINT('Ctrl Pts',(13.5595040180612,4.8,80.8968762858028));
#36819=CARTESIAN_POINT('Ctrl Pts',(13.5516864113113,4.8,80.8895819726066));
#36820=CARTESIAN_POINT('Ctrl Pts',(13.5427187517547,4.8,80.8812145886315));
#36821=CARTESIAN_POINT('Ctrl Pts',(13.5341960435113,4.8,80.8736918154127));
#36822=CARTESIAN_POINT('Ctrl Pts',(13.5261432525711,4.8,80.8670317335012));
#36823=CARTESIAN_POINT('Ctrl Pts',(13.5194131295563,4.8,80.8614655675736));
#36824=CARTESIAN_POINT('Ctrl Pts',(13.5130095491284,4.8,80.8565004016111));
#36825=CARTESIAN_POINT('Ctrl Pts',(13.5069332996928,4.8,80.8521358415414));
#36826=CARTESIAN_POINT('',(13.1243263529939,4.8,80.659589154899));
#36827=CARTESIAN_POINT('',(11.0685824193681,4.8,79.6250374134319));
#36828=CARTESIAN_POINT('',(13.5204349482691,4.8,79.9735089425676));
#36829=CARTESIAN_POINT('Origin',(9.31000000000061,4.8,78.0000000000004));
#36830=CARTESIAN_POINT('',(13.8784887436653,4.8,80.2085829347521));
#36831=CARTESIAN_POINT('',(11.7756417895143,4.8,78.8279953391977));
#36832=CARTESIAN_POINT('',(14.877084102819,4.8,80.237761066812));
#36833=CARTESIAN_POINT('Ctrl Pts',(13.8784887436653,4.8,80.2085829347521));
#36834=CARTESIAN_POINT('Ctrl Pts',(13.9188437915828,4.8,80.226812734718));
#36835=CARTESIAN_POINT('Ctrl Pts',(13.9770681023252,4.8,80.241718981607));
#36836=CARTESIAN_POINT('Ctrl Pts',(14.1646134025171,4.8,80.2805322840692));
#36837=CARTESIAN_POINT('Ctrl Pts',(14.3126847969111,4.8,80.2888018216863));
#36838=CARTESIAN_POINT('Ctrl Pts',(14.5924903558759,4.8,80.2792872449101));
#36839=CARTESIAN_POINT('Ctrl Pts',(14.7270540960429,4.8,80.2651862522944));
#36840=CARTESIAN_POINT('Ctrl Pts',(14.877084102819,4.8,80.237761066812));
#36841=CARTESIAN_POINT('',(15.0130389285914,4.8,79.8642282529162));
#36842=CARTESIAN_POINT('Origin',(9.31,4.8,78.));
#36843=CARTESIAN_POINT('',(14.2293151609602,4.8,79.2446952750862));
#36844=CARTESIAN_POINT('Ctrl Pts',(15.0130389285914,4.8,79.8642282529162));
#36845=CARTESIAN_POINT('Ctrl Pts',(14.9793256323352,4.8,79.8235349418062));
#36846=CARTESIAN_POINT('Ctrl Pts',(14.9453043517715,4.8,79.7844150887897));
#36847=CARTESIAN_POINT('Ctrl Pts',(14.9109738587714,4.8,79.7469320685151));
#36848=CARTESIAN_POINT('Ctrl Pts',(14.8835344026255,4.8,79.7169728805989));
#36849=CARTESIAN_POINT('Ctrl Pts',(14.8558950553602,4.8,79.6880588094625));
#36850=CARTESIAN_POINT('Ctrl Pts',(14.8280791781634,4.8,79.6602137303782));
#36851=CARTESIAN_POINT('Ctrl Pts',(14.8057972773248,4.8,79.6379084373754));
#36852=CARTESIAN_POINT('Ctrl Pts',(14.7834014815771,4.8,79.6162881788984));
#36853=CARTESIAN_POINT('Ctrl Pts',(14.7609401032154,4.8,79.5953764639576));
#36854=CARTESIAN_POINT('Ctrl Pts',(14.7364161795572,4.8,79.5725445035804));
#36855=CARTESIAN_POINT('Ctrl Pts',(14.7118133186302,4.8,79.5505565783982));
#36856=CARTESIAN_POINT('Ctrl Pts',(14.6872641438652,4.8,79.5294735693576));
#36857=CARTESIAN_POINT('Ctrl Pts',(14.6659238006834,4.8,79.5111463281149));
#36858=CARTESIAN_POINT('Ctrl Pts',(14.6446298307527,4.8,79.4935052203248));
#36859=CARTESIAN_POINT('Ctrl Pts',(14.6234635811816,4.8,79.4765915267188));
#36860=CARTESIAN_POINT('Ctrl Pts',(14.6062069397889,4.8,79.4628019536438));
#36861=CARTESIAN_POINT('Ctrl Pts',(14.5890362320106,4.8,79.4494963977045));
#36862=CARTESIAN_POINT('Ctrl Pts',(14.5719576231394,4.8,79.4366838118659));
#36863=CARTESIAN_POINT('Ctrl Pts',(14.553281178991,4.8,79.4226725100313));
#36864=CARTESIAN_POINT('Ctrl Pts',(14.5347110401775,4.8,79.4092492598048));
#36865=CARTESIAN_POINT('Ctrl Pts',(14.5162077004567,4.8,79.3964080598874));
#36866=CARTESIAN_POINT('Ctrl Pts',(14.5024761477173,4.8,79.3868784497433));
#36867=CARTESIAN_POINT('Ctrl Pts',(14.4887793645206,4.8,79.3776686336305));
#36868=CARTESIAN_POINT('Ctrl Pts',(14.4751211327833,4.8,79.3687840744841));
#36869=CARTESIAN_POINT('Ctrl Pts',(14.462638851088,4.8,79.3606644604567));
#36870=CARTESIAN_POINT('Ctrl Pts',(14.4501877585656,4.8,79.3528161290529));
#36871=CARTESIAN_POINT('Ctrl Pts',(14.4378069904251,4.8,79.3452572598632));
#36872=CARTESIAN_POINT('Ctrl Pts',(14.4252566625921,4.8,79.3375948688627));
#36873=CARTESIAN_POINT('Ctrl Pts',(14.4127782118658,4.8,79.330229793408));
#36874=CARTESIAN_POINT('Ctrl Pts',(14.4004646301748,4.8,79.3232009137939));
#36875=CARTESIAN_POINT('Ctrl Pts',(14.3833195226597,4.8,79.3134140865556));
#36876=CARTESIAN_POINT('Ctrl Pts',(14.3664976542761,4.8,79.3042806305664));
#36877=CARTESIAN_POINT('Ctrl Pts',(14.3503407279331,4.8,79.2959384741763));
#36878=CARTESIAN_POINT('Ctrl Pts',(14.3382230331759,4.8,79.2896818568836));
#36879=CARTESIAN_POINT('Ctrl Pts',(14.3264829185903,4.8,79.2838716953493));
#36880=CARTESIAN_POINT('Ctrl Pts',(14.3152484123024,4.8,79.2785582708383));
#36881=CARTESIAN_POINT('Ctrl Pts',(14.3043966432488,4.8,79.2734258641086));
#36882=CARTESIAN_POINT('Ctrl Pts',(14.2940176101361,4.8,79.2687572957321));
#36883=CARTESIAN_POINT('Ctrl Pts',(14.2841766607576,4.8,79.2645766624468));
#36884=CARTESIAN_POINT('Ctrl Pts',(14.2728880033202,4.8,79.2597810136519));
#36885=CARTESIAN_POINT('Ctrl Pts',(14.2623063372479,4.8,79.2556268570475));
#36886=CARTESIAN_POINT('Ctrl Pts',(14.2524613068071,4.8,79.2521226439224));
#36887=CARTESIAN_POINT('Ctrl Pts',(14.2442333190914,4.8,79.2491939965485));
#36888=CARTESIAN_POINT('Ctrl Pts',(14.2365177351167,4.8,79.2467184202557));
#36889=CARTESIAN_POINT('Ctrl Pts',(14.2293151609602,4.8,79.2446952750862));
#36890=CARTESIAN_POINT('',(13.8039273911235,4.8,79.194619857239));
#36891=CARTESIAN_POINT('',(11.5183224515755,4.8,78.9255650547807));
#36892=CARTESIAN_POINT('',(13.941494462579,4.8,78.4144382259154));
#36893=CARTESIAN_POINT('Origin',(9.30999999999925,4.8,77.9999999999999));
#36894=CARTESIAN_POINT('',(14.3583550124563,4.8,78.5128739112901));
#36895=CARTESIAN_POINT('',(11.9101364796933,4.8,77.9347619520498));
#36896=CARTESIAN_POINT('',(15.306707211514,4.8,78.1987526587886));
#36897=CARTESIAN_POINT('Ctrl Pts',(14.3583550124563,4.8,78.5128739112901));
#36898=CARTESIAN_POINT('Ctrl Pts',(14.4025113095208,4.8,78.5162020802714));
#36899=CARTESIAN_POINT('Ctrl Pts',(14.4623224986856,4.8,78.5102954845377));
#36900=CARTESIAN_POINT('Ctrl Pts',(14.655508486079,4.8,78.4820870105105));
#36901=CARTESIAN_POINT('Ctrl Pts',(14.7941933914243,4.8,78.4380535020656));
#36902=CARTESIAN_POINT('Ctrl Pts',(15.0510922588474,4.8,78.3375379190762));
#36903=CARTESIAN_POINT('Ctrl Pts',(15.1814858801512,4.8,78.2720997067482));
#36904=CARTESIAN_POINT('Ctrl Pts',(15.306707211514,4.8,78.1987526587886));
#36905=CARTESIAN_POINT('',(15.3067072115039,4.8,77.8012473409061));
#36906=CARTESIAN_POINT('Origin',(9.31,4.8,78.));
#36907=CARTESIAN_POINT('',(14.3583550124563,4.8,77.4871260887099));
#36908=CARTESIAN_POINT('Ctrl Pts',(15.3067072115039,4.8,77.8012473409061));
#36909=CARTESIAN_POINT('Ctrl Pts',(15.2611091436898,4.8,77.7745387631645));
#36910=CARTESIAN_POINT('Ctrl Pts',(15.2157598196307,4.8,77.7494140892397));
#36911=CARTESIAN_POINT('Ctrl Pts',(15.1706797607092,4.8,77.7259332918341));
#36912=CARTESIAN_POINT('Ctrl Pts',(15.1346484571073,4.8,77.7071657089965));
#36913=CARTESIAN_POINT('Ctrl Pts',(15.0987867683259,4.8,77.6894485816647));
#36914=CARTESIAN_POINT('Ctrl Pts',(15.063124812535,4.8,77.6727963552642));
#36915=CARTESIAN_POINT('Ctrl Pts',(15.0345578158729,4.8,77.6594570953877));
#36916=CARTESIAN_POINT('Ctrl Pts',(15.006118088614,4.8,77.6468005117217));
#36917=CARTESIAN_POINT('Ctrl Pts',(14.9778590700176,4.8,77.6348321717349));
#36918=CARTESIAN_POINT('Ctrl Pts',(14.9470051291957,4.8,77.6217648229016));
#36919=CARTESIAN_POINT('Ctrl Pts',(14.9163656886571,4.8,77.6095176058724));
#36920=CARTESIAN_POINT('Ctrl Pts',(14.8860861961812,4.8,77.5981023701413));
#36921=CARTESIAN_POINT('Ctrl Pts',(14.8597645479413,4.8,77.5881792243115));
#36922=CARTESIAN_POINT('Ctrl Pts',(14.833721147768,4.8,77.5788849724225));
#36923=CARTESIAN_POINT('Ctrl Pts',(14.8080465557734,4.8,77.5702305833215));
#36924=CARTESIAN_POINT('Ctrl Pts',(14.7871143057029,4.8,77.5631747423989));
#36925=CARTESIAN_POINT('Ctrl Pts',(14.7664283504253,4.8,77.5565443377725));
#36926=CARTESIAN_POINT('Ctrl Pts',(14.7459975455092,4.8,77.5503456738222));
#36927=CARTESIAN_POINT('Ctrl Pts',(14.723655282707,4.8,77.5435670775032));
#36928=CARTESIAN_POINT('Ctrl Pts',(14.7016140396996,4.8,77.537304710313));
#36929=CARTESIAN_POINT('Ctrl Pts',(14.6798346402041,4.8,77.5315664448051));
#36930=CARTESIAN_POINT('Ctrl Pts',(14.6636718829377,4.8,77.5273080081778));
#36931=CARTESIAN_POINT('Ctrl Pts',(14.6476511743518,4.8,77.5233381877535));
#36932=CARTESIAN_POINT('Ctrl Pts',(14.6317779367209,4.8,77.5196608235206));
#36933=CARTESIAN_POINT('Ctrl Pts',(14.6172713572202,4.8,77.5163000739471));
#36934=CARTESIAN_POINT('Ctrl Pts',(14.6028868700773,4.8,77.5131835793267));
#36935=CARTESIAN_POINT('Ctrl Pts',(14.5886674681478,4.8,77.5103150378569));
#36936=CARTESIAN_POINT('Ctrl Pts',(14.5742533255308,4.8,77.5074072105056));
#36937=CARTESIAN_POINT('Ctrl Pts',(14.5600084132126,4.8,77.5047541849647));
#36938=CARTESIAN_POINT('Ctrl Pts',(14.5460334128722,4.8,77.5023606916477));
#36939=CARTESIAN_POINT('Ctrl Pts',(14.5265749900718,4.8,77.4990280545245));
#36940=CARTESIAN_POINT('Ctrl Pts',(14.5076437788303,4.8,77.4961988312379));
#36941=CARTESIAN_POINT('Ctrl Pts',(14.4896080491137,4.8,77.4938857627618));
#36942=CARTESIAN_POINT('Ctrl Pts',(14.4760812518262,4.8,77.4921509614047));
#36943=CARTESIAN_POINT('Ctrl Pts',(14.4630619606985,4.8,77.4907065511982));
#36944=CARTESIAN_POINT('Ctrl Pts',(14.4506876800147,4.8,77.4895559928777));
#36945=CARTESIAN_POINT('Ctrl Pts',(14.4387349662656,4.8,77.4884446317726));
#36946=CARTESIAN_POINT('Ctrl Pts',(14.4273851210563,4.8,77.487607450931));
#36947=CARTESIAN_POINT('Ctrl Pts',(14.4167077927931,4.8,77.4870447436184));
#36948=CARTESIAN_POINT('Ctrl Pts',(14.4044597161182,4.8,77.4863992560827));
#36949=CARTESIAN_POINT('Ctrl Pts',(14.3930953972864,4.8,77.4861147687456));
#36950=CARTESIAN_POINT('Ctrl Pts',(14.3826455833045,4.8,77.486189084285));
#36951=CARTESIAN_POINT('Ctrl Pts',(14.3739121480898,4.8,77.4862511935197));
#36952=CARTESIAN_POINT('Ctrl Pts',(14.3658151742579,4.8,77.4865637978793));
#36953=CARTESIAN_POINT('Ctrl Pts',(14.3583550124563,4.8,77.4871260887099));
#36954=CARTESIAN_POINT('',(13.941494462579,4.8,77.5855617740846));
#36955=CARTESIAN_POINT('',(11.7017062047547,4.8,78.1144558906375));
#36956=CARTESIAN_POINT('',(13.8039273911235,4.8,76.805380142761));
#36957=CARTESIAN_POINT('Origin',(9.30999999999972,4.8,78.0000000000001));
#36958=CARTESIAN_POINT('',(14.2293151609602,4.8,76.7553047249138));
#36959=CARTESIAN_POINT('',(11.7310163364939,4.8,77.0493972362957));
#36960=CARTESIAN_POINT('',(15.0130389285309,4.8,76.1357717468986));
#36961=CARTESIAN_POINT('Ctrl Pts',(14.2293151609602,4.8,76.7553047249138));
#36962=CARTESIAN_POINT('Ctrl Pts',(14.2719468108673,4.8,76.7433298370116));
#36963=CARTESIAN_POINT('Ctrl Pts',(14.3261307716226,4.8,76.7173228190353));
#36964=CARTESIAN_POINT('Ctrl Pts',(14.4947475177318,4.8,76.62650373751));
#36965=CARTESIAN_POINT('Ctrl Pts',(14.6134923426114,4.8,76.5376601132773));
#36966=CARTESIAN_POINT('Ctrl Pts',(14.8217199834009,4.8,76.3505159786347));
#36967=CARTESIAN_POINT('Ctrl Pts',(14.9157378453733,4.8,76.2532180867664));
#36968=CARTESIAN_POINT('Ctrl Pts',(15.0130389285309,4.8,76.1357717468986));
#36969=CARTESIAN_POINT('',(14.8770841027247,4.8,75.7622389329533));
#36970=CARTESIAN_POINT('Origin',(9.31,4.8,78.));
#36971=CARTESIAN_POINT('',(13.8784887436653,4.8,75.7914170652479));
#36972=CARTESIAN_POINT('Ctrl Pts',(14.8770841027247,4.8,75.7622389329533));
#36973=CARTESIAN_POINT('Ctrl Pts',(14.7013523460961,4.8,75.7301155190193));
#36974=CARTESIAN_POINT('Ctrl Pts',(14.5237795099726,4.8,75.7123412935216));
#36975=CARTESIAN_POINT('Ctrl Pts',(14.241519484279,4.8,75.7171511830311));
#36976=CARTESIAN_POINT('Ctrl Pts',(14.1524042015108,4.8,75.7255713759847));
#36977=CARTESIAN_POINT('Ctrl Pts',(14.0019814863757,4.8,75.751496104531));
#36978=CARTESIAN_POINT('Ctrl Pts',(13.9260649067567,4.8,75.7699252323531));
#36979=CARTESIAN_POINT('Ctrl Pts',(13.8784887436653,4.8,75.7914170652479));
#36980=CARTESIAN_POINT('',(13.5204349482691,4.8,76.0264910574324));
#36981=CARTESIAN_POINT('',(11.5966148918162,4.8,77.2895416568946));
#36982=CARTESIAN_POINT('',(13.1243263529939,4.8,75.340410845101));
#36983=CARTESIAN_POINT('Origin',(9.31000000000134,4.8,77.9999999999992));
#36984=CARTESIAN_POINT('',(13.5069332996928,4.8,75.1478641584586));
#36985=CARTESIAN_POINT('',(11.2598858927175,4.8,76.278689243247));
#36986=CARTESIAN_POINT('',(14.0314999829165,4.8,74.2976442754215));
#36987=CARTESIAN_POINT('Ctrl Pts',(13.5069332996928,4.8,75.1478641584586));
#36988=CARTESIAN_POINT('Ctrl Pts',(13.5428982946376,4.8,75.1220305609756));
#36989=CARTESIAN_POINT('Ctrl Pts',(13.5849196393322,4.8,75.079059950823));
#36990=CARTESIAN_POINT('Ctrl Pts',(13.7123055934936,4.8,74.9360476097479));
#36991=CARTESIAN_POINT('Ctrl Pts',(13.7935029203389,4.8,74.8119487895258));
#36992=CARTESIAN_POINT('Ctrl Pts',(13.9251658340055,4.8,74.5648727799932));
#36993=CARTESIAN_POINT('Ctrl Pts',(13.980235886818,4.8,74.4412866654118));
#36994=CARTESIAN_POINT('Ctrl Pts',(14.0314999829165,4.8,74.2976442754215));
#36995=CARTESIAN_POINT('',(13.7759884897161,4.8,73.993137535462));
#36996=CARTESIAN_POINT('Origin',(9.31,4.8,78.));
#36997=CARTESIAN_POINT('',(12.8475953086752,4.8,74.3620957389297));
#36998=CARTESIAN_POINT('Ctrl Pts',(13.7759884897161,4.8,73.993137535462));
#36999=CARTESIAN_POINT('Ctrl Pts',(13.7238904004033,4.8,74.0019874509187));
#37000=CARTESIAN_POINT('Ctrl Pts',(13.6730009735598,4.8,74.0118908177042));
#37001=CARTESIAN_POINT('Ctrl Pts',(13.6233744792638,4.8,74.0228803866613));
#37002=CARTESIAN_POINT('Ctrl Pts',(13.5837093243563,4.8,74.0316640608102));
#37003=CARTESIAN_POINT('Ctrl Pts',(13.5448493219531,4.8,74.0411434044381));
#37004=CARTESIAN_POINT('Ctrl Pts',(13.5068268292634,4.8,74.0513101237898));
#37005=CARTESIAN_POINT('Ctrl Pts',(13.4763689303774,4.8,74.0594541692774));
#37006=CARTESIAN_POINT('Ctrl Pts',(13.4464473412981,4.8,74.068039367854));
#37007=CARTESIAN_POINT('Ctrl Pts',(13.4171065775658,4.8,74.0770356343559));
#37008=CARTESIAN_POINT('Ctrl Pts',(13.3850715584932,4.8,74.0868579952051));
#37009=CARTESIAN_POINT('Ctrl Pts',(13.3537280267159,4.8,74.0971707353158));
#37010=CARTESIAN_POINT('Ctrl Pts',(13.3231950184018,4.8,74.1078894398987));
#37011=CARTESIAN_POINT('Ctrl Pts',(13.2966529914007,4.8,74.1172070984644));
#37012=CARTESIAN_POINT('Ctrl Pts',(13.2707283600065,4.8,74.1268276633136));
#37013=CARTESIAN_POINT('Ctrl Pts',(13.2454975479251,4.8,74.1367013261576));
#37014=CARTESIAN_POINT('Ctrl Pts',(13.2249271074216,4.8,74.1447512293248));
#37015=CARTESIAN_POINT('Ctrl Pts',(13.2048188048439,4.8,74.1529687203539));
#37016=CARTESIAN_POINT('Ctrl Pts',(13.1851834763243,4.8,74.1613529364339));
#37017=CARTESIAN_POINT('Ctrl Pts',(13.1637111136978,4.8,74.1705215596035));
#37018=CARTESIAN_POINT('Ctrl Pts',(13.1428011712343,4.8,74.1798921454136));
#37019=CARTESIAN_POINT('Ctrl Pts',(13.122428698542,4.8,74.1894959066136));
#37020=CARTESIAN_POINT('Ctrl Pts',(13.1073100380069,4.8,74.1966229749688));
#37021=CARTESIAN_POINT('Ctrl Pts',(13.0924857119884,4.8,74.2038798290292));
#37022=CARTESIAN_POINT('Ctrl Pts',(13.0779623424873,4.8,74.211265925024));
#37023=CARTESIAN_POINT('Ctrl Pts',(13.0646894097681,4.8,74.2180160910367));
#37024=CARTESIAN_POINT('Ctrl Pts',(13.0516670092769,4.8,74.2248748877425));
#37025=CARTESIAN_POINT('Ctrl Pts',(13.0389304526091,4.8,74.2318175128486));
#37026=CARTESIAN_POINT('Ctrl Pts',(13.0260194633204,4.8,74.2388552201912));
#37027=CARTESIAN_POINT('Ctrl Pts',(13.0134018954141,4.8,74.245979337904));
#37028=CARTESIAN_POINT('Ctrl Pts',(13.0011579161868,4.8,74.2531287727555));
#37029=CARTESIAN_POINT('Ctrl Pts',(12.9841097219238,4.8,74.263083457581));
#37030=CARTESIAN_POINT('Ctrl Pts',(12.9677889833194,4.8,74.273084894711));
#37031=CARTESIAN_POINT('Ctrl Pts',(12.9524860012689,4.8,74.2829061249336));
#37032=CARTESIAN_POINT('Ctrl Pts',(12.941008764731,4.8,74.2902720476006));
#37033=CARTESIAN_POINT('Ctrl Pts',(12.930106960295,4.8,74.2975342041223));
#37034=CARTESIAN_POINT('Ctrl Pts',(12.9198881468665,4.8,74.3046068595292));
#37035=CARTESIAN_POINT('Ctrl Pts',(12.9100174678259,4.8,74.3114385638141));
#37036=CARTESIAN_POINT('Ctrl Pts',(12.9007848525593,4.8,74.3180927859375));
#37037=CARTESIAN_POINT('Ctrl Pts',(12.8922438433448,4.8,74.3245249814216));
#37038=CARTESIAN_POINT('Ctrl Pts',(12.8824463607762,4.8,74.3319034213167));
#37039=CARTESIAN_POINT('Ctrl Pts',(12.8735579224768,4.8,74.3389903348055));
#37040=CARTESIAN_POINT('Ctrl Pts',(12.8656006696037,4.8,74.3457642748448));
#37041=CARTESIAN_POINT('Ctrl Pts',(12.858950393561,4.8,74.3514255968961));
#37042=CARTESIAN_POINT('Ctrl Pts',(12.8529486903123,4.8,74.3568696998768));
#37043=CARTESIAN_POINT('Ctrl Pts',(12.8475953086752,4.8,74.3620957389297));
#37044=CARTESIAN_POINT('',(12.5915348397961,4.8,74.7054546451438));
#37045=CARTESIAN_POINT('',(11.215724076083,4.8,76.5503191845784));
#37046=CARTESIAN_POINT('',(11.9846612632316,4.8,74.1962272508773));
#37047=CARTESIAN_POINT('Origin',(9.3099999999996,4.8,78.0000000000005));
#37048=CARTESIAN_POINT('',(12.2783393423437,4.8,73.8844332675354));
#37049=CARTESIAN_POINT('',(10.5535704330285,4.8,75.7155967313038));
#37050=CARTESIAN_POINT('',(12.4804784574649,4.8,72.906075545245));
#37051=CARTESIAN_POINT('Ctrl Pts',(12.2783393423437,4.8,73.8844332675354));
#37052=CARTESIAN_POINT('Ctrl Pts',(12.3032997730562,4.8,73.847856872409));
#37053=CARTESIAN_POINT('Ctrl Pts',(12.3280901065664,4.8,73.7931055586751));
#37054=CARTESIAN_POINT('Ctrl Pts',(12.3988806442072,4.8,73.6151493612448));
#37055=CARTESIAN_POINT('Ctrl Pts',(12.4327368770971,4.8,73.4707634939834));
#37056=CARTESIAN_POINT('Ctrl Pts',(12.4719545735749,4.8,73.1935566220854));
#37057=CARTESIAN_POINT('Ctrl Pts',(12.4814345554534,4.8,73.0585885935031));
#37058=CARTESIAN_POINT('Ctrl Pts',(12.4804784574649,4.8,72.906075545245));
#37059=CARTESIAN_POINT('',(12.1362287539072,4.8,72.7073228862334));
#37060=CARTESIAN_POINT('Origin',(9.31,4.8,78.));
#37061=CARTESIAN_POINT('',(11.3900156701126,4.8,73.3715593562453));
#37062=CARTESIAN_POINT('Ctrl Pts',(12.1362287539072,4.8,72.7073228862334));
#37063=CARTESIAN_POINT('Ctrl Pts',(12.0902994131742,4.8,72.7334576824571));
#37064=CARTESIAN_POINT('Ctrl Pts',(12.0458661451943,4.8,72.7601690122162));
#37065=CARTESIAN_POINT('Ctrl Pts',(12.0029911486446,4.8,72.7874690897655));
#37066=CARTESIAN_POINT('Ctrl Pts',(11.9687222872374,4.8,72.8092893264821));
#37067=CARTESIAN_POINT('Ctrl Pts',(11.935447954768,4.8,72.8314879003312));
#37068=CARTESIAN_POINT('Ctrl Pts',(11.9031957204388,4.8,72.8540459509127));
#37069=CARTESIAN_POINT('Ctrl Pts',(11.8773600856403,4.8,72.8721160650835));
#37070=CARTESIAN_POINT('Ctrl Pts',(11.8521793004395,4.8,72.8904172987917));
#37071=CARTESIAN_POINT('Ctrl Pts',(11.8276849060244,4.8,72.90890615602));
#37072=CARTESIAN_POINT('Ctrl Pts',(11.8009412807114,4.8,72.9290927775709));
#37073=CARTESIAN_POINT('Ctrl Pts',(11.7750151604701,4.8,72.949503702302));
#37074=CARTESIAN_POINT('Ctrl Pts',(11.7499895311469,4.8,72.9700188934941));
#37075=CARTESIAN_POINT('Ctrl Pts',(11.7282350112657,4.8,72.9878525363126));
#37076=CARTESIAN_POINT('Ctrl Pts',(11.707164253526,4.8,73.0057596561935));
#37077=CARTESIAN_POINT('Ctrl Pts',(11.6868320372831,4.8,73.0236673102102));
#37078=CARTESIAN_POINT('Ctrl Pts',(11.6702553752548,4.8,73.0382672497746));
#37079=CARTESIAN_POINT('Ctrl Pts',(11.654170299247,4.8,73.0528666099356));
#37080=CARTESIAN_POINT('Ctrl Pts',(11.6385866967945,4.8,73.067460873742));
#37081=CARTESIAN_POINT('Ctrl Pts',(11.6215451301536,4.8,73.0834205416036));
#37082=CARTESIAN_POINT('Ctrl Pts',(11.6051011408651,4.8,73.0993776332441));
#37083=CARTESIAN_POINT('Ctrl Pts',(11.5892419586191,4.8,73.1153700125893));
#37084=CARTESIAN_POINT('Ctrl Pts',(11.5774726658493,4.8,73.1272381525525));
#37085=CARTESIAN_POINT('Ctrl Pts',(11.5660243463772,4.8,73.1391275828518));
#37086=CARTESIAN_POINT('Ctrl Pts',(11.5549030368674,4.8,73.1510355276518));
#37087=CARTESIAN_POINT('Ctrl Pts',(11.5447392527121,4.8,73.1619182191707));
#37088=CARTESIAN_POINT('Ctrl Pts',(11.5348480457267,4.8,73.1728173030816));
#37089=CARTESIAN_POINT('Ctrl Pts',(11.5252541150731,4.8,73.1836973955759));
#37090=CARTESIAN_POINT('Ctrl Pts',(11.5155287913938,4.8,73.1947264956381));
#37091=CARTESIAN_POINT('Ctrl Pts',(11.5061087477094,4.8,73.2057364388639));
#37092=CARTESIAN_POINT('Ctrl Pts',(11.4970484215219,4.8,73.2166423975633));
#37093=CARTESIAN_POINT('Ctrl Pts',(11.484433061942,4.8,73.2318275672483));
#37094=CARTESIAN_POINT('Ctrl Pts',(11.472517277305,4.8,73.2468078652383));
#37095=CARTESIAN_POINT('Ctrl Pts',(11.461496236598,4.8,73.2612707308838));
#37096=CARTESIAN_POINT('Ctrl Pts',(11.4532304560678,4.8,73.272117880118));
#37097=CARTESIAN_POINT('Ctrl Pts',(11.4454699147249,4.8,73.2826707117006));
#37098=CARTESIAN_POINT('Ctrl Pts',(11.4382863617921,4.8,73.2928118738022));
#37099=CARTESIAN_POINT('Ctrl Pts',(11.4313475380429,4.8,73.3026075469311));
#37100=CARTESIAN_POINT('Ctrl Pts',(11.4249475956373,4.8,73.3120182107202));
#37101=CARTESIAN_POINT('Ctrl Pts',(11.4191216127486,4.8,73.3209836945166));
#37102=CARTESIAN_POINT('Ctrl Pts',(11.4124385657172,4.8,73.3312680964817));
#37103=CARTESIAN_POINT('Ctrl Pts',(11.4065100329821,4.8,73.3409676417767));
#37104=CARTESIAN_POINT('Ctrl Pts',(11.4013494851028,4.8,73.350054604053));
#37105=CARTESIAN_POINT('Ctrl Pts',(11.3970365560116,4.8,73.3576490348903));
#37106=CARTESIAN_POINT('Ctrl Pts',(11.3932587926791,4.8,73.3648175216196));
#37107=CARTESIAN_POINT('Ctrl Pts',(11.3900156701126,4.8,73.3715593562453));
#37108=CARTESIAN_POINT('',(11.2668331993474,4.8,73.7817890249619));
#37109=CARTESIAN_POINT('',(10.6049748112822,4.8,75.9859496136124));
#37110=CARTESIAN_POINT('',(10.5223925513275,4.8,73.5108347879048));
#37111=CARTESIAN_POINT('Origin',(9.31000000000015,4.8,77.9999999999997));
#37112=CARTESIAN_POINT('',(10.691719852285,4.8,73.1174004638434));
#37113=CARTESIAN_POINT('',(9.6972620259713,4.8,75.428036967767));
#37114=CARTESIAN_POINT('',(10.5470504387829,4.8,72.1289092826028));
#37115=CARTESIAN_POINT('Ctrl Pts',(10.691719852285,4.8,73.1174004638434));
#37116=CARTESIAN_POINT('Ctrl Pts',(10.7026651211628,4.8,73.0744929241743));
#37117=CARTESIAN_POINT('Ctrl Pts',(10.7072343623596,4.8,73.0145647240501));
#37118=CARTESIAN_POINT('Ctrl Pts',(10.7128911037806,4.8,72.8231288094491));
#37119=CARTESIAN_POINT('Ctrl Pts',(10.6953226809553,4.8,72.6758709620368));
#37120=CARTESIAN_POINT('Ctrl Pts',(10.6373649269874,4.8,72.4019684691396));
#37121=CARTESIAN_POINT('Ctrl Pts',(10.6001114115581,4.8,72.2718976636863));
#37122=CARTESIAN_POINT('Ctrl Pts',(10.5470504387829,4.8,72.1289092826028));
#37123=CARTESIAN_POINT('',(10.1555841196958,4.8,72.059883208512));
#37124=CARTESIAN_POINT('Origin',(9.31,4.8,78.));
#37125=CARTESIAN_POINT('',(9.68155544397255,4.8,72.9392812237066));
#37126=CARTESIAN_POINT('Ctrl Pts',(10.1555841196958,4.8,72.059883208512));
#37127=CARTESIAN_POINT('Ctrl Pts',(10.1213632838796,4.8,72.1001506433707));
#37128=CARTESIAN_POINT('Ctrl Pts',(10.0887454826508,4.8,72.1404481555294));
#37129=CARTESIAN_POINT('Ctrl Pts',(10.0577933412008,4.8,72.1807659494182));
#37130=CARTESIAN_POINT('Ctrl Pts',(10.0330541051411,4.8,72.2129909061963));
#37131=CARTESIAN_POINT('Ctrl Pts',(10.009378819543,4.8,72.2452312346535));
#37132=CARTESIAN_POINT('Ctrl Pts',(9.98678694034531,4.8,72.2774597825885));
#37133=CARTESIAN_POINT('Ctrl Pts',(9.96868972816606,4.8,72.303276442863));
#37134=CARTESIAN_POINT('Ctrl Pts',(9.95128692085213,4.8,72.3290863127067));
#37135=CARTESIAN_POINT('Ctrl Pts',(9.93459328090694,4.8,72.3548377315138));
#37136=CARTESIAN_POINT('Ctrl Pts',(9.91636672526524,4.8,72.3829538086114));
#37137=CARTESIAN_POINT('Ctrl Pts',(9.89898508926508,4.8,72.411001058554));
#37138=CARTESIAN_POINT('Ctrl Pts',(9.88248529911423,4.8,72.4388383009022));
#37139=CARTESIAN_POINT('Ctrl Pts',(9.86814220232304,4.8,72.4630369275363));
#37140=CARTESIAN_POINT('Ctrl Pts',(9.85446676240731,4.8,72.4870707395995));
#37141=CARTESIAN_POINT('Ctrl Pts',(9.84148550717457,4.8,72.5108524575166));
#37142=CARTESIAN_POINT('Ctrl Pts',(9.83090201362154,4.8,72.5302414652623));
#37143=CARTESIAN_POINT('Ctrl Pts',(9.82078026165405,4.8,72.5494617962272));
#37144=CARTESIAN_POINT('Ctrl Pts',(9.81112799762775,4.8,72.5685058241284));
#37145=CARTESIAN_POINT('Ctrl Pts',(9.80057269094209,4.8,72.5893315655792));
#37146=CARTESIAN_POINT('Ctrl Pts',(9.79057804217991,4.8,72.6099505026764));
#37147=CARTESIAN_POINT('Ctrl Pts',(9.78114500139984,4.8,72.6304025835768));
#37148=CARTESIAN_POINT('Ctrl Pts',(9.7741446267435,4.8,72.6455803223508));
#37149=CARTESIAN_POINT('Ctrl Pts',(9.76745315005117,4.8,72.660668288163));
#37150=CARTESIAN_POINT('Ctrl Pts',(9.7610752945402,4.8,72.6756618079211));
#37151=CARTESIAN_POINT('Ctrl Pts',(9.75524656128037,4.8,72.6893644117423));
#37152=CARTESIAN_POINT('Ctrl Pts',(9.7496795733032,4.8,72.7029891924912));
#37153=CARTESIAN_POINT('Ctrl Pts',(9.7443854382534,4.8,72.7164944526537));
#37154=CARTESIAN_POINT('Ctrl Pts',(9.73901879774745,4.8,72.7301846731619));
#37155=CARTESIAN_POINT('Ctrl Pts',(9.73393247457399,4.8,72.7437524802262));
#37156=CARTESIAN_POINT('Ctrl Pts',(9.72914861047331,4.8,72.7570995431718));
#37157=CARTESIAN_POINT('Ctrl Pts',(9.72248768404499,4.8,72.7756836422271));
#37158=CARTESIAN_POINT('Ctrl Pts',(9.71641407278451,4.8,72.7938359561415));
#37159=CARTESIAN_POINT('Ctrl Pts',(9.71100427351269,4.8,72.8111960222505));
#37160=CARTESIAN_POINT('Ctrl Pts',(9.70694692405882,4.8,72.8242160718323));
#37161=CARTESIAN_POINT('Ctrl Pts',(9.70326368157836,4.8,72.8367867513079));
#37162=CARTESIAN_POINT('Ctrl Pts',(9.69998183159711,4.8,72.8487732463486));
#37163=CARTESIAN_POINT('Ctrl Pts',(9.69681178764907,4.8,72.8603513855929));
#37164=CARTESIAN_POINT('Ctrl Pts',(9.69401644557314,4.8,72.8713834261291));
#37165=CARTESIAN_POINT('Ctrl Pts',(9.6916081884937,4.8,72.8818008285971));
#37166=CARTESIAN_POINT('Ctrl Pts',(9.68884565114532,4.8,72.8937507419333));
#37167=CARTESIAN_POINT('Ctrl Pts',(9.68659209254914,4.8,72.9048930106879));
#37168=CARTESIAN_POINT('Ctrl Pts',(9.68485068791891,4.8,72.9151969734135));
#37169=CARTESIAN_POINT('Ctrl Pts',(9.68339530857426,4.8,72.9238085127757));
#37170=CARTESIAN_POINT('Ctrl Pts',(9.68229713908583,4.8,72.9318367581203));
#37171=CARTESIAN_POINT('Ctrl Pts',(9.68155544397255,4.8,72.9392812237066));
#37172=CARTESIAN_POINT('',(9.70610859527519,4.8,73.3669019025333));
#37173=CARTESIAN_POINT('',(9.83803247244813,4.8,75.6645042434626));
#37174=CARTESIAN_POINT('',(8.91389140472481,4.8,73.3669019025333));
#37175=CARTESIAN_POINT('Origin',(9.31,4.8,77.9999999999998));
#37176=CARTESIAN_POINT('',(8.93844455602745,4.8,72.9392812237066));
#37177=CARTESIAN_POINT('',(8.79424410320319,4.8,75.4506939040492));
#37178=CARTESIAN_POINT('',(8.46441588028028,4.8,72.0598832085154));
#37179=CARTESIAN_POINT('Ctrl Pts',(8.93844455602745,4.8,72.9392812237066));
#37180=CARTESIAN_POINT('Ctrl Pts',(8.93405450155534,4.8,72.8952178225727));
#37181=CARTESIAN_POINT('Ctrl Pts',(8.91785153193323,4.8,72.8373409623484));
#37182=CARTESIAN_POINT('Ctrl Pts',(8.85769219205878,4.8,72.6555153283963));
#37183=CARTESIAN_POINT('Ctrl Pts',(8.79081812458728,4.8,72.5231469699846));
#37184=CARTESIAN_POINT('Ctrl Pts',(8.64267548147068,4.8,72.2855855384878));
#37185=CARTESIAN_POINT('Ctrl Pts',(8.56318179199311,4.8,72.1761004142322));
#37186=CARTESIAN_POINT('Ctrl Pts',(8.46441588028027,4.8,72.0598832085154));
#37187=CARTESIAN_POINT('',(8.07294956118024,4.8,72.1289092826106));
#37188=CARTESIAN_POINT('Origin',(9.31,4.8,78.));
#37189=CARTESIAN_POINT('',(7.92828014771504,4.8,73.1174004638434));
#37190=CARTESIAN_POINT('Ctrl Pts',(8.07294956118024,4.8,72.1289092826106));
#37191=CARTESIAN_POINT('Ctrl Pts',(8.01079867475487,4.8,72.2963931067747));
#37192=CARTESIAN_POINT('Ctrl Pts',(7.96245928031717,4.8,72.4681817504002));
#37193=CARTESIAN_POINT('Ctrl Pts',(7.91818215761049,4.8,72.7469888411323));
#37194=CARTESIAN_POINT('Ctrl Pts',(7.91099972253224,4.8,72.8362124135078));
#37195=CARTESIAN_POINT('Ctrl Pts',(7.9104099657788,4.8,72.9888516549209));
#37196=CARTESIAN_POINT('Ctrl Pts',(7.91537633853598,4.8,73.0668150730702));
#37197=CARTESIAN_POINT('Ctrl Pts',(7.92828014771504,4.8,73.1174004638434));
#37198=CARTESIAN_POINT('',(8.09760744867254,4.8,73.5108347879048));
#37199=CARTESIAN_POINT('',(9.00740162450745,4.8,75.6247541297977));
#37200=CARTESIAN_POINT('',(7.3531668006526,4.8,73.7817890249619));
#37201=CARTESIAN_POINT('Origin',(9.30999999999986,4.8,77.9999999999997));
#37202=CARTESIAN_POINT('',(7.22998432988738,4.8,73.3715593562453));
#37203=CARTESIAN_POINT('',(7.95343395333514,4.8,75.7808347792541));
#37204=CARTESIAN_POINT('',(6.48377124607659,4.8,72.7073228862421));
#37205=CARTESIAN_POINT('Ctrl Pts',(7.22998432988738,4.8,73.3715593562453));
#37206=CARTESIAN_POINT('Ctrl Pts',(7.21078845692561,4.8,73.3316547895226));
#37207=CARTESIAN_POINT('Ctrl Pts',(7.17576759298895,4.8,73.2828100723767));
#37208=CARTESIAN_POINT('Ctrl Pts',(7.05704827823986,4.8,73.1325255745702));
#37209=CARTESIAN_POINT('Ctrl Pts',(6.94893456556166,4.8,73.0310122828858));
#37210=CARTESIAN_POINT('Ctrl Pts',(6.72847522208608,4.8,72.858445326573));
#37211=CARTESIAN_POINT('Ctrl Pts',(6.61632947039997,4.8,72.7827514058996));
#37212=CARTESIAN_POINT('Ctrl Pts',(6.48377124607659,4.8,72.7073228862421));
#37213=CARTESIAN_POINT('',(6.13952154251132,4.8,72.9060755452598));
#37214=CARTESIAN_POINT('Origin',(9.31,4.8,78.));
#37215=CARTESIAN_POINT('',(6.34166065765632,4.8,73.8844332675354));
#37216=CARTESIAN_POINT('Ctrl Pts',(6.13952154251132,4.8,72.9060755452598));
#37217=CARTESIAN_POINT('Ctrl Pts',(6.13919026958786,4.8,72.9589189192305));
#37218=CARTESIAN_POINT('Ctrl Pts',(6.14010632567283,4.8,73.0107549229785));
#37219=CARTESIAN_POINT('Ctrl Pts',(6.14231138804498,4.8,73.0615357979665));
#37220=CARTESIAN_POINT('Ctrl Pts',(6.14407383648731,4.8,73.1021236176823));
#37221=CARTESIAN_POINT('Ctrl Pts',(6.14666119885485,4.8,73.1420393187381));
#37222=CARTESIAN_POINT('Ctrl Pts',(6.15007092616186,4.8,73.1812495953145));
#37223=CARTESIAN_POINT('Ctrl Pts',(6.15280228663195,4.8,73.2126589690911));
#37224=CARTESIAN_POINT('Ctrl Pts',(6.15606122731895,4.8,73.2436167862334));
#37225=CARTESIAN_POINT('Ctrl Pts',(6.15982585015175,4.8,73.2740739832677));
#37226=CARTESIAN_POINT('Ctrl Pts',(6.16393616428756,4.8,73.3073279513457));
#37227=CARTESIAN_POINT('Ctrl Pts',(6.16864948314967,4.8,73.3399860909232));
#37228=CARTESIAN_POINT('Ctrl Pts',(6.17390334482274,4.8,73.3719165158161));
#37229=CARTESIAN_POINT('Ctrl Pts',(6.17847047257082,4.8,73.3996733047479));
#37230=CARTESIAN_POINT('Ctrl Pts',(6.18344311440971,4.8,73.4268746768222));
#37231=CARTESIAN_POINT('Ctrl Pts',(6.18878548958805,4.8,73.4534367202513));
#37232=CARTESIAN_POINT('Ctrl Pts',(6.1931410770833,4.8,73.4750925007508));
#37233=CARTESIAN_POINT('Ctrl Pts',(6.19774195581625,4.8,73.4963222655652));
#37234=CARTESIAN_POINT('Ctrl Pts',(6.20258915775713,4.8,73.5171151933554));
#37235=CARTESIAN_POINT('Ctrl Pts',(6.20788985257399,4.8,73.5398534588348));
#37236=CARTESIAN_POINT('Ctrl Pts',(6.21348710503892,4.8,73.5620729189504));
#37237=CARTESIAN_POINT('Ctrl Pts',(6.21940732112328,4.8,73.5838035650851));
#37238=CARTESIAN_POINT('Ctrl Pts',(6.22380078545766,4.8,73.5999301417836));
#37239=CARTESIAN_POINT('Ctrl Pts',(6.22837317441562,4.8,73.6157893926149));
#37240=CARTESIAN_POINT('Ctrl Pts',(6.23312510238621,4.8,73.6313747017585));
#37241=CARTESIAN_POINT('Ctrl Pts',(6.23746789761259,4.8,73.6456181428564));
#37242=CARTESIAN_POINT('Ctrl Pts',(6.2419611776524,4.8,73.6596337213974));
#37243=CARTESIAN_POINT('Ctrl Pts',(6.2465866488109,4.8,73.6733823553783));
#37244=CARTESIAN_POINT('Ctrl Pts',(6.25127546773714,4.8,73.6873192826687));
#37245=CARTESIAN_POINT('Ctrl Pts',(6.25610033635251,4.8,73.7009822513204));
#37246=CARTESIAN_POINT('Ctrl Pts',(6.26101501047773,4.8,73.7142817032348));
#37247=CARTESIAN_POINT('Ctrl Pts',(6.26785807347238,4.8,73.7327995103013));
#37248=CARTESIAN_POINT('Ctrl Pts',(6.27487349986076,4.8,73.7506090318451));
#37249=CARTESIAN_POINT('Ctrl Pts',(6.28188818866958,4.8,73.7673849662274));
#37250=CARTESIAN_POINT('Ctrl Pts',(6.28714920527619,4.8,73.7799669170141));
#37251=CARTESIAN_POINT('Ctrl Pts',(6.29240795491918,4.8,73.7919641589943));
#37252=CARTESIAN_POINT('Ctrl Pts',(6.29759868254043,4.8,73.8032558795968));
#37253=CARTESIAN_POINT('Ctrl Pts',(6.3026125724438,4.8,73.8141629138417));
#37254=CARTESIAN_POINT('Ctrl Pts',(6.3075624751535,4.8,73.824410758489));
#37255=CARTESIAN_POINT('Ctrl Pts',(6.31241382043933,4.8,73.8339389496217));
#37256=CARTESIAN_POINT('Ctrl Pts',(6.31797885022995,4.8,73.84486883904));
#37257=CARTESIAN_POINT('Ctrl Pts',(6.32341463643833,4.8,73.8548528716026));
#37258=CARTESIAN_POINT('Ctrl Pts',(6.32870390261798,4.8,73.8638655182879));
#37259=CARTESIAN_POINT('Ctrl Pts',(6.33312440839882,4.8,73.8713978404324));
#37260=CARTESIAN_POINT('Ctrl Pts',(6.33744361862487,4.8,73.8782537232953));
#37261=CARTESIAN_POINT('Ctrl Pts',(6.34166065765632,4.8,73.8844332675354));
#37262=CARTESIAN_POINT('',(6.63533873676838,4.8,74.1962272508773));
#37263=CARTESIAN_POINT('',(8.21326860652757,4.8,75.8714937229748));
#37264=CARTESIAN_POINT('',(6.02846516020394,4.8,74.7054546451438));
#37265=CARTESIAN_POINT('Origin',(9.30999999999964,4.8,77.9999999999996));
#37266=CARTESIAN_POINT('',(5.77240469132477,4.8,74.3620957389297));
#37267=CARTESIAN_POINT('',(7.27624568947745,4.8,76.3786397314713));
#37268=CARTESIAN_POINT('',(4.84401151027683,4.8,73.9931375354699));
#37269=CARTESIAN_POINT('Ctrl Pts',(5.77240469132477,4.8,74.3620957389297));
#37270=CARTESIAN_POINT('Ctrl Pts',(5.74071830526386,4.8,74.3311630869991));
#37271=CARTESIAN_POINT('Ctrl Pts',(5.69110358025555,4.8,74.2972419075011));
#37272=CARTESIAN_POINT('Ctrl Pts',(5.52814359189328,4.8,74.1966250715416));
#37273=CARTESIAN_POINT('Ctrl Pts',(5.39183034320095,4.8,74.1382108478629));
#37274=CARTESIAN_POINT('Ctrl Pts',(5.12564495012972,4.8,74.0514524887457));
#37275=CARTESIAN_POINT('Ctrl Pts',(4.99437356897251,4.8,74.0186795759735));
#37276=CARTESIAN_POINT('Ctrl Pts',(4.84401151027683,4.8,73.9931375354699));
#37277=CARTESIAN_POINT('',(4.58850001706627,4.8,74.2976442754434));
#37278=CARTESIAN_POINT('Origin',(9.31,4.8,78.));
#37279=CARTESIAN_POINT('',(5.11306670030725,4.8,75.1478641584586));
#37280=CARTESIAN_POINT('Ctrl Pts',(4.58850001706627,4.8,74.2976442754434));
#37281=CARTESIAN_POINT('Ctrl Pts',(4.60626222068121,4.8,74.3474141060367));
#37282=CARTESIAN_POINT('Ctrl Pts',(4.6248519892365,4.8,74.3958107066347));
#37283=CARTESIAN_POINT('Ctrl Pts',(4.64429215220695,4.8,74.4427749443995));
#37284=CARTESIAN_POINT('Ctrl Pts',(4.65983016360494,4.8,74.4803122254808));
#37285=CARTESIAN_POINT('Ctrl Pts',(4.67591346239461,4.8,74.5169357844687));
#37286=CARTESIAN_POINT('Ctrl Pts',(4.69252826205227,4.8,74.5526151959383));
#37287=CARTESIAN_POINT('Ctrl Pts',(4.70583753983714,4.8,74.5811961724311));
#37288=CARTESIAN_POINT('Ctrl Pts',(4.71948813939692,4.8,74.6091723814237));
#37289=CARTESIAN_POINT('Ctrl Pts',(4.73344270257734,4.8,74.6365052079171));
#37290=CARTESIAN_POINT('Ctrl Pts',(4.74867866115537,4.8,74.6663479057422));
#37291=CARTESIAN_POINT('Ctrl Pts',(4.76427747346707,4.8,74.6954244681821));
#37292=CARTESIAN_POINT('Ctrl Pts',(4.78013533678421,4.8,74.7236323260018));
#37293=CARTESIAN_POINT('Ctrl Pts',(4.79392041401104,4.8,74.7481531262302));
#37294=CARTESIAN_POINT('Ctrl Pts',(4.80789658608741,4.8,74.7720133113463));
#37295=CARTESIAN_POINT('Ctrl Pts',(4.8220015305823,4.8,74.7951462677966));
#37296=CARTESIAN_POINT('Ctrl Pts',(4.83350115716757,4.8,74.8140063463377));
#37297=CARTESIAN_POINT('Ctrl Pts',(4.84508557617433,4.8,74.8323822065386));
#37298=CARTESIAN_POINT('Ctrl Pts',(4.85675205622014,4.8,74.8502633267103));
#37299=CARTESIAN_POINT('Ctrl Pts',(4.86951002512632,4.8,74.8698173630831));
#37300=CARTESIAN_POINT('Ctrl Pts',(4.88236922518497,4.8,74.8887824531661));
#37301=CARTESIAN_POINT('Ctrl Pts',(4.8953647275517,4.8,74.9071777482689));
#37302=CARTESIAN_POINT('Ctrl Pts',(4.90500884766322,4.8,74.9208291201398));
#37303=CARTESIAN_POINT('Ctrl Pts',(4.91472967109205,4.8,74.9341680920388));
#37304=CARTESIAN_POINT('Ctrl Pts',(4.92452551243159,4.8,74.9471882369959));
#37305=CARTESIAN_POINT('Ctrl Pts',(4.93347794881098,4.8,74.9590873700401));
#37306=CARTESIAN_POINT('Ctrl Pts',(4.94249386107474,4.8,74.970720913485));
#37307=CARTESIAN_POINT('Ctrl Pts',(4.95154269194146,4.8,74.9820583990737));
#37308=CARTESIAN_POINT('Ctrl Pts',(4.96071545031099,4.8,74.9935511562436));
#37309=CARTESIAN_POINT('Ctrl Pts',(4.96992235419727,4.8,75.0047399447727));
#37310=CARTESIAN_POINT('Ctrl Pts',(4.97908931761474,4.8,75.0155564240187));
#37311=CARTESIAN_POINT('Ctrl Pts',(4.99185315650524,4.8,75.030617005388));
#37312=CARTESIAN_POINT('Ctrl Pts',(5.00453671609312,4.8,75.0449530643228));
#37313=CARTESIAN_POINT('Ctrl Pts',(5.01686607495472,4.8,75.0583181212877));
#37314=CARTESIAN_POINT('Ctrl Pts',(5.02611309410092,4.8,75.0683419140114));
#37315=CARTESIAN_POINT('Ctrl Pts',(5.03515800080879,4.8,75.0778170355269));
#37316=CARTESIAN_POINT('Ctrl Pts',(5.0438976852005,4.8,75.0866524487053));
#37317=CARTESIAN_POINT('Ctrl Pts',(5.05233962593721,4.8,75.0951868569394));
#37318=CARTESIAN_POINT('Ctrl Pts',(5.06049598226297,4.8,75.1031237144866));
#37319=CARTESIAN_POINT('Ctrl Pts',(5.0683135889096,4.8,75.1104180275667));
#37320=CARTESIAN_POINT('Ctrl Pts',(5.07728124869061,4.8,75.1187854117285));
#37321=CARTESIAN_POINT('Ctrl Pts',(5.0858039571351,4.8,75.1263081850942));
#37322=CARTESIAN_POINT('Ctrl Pts',(5.09385674825335,4.8,75.1329682671262));
#37323=CARTESIAN_POINT('Ctrl Pts',(5.1005868709652,4.8,75.1385344327809));
#37324=CARTESIAN_POINT('Ctrl Pts',(5.10699045111816,4.8,75.1434995985332));
#37325=CARTESIAN_POINT('Ctrl Pts',(5.11306670030725,4.8,75.1478641584586));
#37326=CARTESIAN_POINT('',(5.49567364700612,4.8,75.340410845101));
#37327=CARTESIAN_POINT('',(7.55141758063195,4.8,76.3749625865681));
#37328=CARTESIAN_POINT('',(5.09956505173093,4.8,76.0264910574324));
#37329=CARTESIAN_POINT('Origin',(9.30999999999911,4.8,77.9999999999995));
#37330=CARTESIAN_POINT('',(4.7415112563347,4.8,75.7914170652479));
#37331=CARTESIAN_POINT('',(6.84435821048571,4.8,77.1720046608023));
#37332=CARTESIAN_POINT('',(3.74291589727828,4.8,75.7622389329459));
#37333=CARTESIAN_POINT('Ctrl Pts',(4.7415112563347,4.8,75.7914170652479));
#37334=CARTESIAN_POINT('Ctrl Pts',(4.70115619977021,4.8,75.7731872611718));
#37335=CARTESIAN_POINT('Ctrl Pts',(4.64293187777709,4.8,75.7582810147208));
#37336=CARTESIAN_POINT('Ctrl Pts',(4.45538660771444,4.8,75.7194677169205));
#37337=CARTESIAN_POINT('Ctrl Pts',(4.30731521231246,4.8,75.7111981783558));
#37338=CARTESIAN_POINT('Ctrl Pts',(4.02750965317559,4.8,75.7207127544803));
#37339=CARTESIAN_POINT('Ctrl Pts',(3.89294590785691,4.8,75.7348137468304));
#37340=CARTESIAN_POINT('Ctrl Pts',(3.74291589727828,4.8,75.7622389329459));
#37341=CARTESIAN_POINT('',(3.60696107145241,4.8,76.1357717469497));
#37342=CARTESIAN_POINT('Origin',(9.31,4.8,78.));
#37343=CARTESIAN_POINT('',(4.39068483903982,4.8,76.7553047249138));
#37344=CARTESIAN_POINT('Ctrl Pts',(3.60696107145242,4.8,76.1357717469498));
#37345=CARTESIAN_POINT('Ctrl Pts',(3.6406743677089,4.8,76.1764650580725));
#37346=CARTESIAN_POINT('Ctrl Pts',(3.67469564829431,4.8,76.215584911225));
#37347=CARTESIAN_POINT('Ctrl Pts',(3.70902614130493,4.8,76.253067931571));
#37348=CARTESIAN_POINT('Ctrl Pts',(3.7364656004989,4.8,76.2830271228629));
#37349=CARTESIAN_POINT('Ctrl Pts',(3.76410495085053,4.8,76.3119411971029));
#37350=CARTESIAN_POINT('Ctrl Pts',(3.79192083116205,4.8,76.3397862790184));
#37351=CARTESIAN_POINT('Ctrl Pts',(3.8142027312811,4.8,76.3620915710709));
#37352=CARTESIAN_POINT('Ctrl Pts',(3.83659852629453,4.8,76.3837118286243));
#37353=CARTESIAN_POINT('Ctrl Pts',(3.85905990391048,4.8,76.4046235426909));
#37354=CARTESIAN_POINT('Ctrl Pts',(3.88358382515552,4.8,76.4274555006248));
#37355=CARTESIAN_POINT('Ctrl Pts',(3.90818668364436,4.8,76.4494434235343));
#37356=CARTESIAN_POINT('Ctrl Pts',(3.93273585598364,4.8,76.4705264304943));
#37357=CARTESIAN_POINT('Ctrl Pts',(3.9540761991713,4.8,76.4888536717444));
#37358=CARTESIAN_POINT('Ctrl Pts',(3.97537016910973,4.8,76.5064947795499));
#37359=CARTESIAN_POINT('Ctrl Pts',(3.99653641868867,4.8,76.5234084731701));
#37360=CARTESIAN_POINT('Ctrl Pts',(4.01379305985171,4.8,76.537198046068));
#37361=CARTESIAN_POINT('Ctrl Pts',(4.0309637674028,4.8,76.5505036018421));
#37362=CARTESIAN_POINT('Ctrl Pts',(4.04804237604851,4.8,76.563316187525));
#37363=CARTESIAN_POINT('Ctrl Pts',(4.06671882044551,4.8,76.5773274895609));
#37364=CARTESIAN_POINT('Ctrl Pts',(4.08528895950369,4.8,76.5907507399687));
#37365=CARTESIAN_POINT('Ctrl Pts',(4.10379229946702,4.8,76.6035919400525));
#37366=CARTESIAN_POINT('Ctrl Pts',(4.11752385220946,4.8,76.6131215501973));
#37367=CARTESIAN_POINT('Ctrl Pts',(4.13122063540912,4.8,76.6223313663111));
#37368=CARTESIAN_POINT('Ctrl Pts',(4.14487886714958,4.8,76.6312159254611));
#37369=CARTESIAN_POINT('Ctrl Pts',(4.15736114877002,4.8,76.6393355394413));
#37370=CARTESIAN_POINT('Ctrl Pts',(4.16981224121807,4.8,76.6471838708035));
#37371=CARTESIAN_POINT('Ctrl Pts',(4.18219300928576,4.8,76.6547427399577));
#37372=CARTESIAN_POINT('Ctrl Pts',(4.19474333702386,4.8,76.6624051309092));
#37373=CARTESIAN_POINT('Ctrl Pts',(4.207221787657,4.8,76.6697702063222));
#37374=CARTESIAN_POINT('Ctrl Pts',(4.21953536925903,4.8,76.6767990859001));
#37375=CARTESIAN_POINT('Ctrl Pts',(4.23668047682952,4.8,76.6865859131902));
#37376=CARTESIAN_POINT('Ctrl Pts',(4.25350234527019,4.8,76.6957193692272));
#37377=CARTESIAN_POINT('Ctrl Pts',(4.2696592716686,4.8,76.7040615256509));
#37378=CARTESIAN_POINT('Ctrl Pts',(4.2817769664674,4.8,76.7103181429686));
#37379=CARTESIAN_POINT('Ctrl Pts',(4.29351708109353,4.8,76.7161283045197));
#37380=CARTESIAN_POINT('Ctrl Pts',(4.30475158741952,4.8,76.7214417290397));
#37381=CARTESIAN_POINT('Ctrl Pts',(4.31560335638421,4.8,76.7265741357187));
#37382=CARTESIAN_POINT('Ctrl Pts',(4.32598238941678,4.8,76.731242704048));
#37383=CARTESIAN_POINT('Ctrl Pts',(4.33582333872569,4.8,76.7354233372979));
#37384=CARTESIAN_POINT('Ctrl Pts',(4.34711199630289,4.8,76.7402189861455));
#37385=CARTESIAN_POINT('Ctrl Pts',(4.35769366250113,4.8,76.7443731427938));
#37386=CARTESIAN_POINT('Ctrl Pts',(4.36753869305379,4.8,76.7478773559685));
#37387=CARTESIAN_POINT('Ctrl Pts',(4.37576668082011,4.8,76.7508060033686));
#37388=CARTESIAN_POINT('Ctrl Pts',(4.38348226484115,4.8,76.7532815796966));
#37389=CARTESIAN_POINT('Ctrl Pts',(4.39068483903982,4.8,76.7553047249138));
#37390=CARTESIAN_POINT('',(4.81607260887647,4.8,76.805380142761));
#37391=CARTESIAN_POINT('',(7.10167754842447,4.8,77.0744349452193));
#37392=CARTESIAN_POINT('',(4.67850553742098,4.8,77.5855617740846));
#37393=CARTESIAN_POINT('Origin',(9.3100000000004,4.8,78.0000000000001));
#37394=CARTESIAN_POINT('',(4.2616449875437,4.8,77.4871260887099));
#37395=CARTESIAN_POINT('',(6.70986352030667,4.8,78.0652380479502));
#37396=CARTESIAN_POINT('',(3.31329278849671,4.8,77.8012473408872));
#37397=CARTESIAN_POINT('Ctrl Pts',(4.2616449875437,4.8,77.4871260887099));
#37398=CARTESIAN_POINT('Ctrl Pts',(4.21748867968916,4.8,77.4837979186763));
#37399=CARTESIAN_POINT('Ctrl Pts',(4.15767747875508,4.8,77.4897045193291));
#37400=CARTESIAN_POINT('Ctrl Pts',(3.9644915235101,4.8,77.5179129865806));
#37401=CARTESIAN_POINT('Ctrl Pts',(3.82580661557927,4.8,77.5619464956297));
#37402=CARTESIAN_POINT('Ctrl Pts',(3.56890774902052,4.8,77.6624620772996));
#37403=CARTESIAN_POINT('Ctrl Pts',(3.43851412071864,4.8,77.7279002925011));
#37404=CARTESIAN_POINT('Ctrl Pts',(3.31329278849671,4.8,77.8012473408872));
#37405=CARTESIAN_POINT('Origin',(9.31,4.8,78.));
#37406=CARTESIAN_POINT('Origin',(9.31,9.325,78.));
#37407=CARTESIAN_POINT('',(3.06,13.85,78.));
#37408=CARTESIAN_POINT('',(3.06,9.325,78.));
#37409=CARTESIAN_POINT('Origin',(9.31,13.85,78.));
#37410=CARTESIAN_POINT('Origin',(12.21,23.,78.));
#37411=CARTESIAN_POINT('',(6.41,23.,78.));
#37412=CARTESIAN_POINT('Origin',(9.31,23.,78.));
#37413=CARTESIAN_POINT('Origin',(9.31,22.95,78.));
#37414=CARTESIAN_POINT('',(6.31,22.9,78.));
#37415=CARTESIAN_POINT('Origin',(9.31,22.9,78.));
#37416=CARTESIAN_POINT('',(6.36,22.95,78.));
#37417=CARTESIAN_POINT('Origin',(9.31,18.45,78.));
#37418=CARTESIAN_POINT('',(6.31,14.,78.));
#37419=CARTESIAN_POINT('Origin',(9.31,14.,78.));
#37420=CARTESIAN_POINT('',(6.31,18.45,78.));
#37421=CARTESIAN_POINT('Origin',(15.41,14.,78.));
#37422=CARTESIAN_POINT('',(3.21,14.,78.));
#37423=CARTESIAN_POINT('Origin',(9.31,14.,78.));
#37424=CARTESIAN_POINT('Origin',(9.31,13.925,78.));
#37425=CARTESIAN_POINT('',(3.135,13.925,78.));
#37426=CARTESIAN_POINT('Origin',(9.31,-13.925,78.));
#37427=CARTESIAN_POINT('',(3.21,-14.,78.));
#37428=CARTESIAN_POINT('Origin',(9.31,-14.,78.));
#37429=CARTESIAN_POINT('',(3.135,-13.925,78.));
#37430=CARTESIAN_POINT('Origin',(12.31,-14.,78.));
#37431=CARTESIAN_POINT('',(6.31,-14.,78.));
#37432=CARTESIAN_POINT('Origin',(9.31,-14.,78.));
#37433=CARTESIAN_POINT('Origin',(9.31,-16.2,78.));
#37434=CARTESIAN_POINT('',(6.31,-18.4,78.));
#37435=CARTESIAN_POINT('Origin',(9.31,-18.4,78.));
#37436=CARTESIAN_POINT('',(6.31,-16.2,78.));
#37437=CARTESIAN_POINT('Origin',(9.31,-18.45,78.));
#37438=CARTESIAN_POINT('',(6.41,-18.5,78.));
#37439=CARTESIAN_POINT('Origin',(9.31,-18.5,78.));
#37440=CARTESIAN_POINT('',(6.36,-18.45,78.));
#37441=CARTESIAN_POINT('Origin',(9.31,-18.5,78.));
#37442=CARTESIAN_POINT('Ctrl Pts',(4.55037293434634,-5.,81.8152261002327));
#37443=CARTESIAN_POINT('Ctrl Pts',(4.55037293434634,5.,81.8152261002327));
#37444=CARTESIAN_POINT('Ctrl Pts',(4.55326576923268,-5.,81.8061728189788));
#37445=CARTESIAN_POINT('Ctrl Pts',(4.55326576923268,5.,81.8061728189788));
#37446=CARTESIAN_POINT('Ctrl Pts',(4.55909298521487,-5.,81.7881352345572));
#37447=CARTESIAN_POINT('Ctrl Pts',(4.55909298521487,5.,81.7881352345572));
#37448=CARTESIAN_POINT('Ctrl Pts',(4.56795844777182,-5.,81.7612857920655));
#37449=CARTESIAN_POINT('Ctrl Pts',(4.56795844777182,5.,81.7612857920655));
#37450=CARTESIAN_POINT('Ctrl Pts',(4.5800287934221,-5.,81.7259011540785));
#37451=CARTESIAN_POINT('Ctrl Pts',(4.5800287934221,5.,81.7259011540785));
#37452=CARTESIAN_POINT('Ctrl Pts',(4.59553572302973,-5.,81.6823663399517));
#37453=CARTESIAN_POINT('Ctrl Pts',(4.59553572302973,5.,81.6823663399517));
#37454=CARTESIAN_POINT('Ctrl Pts',(4.61146542604692,-5.,81.6395347836739));
#37455=CARTESIAN_POINT('Ctrl Pts',(4.61146542604692,5.,81.6395347836739));
#37456=CARTESIAN_POINT('Ctrl Pts',(4.62782195277065,-5.,81.5974152138272));
#37457=CARTESIAN_POINT('Ctrl Pts',(4.62782195277065,5.,81.5974152138272));
#37458=CARTESIAN_POINT('Ctrl Pts',(4.64460884258077,-5.,81.5560168849901));
#37459=CARTESIAN_POINT('Ctrl Pts',(4.64460884258077,5.,81.5560168849901));
#37460=CARTESIAN_POINT('Ctrl Pts',(4.66182827725197,-5.,81.51534844747));
#37461=CARTESIAN_POINT('Ctrl Pts',(4.66182827725197,5.,81.51534844747));
#37462=CARTESIAN_POINT('Ctrl Pts',(4.6794801351961,-5.,81.4754169688554));
#37463=CARTESIAN_POINT('Ctrl Pts',(4.6794801351961,5.,81.4754169688554));
#37464=CARTESIAN_POINT('Ctrl Pts',(4.69756020902606,-5.,81.4362308703527));
#37465=CARTESIAN_POINT('Ctrl Pts',(4.69756020902606,5.,81.4362308703527));
#37466=CARTESIAN_POINT('Ctrl Pts',(4.71605851282859,-5.,81.397802395678));
#37467=CARTESIAN_POINT('Ctrl Pts',(4.71605851282859,5.,81.397802395678));
#37468=CARTESIAN_POINT('Ctrl Pts',(4.73495715972825,-5.,81.3601503543456));
#37469=CARTESIAN_POINT('Ctrl Pts',(4.73495715972825,5.,81.3601503543456));
#37470=CARTESIAN_POINT('Ctrl Pts',(4.7542288770199,-5.,81.3233020975585));
#37471=CARTESIAN_POINT('Ctrl Pts',(4.7542288770199,5.,81.3233020975585));
#37472=CARTESIAN_POINT('Ctrl Pts',(4.77383361228162,-5.,81.2872970095592));
#37473=CARTESIAN_POINT('Ctrl Pts',(4.77383361228162,5.,81.2872970095592));
#37474=CARTESIAN_POINT('Ctrl Pts',(4.79372122786719,-5.,81.2521844855106));
#37475=CARTESIAN_POINT('Ctrl Pts',(4.79372122786719,5.,81.2521844855106));
#37476=CARTESIAN_POINT('Ctrl Pts',(4.81384166090125,-5.,81.2180152029093));
#37477=CARTESIAN_POINT('Ctrl Pts',(4.81384166090125,5.,81.2180152029093));
#37478=CARTESIAN_POINT('Ctrl Pts',(4.8341534505068,-5.,81.184833647465));
#37479=CARTESIAN_POINT('Ctrl Pts',(4.8341534505068,5.,81.184833647465));
#37480=CARTESIAN_POINT('Ctrl Pts',(4.85463221422933,-5.,81.152670529545));
#37481=CARTESIAN_POINT('Ctrl Pts',(4.85463221422933,5.,81.152670529545));
#37482=CARTESIAN_POINT('Ctrl Pts',(4.87528087827813,-5.,81.1215334547639));
#37483=CARTESIAN_POINT('Ctrl Pts',(4.87528087827813,5.,81.1215334547639));
#37484=CARTESIAN_POINT('Ctrl Pts',(4.89613444857731,-5.,81.091402307974));
#37485=CARTESIAN_POINT('Ctrl Pts',(4.89613444857731,5.,81.091402307974));
#37486=CARTESIAN_POINT('Ctrl Pts',(4.91722853182858,-5.,81.0622569233023));
#37487=CARTESIAN_POINT('Ctrl Pts',(4.91722853182858,5.,81.0622569233023));
#37488=CARTESIAN_POINT('Ctrl Pts',(4.93857071576868,-5.,81.0341019923514));
#37489=CARTESIAN_POINT('Ctrl Pts',(4.93857071576868,5.,81.0341019923514));
#37490=CARTESIAN_POINT('Ctrl Pts',(4.96011273429653,-5.,81.0069911329727));
#37491=CARTESIAN_POINT('Ctrl Pts',(4.96011273429653,5.,81.0069911329727));
#37492=CARTESIAN_POINT('Ctrl Pts',(4.98171699052596,-5.,80.981055696686));
#37493=CARTESIAN_POINT('Ctrl Pts',(4.98171699052596,5.,80.981055696686));
#37494=CARTESIAN_POINT('Ctrl Pts',(5.00313954967413,-5.,80.9565189839515));
#37495=CARTESIAN_POINT('Ctrl Pts',(5.00313954967413,5.,80.9565189839515));
#37496=CARTESIAN_POINT('Ctrl Pts',(5.02408529635557,-5.,80.9336473146961));
#37497=CARTESIAN_POINT('Ctrl Pts',(5.02408529635557,5.,80.9336473146961));
#37498=CARTESIAN_POINT('Ctrl Pts',(5.0442546199981,-5.,80.9127081471617));
#37499=CARTESIAN_POINT('Ctrl Pts',(5.0442546199981,5.,80.9127081471617));
#37500=CARTESIAN_POINT('Ctrl Pts',(5.06338898078167,-5.,80.8939293165779));
#37501=CARTESIAN_POINT('Ctrl Pts',(5.06338898078167,5.,80.8939293165779));
#37502=CARTESIAN_POINT('Ctrl Pts',(5.0813283019591,-5.,80.8774468502762));
#37503=CARTESIAN_POINT('Ctrl Pts',(5.0813283019591,5.,80.8774468502762));
#37504=CARTESIAN_POINT('Ctrl Pts',(5.09466658957796,-5.,80.8661420261577));
#37505=CARTESIAN_POINT('Ctrl Pts',(5.09466658957796,5.,80.8661420261577));
#37506=CARTESIAN_POINT('Ctrl Pts',(5.10409134141797,-5.,80.8587263580475));
#37507=CARTESIAN_POINT('Ctrl Pts',(5.10409134141797,5.,80.8587263580475));
#37508=CARTESIAN_POINT('Ctrl Pts',(5.11011771525274,-5.,80.8542540927006));
#37509=CARTESIAN_POINT('Ctrl Pts',(5.11011771525274,5.,80.8542540927006));
#37510=CARTESIAN_POINT('Ctrl Pts',(5.11306670030725,-5.,80.8521358415414));
#37511=CARTESIAN_POINT('Ctrl Pts',(5.11306670030725,5.,80.8521358415414));
#37512=CARTESIAN_POINT('',(5.11306670030725,0.,80.8521358415414));
#37513=CARTESIAN_POINT('Ctrl Pts',(4.58850001701745,4.8,81.7023557244943));
#37514=CARTESIAN_POINT('Ctrl Pts',(4.58850001701745,3.13333333333333,81.7023557244943));
#37515=CARTESIAN_POINT('Ctrl Pts',(4.58850001701745,1.46666666666667,81.7023557244943));
#37516=CARTESIAN_POINT('Ctrl Pts',(4.58850001701745,-1.73333333333333,81.7023557244943));
#37517=CARTESIAN_POINT('Ctrl Pts',(4.58850001701746,-3.26666666666667,81.7023557244943));
#37518=CARTESIAN_POINT('Ctrl Pts',(4.58850001701746,-4.8,81.7023557244943));
#37519=CARTESIAN_POINT('Origin',(9.30999999999911,0.,78.0000000000005));
#37520=CARTESIAN_POINT('',(5.09956505173093,0.,79.9735089425676));
#37521=CARTESIAN_POINT('',(5.49567364700612,0.,80.659589154899));
#37522=CARTESIAN_POINT('Origin',(5.11306670030725,0.,80.8521358415414));
#37523=CARTESIAN_POINT('Ctrl Pts',(4.7415112563347,-5.,80.2085829347521));
#37524=CARTESIAN_POINT('Ctrl Pts',(4.7415112563347,5.,80.2085829347521));
#37525=CARTESIAN_POINT('Ctrl Pts',(4.73820230448305,-5.,80.2100777051253));
#37526=CARTESIAN_POINT('Ctrl Pts',(4.73820230448305,5.,80.2100777051253));
#37527=CARTESIAN_POINT('Ctrl Pts',(4.73131602214839,-5.,80.2130605652534));
#37528=CARTESIAN_POINT('Ctrl Pts',(4.73131602214839,5.,80.2130605652534));
#37529=CARTESIAN_POINT('Ctrl Pts',(4.72018148924741,-5.,80.2175148056905));
#37530=CARTESIAN_POINT('Ctrl Pts',(4.72018148924741,5.,80.2175148056905));
#37531=CARTESIAN_POINT('Ctrl Pts',(4.70372208056832,-5.,80.2234136895571));
#37532=CARTESIAN_POINT('Ctrl Pts',(4.70372208056832,5.,80.2234136895571));
#37533=CARTESIAN_POINT('Ctrl Pts',(4.68047818546464,-5.,80.2307083643155));
#37534=CARTESIAN_POINT('Ctrl Pts',(4.68047818546464,5.,80.2307083643155));
#37535=CARTESIAN_POINT('Ctrl Pts',(4.65464806075414,-5.,80.2378897915926));
#37536=CARTESIAN_POINT('Ctrl Pts',(4.65464806075414,5.,80.2378897915926));
#37537=CARTESIAN_POINT('Ctrl Pts',(4.62642954792474,-5.,80.2448873545015));
#37538=CARTESIAN_POINT('Ctrl Pts',(4.62642954792474,5.,80.2448873545015));
#37539=CARTESIAN_POINT('Ctrl Pts',(4.59614922798182,-5.,80.2515910686015));
#37540=CARTESIAN_POINT('Ctrl Pts',(4.59614922798182,5.,80.2515910686015));
#37541=CARTESIAN_POINT('Ctrl Pts',(4.56418853184677,-5.,80.2578751926538));
#37542=CARTESIAN_POINT('Ctrl Pts',(4.56418853184677,5.,80.2578751926538));
#37543=CARTESIAN_POINT('Ctrl Pts',(4.53092565703995,-5.,80.263617309213));
#37544=CARTESIAN_POINT('Ctrl Pts',(4.53092565703995,5.,80.263617309213));
#37545=CARTESIAN_POINT('Ctrl Pts',(4.49667595482943,-5.,80.2687178148024));
#37546=CARTESIAN_POINT('Ctrl Pts',(4.49667595482943,5.,80.2687178148024));
#37547=CARTESIAN_POINT('Ctrl Pts',(4.46162197741276,-5.,80.2731232227872));
#37548=CARTESIAN_POINT('Ctrl Pts',(4.46162197741276,5.,80.2731232227872));
#37549=CARTESIAN_POINT('Ctrl Pts',(4.42583429226076,-5.,80.2768185424213));
#37550=CARTESIAN_POINT('Ctrl Pts',(4.42583429226076,5.,80.2768185424213));
#37551=CARTESIAN_POINT('Ctrl Pts',(4.38931316854944,-5.,80.2798126906734));
#37552=CARTESIAN_POINT('Ctrl Pts',(4.38931316854944,5.,80.2798126906734));
#37553=CARTESIAN_POINT('Ctrl Pts',(4.35202333876695,-5.,80.2821264209091));
#37554=CARTESIAN_POINT('Ctrl Pts',(4.35202333876695,5.,80.2821264209091));
#37555=CARTESIAN_POINT('Ctrl Pts',(4.31392987972062,-5.,80.28377999157));
#37556=CARTESIAN_POINT('Ctrl Pts',(4.31392987972062,5.,80.28377999157));
#37557=CARTESIAN_POINT('Ctrl Pts',(4.27503791496249,-5.,80.2847797396365));
#37558=CARTESIAN_POINT('Ctrl Pts',(4.27503791496249,5.,80.2847797396365));
#37559=CARTESIAN_POINT('Ctrl Pts',(4.23538623168037,-5.,80.2851199044714));
#37560=CARTESIAN_POINT('Ctrl Pts',(4.23538623168037,5.,80.2851199044714));
#37561=CARTESIAN_POINT('Ctrl Pts',(4.19503408606993,-5.,80.2847868227625));
#37562=CARTESIAN_POINT('Ctrl Pts',(4.19503408606993,5.,80.2847868227625));
#37563=CARTESIAN_POINT('Ctrl Pts',(4.15405039756986,-5.,80.2837624775403));
#37564=CARTESIAN_POINT('Ctrl Pts',(4.15405039756986,5.,80.2837624775403));
#37565=CARTESIAN_POINT('Ctrl Pts',(4.1125030124698,-5.,80.282028145913));
#37566=CARTESIAN_POINT('Ctrl Pts',(4.1125030124698,5.,80.282028145913));
#37567=CARTESIAN_POINT('Ctrl Pts',(4.07044606473299,-5.,80.2795688335823));
#37568=CARTESIAN_POINT('Ctrl Pts',(4.07044606473299,5.,80.2795688335823));
#37569=CARTESIAN_POINT('Ctrl Pts',(4.02791687754441,-5.,80.2763745972855));
#37570=CARTESIAN_POINT('Ctrl Pts',(4.02791687754441,5.,80.2763745972855));
#37571=CARTESIAN_POINT('Ctrl Pts',(3.98494068385443,-5.,80.2724393512809));
#37572=CARTESIAN_POINT('Ctrl Pts',(3.98494068385443,5.,80.2724393512809));
#37573=CARTESIAN_POINT('Ctrl Pts',(3.94153307998497,-5.,80.267760569364));
#37574=CARTESIAN_POINT('Ctrl Pts',(3.94153307998497,5.,80.267760569364));
#37575=CARTESIAN_POINT('Ctrl Pts',(3.89770346260675,-5.,80.2623388184301));
#37576=CARTESIAN_POINT('Ctrl Pts',(3.89770346260675,5.,80.2623388184301));
#37577=CARTESIAN_POINT('Ctrl Pts',(3.85345801322638,-5.,80.2561775269785));
#37578=CARTESIAN_POINT('Ctrl Pts',(3.85345801322638,5.,80.2561775269785));
#37579=CARTESIAN_POINT('Ctrl Pts',(3.80880313234891,-5.,80.249282909649));
#37580=CARTESIAN_POINT('Ctrl Pts',(3.80880313234891,5.,80.249282909649));
#37581=CARTESIAN_POINT('Ctrl Pts',(3.76374506499486,-5.,80.2416626589451));
#37582=CARTESIAN_POINT('Ctrl Pts',(3.76374506499486,5.,80.2416626589451));
#37583=CARTESIAN_POINT('Ctrl Pts',(3.71828934520081,-5.,80.2333246468413));
#37584=CARTESIAN_POINT('Ctrl Pts',(3.71828934520081,5.,80.2333246468413));
#37585=CARTESIAN_POINT('Ctrl Pts',(3.68161017699181,-5.,80.2260855538483));
#37586=CARTESIAN_POINT('Ctrl Pts',(3.68161017699181,5.,80.2260855538483));
#37587=CARTESIAN_POINT('Ctrl Pts',(3.65392514646726,-5.,80.220338548454));
#37588=CARTESIAN_POINT('Ctrl Pts',(3.65392514646726,5.,80.220338548454));
#37589=CARTESIAN_POINT('Ctrl Pts',(3.63539053217137,-5.,80.2163662733738));
#37590=CARTESIAN_POINT('Ctrl Pts',(3.63539053217137,5.,80.2163662733738));
#37591=CARTESIAN_POINT('Ctrl Pts',(3.62610374319018,-5.,80.2143449012797));
#37592=CARTESIAN_POINT('Ctrl Pts',(3.62610374319018,5.,80.2143449012797));
#37593=CARTESIAN_POINT('Ctrl Pts',(3.74291589718233,-4.8,80.2377610668154));
#37594=CARTESIAN_POINT('Ctrl Pts',(3.74291589718233,-3.13333333333333,80.2377610668154));
#37595=CARTESIAN_POINT('Ctrl Pts',(3.74291589718233,-1.46666666666667,80.2377610668154));
#37596=CARTESIAN_POINT('Ctrl Pts',(3.74291589718233,1.73333333333333,80.2377610668154));
#37597=CARTESIAN_POINT('Ctrl Pts',(3.74291589718234,3.26666666666667,80.2377610668154));
#37598=CARTESIAN_POINT('Ctrl Pts',(3.74291589718234,4.8,80.2377610668154));
#37599=CARTESIAN_POINT('',(4.7415112563347,0.,80.2085829347521));
#37600=CARTESIAN_POINT('Origin',(5.09956505173093,0.,79.9735089425676));
#37601=CARTESIAN_POINT('Ctrl Pts',(8.11629420041964,-5.,83.9820620578567));
#37602=CARTESIAN_POINT('Ctrl Pts',(8.11629420041964,5.,83.9820620578567));
#37603=CARTESIAN_POINT('Ctrl Pts',(8.11269090350116,-5.,83.9732673636178));
#37604=CARTESIAN_POINT('Ctrl Pts',(8.11269090350116,5.,83.9732673636178));
#37605=CARTESIAN_POINT('Ctrl Pts',(8.10556047416415,-5.,83.9557041100362));
#37606=CARTESIAN_POINT('Ctrl Pts',(8.10556047416415,5.,83.9557041100362));
#37607=CARTESIAN_POINT('Ctrl Pts',(8.09509332354789,-5.,83.9294376342902));
#37608=CARTESIAN_POINT('Ctrl Pts',(8.09509332354789,5.,83.9294376342902));
#37609=CARTESIAN_POINT('Ctrl Pts',(8.0815949378981,-5.,83.8945727603373));
#37610=CARTESIAN_POINT('Ctrl Pts',(8.0815949378981,5.,83.8945727603373));
#37611=CARTESIAN_POINT('Ctrl Pts',(8.06549029603877,-5.,83.8512554956866));
#37612=CARTESIAN_POINT('Ctrl Pts',(8.06549029603877,5.,83.8512554956866));
#37613=CARTESIAN_POINT('Ctrl Pts',(8.05016156282195,-5.,83.8082052043177));
#37614=CARTESIAN_POINT('Ctrl Pts',(8.05016156282195,5.,83.8082052043177));
#37615=CARTESIAN_POINT('Ctrl Pts',(8.03561745158609,-5.,83.7654259692167));
#37616=CARTESIAN_POINT('Ctrl Pts',(8.03561745158609,5.,83.7654259692167));
#37617=CARTESIAN_POINT('Ctrl Pts',(8.0218666223879,-5.,83.7229226047198));
#37618=CARTESIAN_POINT('Ctrl Pts',(8.0218666223879,5.,83.7229226047198));
#37619=CARTESIAN_POINT('Ctrl Pts',(8.00891630687788,-5.,83.6807003349195));
#37620=CARTESIAN_POINT('Ctrl Pts',(8.00891630687788,5.,83.6807003349195));
#37621=CARTESIAN_POINT('Ctrl Pts',(7.9967709548731,-5.,83.6387646520556));
#37622=CARTESIAN_POINT('Ctrl Pts',(7.9967709548731,5.,83.6387646520556));
#37623=CARTESIAN_POINT('Ctrl Pts',(7.98543275637429,-5.,83.597124711605));
#37624=CARTESIAN_POINT('Ctrl Pts',(7.98543275637429,5.,83.597124711605));
#37625=CARTESIAN_POINT('Ctrl Pts',(7.97490193183486,-5.,83.555796311625));
#37626=CARTESIAN_POINT('Ctrl Pts',(7.97490193183486,5.,83.555796311625));
#37627=CARTESIAN_POINT('Ctrl Pts',(7.96517686963337,-5.,83.5148053585083));
#37628=CARTESIAN_POINT('Ctrl Pts',(7.96517686963337,5.,83.5148053585083));
#37629=CARTESIAN_POINT('Ctrl Pts',(7.95625425867753,-5.,83.4741903350539));
#37630=CARTESIAN_POINT('Ctrl Pts',(7.95625425867753,5.,83.4741903350539));
#37631=CARTESIAN_POINT('Ctrl Pts',(7.94812873273393,-5.,83.4340071565454));
#37632=CARTESIAN_POINT('Ctrl Pts',(7.94812873273393,5.,83.4340071565454));
#37633=CARTESIAN_POINT('Ctrl Pts',(7.94079363473637,-5.,83.3943258897297));
#37634=CARTESIAN_POINT('Ctrl Pts',(7.94079363473637,5.,83.3943258897297));
#37635=CARTESIAN_POINT('Ctrl Pts',(7.93424318916526,-5.,83.3552175356154));
#37636=CARTESIAN_POINT('Ctrl Pts',(7.93424318916526,5.,83.3552175356154));
#37637=CARTESIAN_POINT('Ctrl Pts',(7.9284742300107,-5.,83.3167428227687));
#37638=CARTESIAN_POINT('Ctrl Pts',(7.9284742300107,5.,83.3167428227687));
#37639=CARTESIAN_POINT('Ctrl Pts',(7.92348781947404,-5.,83.2789409494337));
#37640=CARTESIAN_POINT('Ctrl Pts',(7.92348781947404,5.,83.2789409494337));
#37641=CARTESIAN_POINT('Ctrl Pts',(7.91929108795717,-5.,83.2418158609173));
#37642=CARTESIAN_POINT('Ctrl Pts',(7.91929108795717,5.,83.2418158609173));
#37643=CARTESIAN_POINT('Ctrl Pts',(7.91589792178468,-5.,83.2053296467483));
#37644=CARTESIAN_POINT('Ctrl Pts',(7.91589792178468,5.,83.2053296467483));
#37645=CARTESIAN_POINT('Ctrl Pts',(7.9133226348972,-5.,83.1694439714255));
#37646=CARTESIAN_POINT('Ctrl Pts',(7.9133226348972,5.,83.1694439714255));
#37647=CARTESIAN_POINT('Ctrl Pts',(7.91157405554035,-5.,83.1341575516226));
#37648=CARTESIAN_POINT('Ctrl Pts',(7.91157405554035,5.,83.1341575516226));
#37649=CARTESIAN_POINT('Ctrl Pts',(7.91064967462546,-5.,83.0995424858489));
#37650=CARTESIAN_POINT('Ctrl Pts',(7.91064967462546,5.,83.0995424858489));
#37651=CARTESIAN_POINT('Ctrl Pts',(7.91052851795315,-5.,83.0657878407806));
#37652=CARTESIAN_POINT('Ctrl Pts',(7.91052851795315,5.,83.0657878407806));
#37653=CARTESIAN_POINT('Ctrl Pts',(7.91116725541189,-5.,83.0332214727501));
#37654=CARTESIAN_POINT('Ctrl Pts',(7.91116725541189,5.,83.0332214727501));
#37655=CARTESIAN_POINT('Ctrl Pts',(7.91251100265399,-5.,83.00223709117));
#37656=CARTESIAN_POINT('Ctrl Pts',(7.91251100265399,5.,83.00223709117));
#37657=CARTESIAN_POINT('Ctrl Pts',(7.91450216351211,-5.,82.9732321669035));
#37658=CARTESIAN_POINT('Ctrl Pts',(7.91450216351211,5.,82.9732321669035));
#37659=CARTESIAN_POINT('Ctrl Pts',(7.91708913465533,-5.,82.9465474180553));
#37660=CARTESIAN_POINT('Ctrl Pts',(7.91708913465533,5.,82.9465474180553));
#37661=CARTESIAN_POINT('Ctrl Pts',(7.92023672685611,-5.,82.9223899429567));
#37662=CARTESIAN_POINT('Ctrl Pts',(7.92023672685611,5.,82.9223899429567));
#37663=CARTESIAN_POINT('Ctrl Pts',(7.92318784709605,-5.,82.9051562592444));
#37664=CARTESIAN_POINT('Ctrl Pts',(7.92318784709605,5.,82.9051562592444));
#37665=CARTESIAN_POINT('Ctrl Pts',(7.92564092628298,-5.,82.8934174141896));
#37666=CARTESIAN_POINT('Ctrl Pts',(7.92564092628298,5.,82.8934174141896));
#37667=CARTESIAN_POINT('Ctrl Pts',(7.92738267970764,-5.,82.8861177817404));
#37668=CARTESIAN_POINT('Ctrl Pts',(7.92738267970764,5.,82.8861177817404));
#37669=CARTESIAN_POINT('Ctrl Pts',(7.92828014771505,-5.,82.8825995361566));
#37670=CARTESIAN_POINT('Ctrl Pts',(7.92828014771505,5.,82.8825995361566));
#37671=CARTESIAN_POINT('',(7.92828014771505,0.,82.8825995361566));
#37672=CARTESIAN_POINT('Ctrl Pts',(8.07294956130202,4.8,83.871090717415));
#37673=CARTESIAN_POINT('Ctrl Pts',(8.07294956130202,3.13333333333333,83.871090717415));
#37674=CARTESIAN_POINT('Ctrl Pts',(8.07294956130202,1.46666666666667,83.871090717415));
#37675=CARTESIAN_POINT('Ctrl Pts',(8.07294956130202,-1.73333333333333,83.871090717415));
#37676=CARTESIAN_POINT('Ctrl Pts',(8.07294956130202,-3.26666666666667,83.871090717415));
#37677=CARTESIAN_POINT('Ctrl Pts',(8.07294956130202,-4.8,83.871090717415));
#37678=CARTESIAN_POINT('Origin',(9.31000000000056,0.,77.9999999999986));
#37679=CARTESIAN_POINT('',(7.3531668006526,0.,82.2182109750381));
#37680=CARTESIAN_POINT('',(8.09760744867255,0.,82.4891652120952));
#37681=CARTESIAN_POINT('Origin',(7.92828014771505,0.,82.8825995361566));
#37682=CARTESIAN_POINT('Ctrl Pts',(7.22998432988738,-5.,82.6284406437547));
#37683=CARTESIAN_POINT('Ctrl Pts',(7.22998432988738,5.,82.6284406437547));
#37684=CARTESIAN_POINT('Ctrl Pts',(7.22841034559216,-5.,82.6317126575429));
#37685=CARTESIAN_POINT('Ctrl Pts',(7.22841034559216,5.,82.6317126575429));
#37686=CARTESIAN_POINT('Ctrl Pts',(7.22505249282082,-5.,82.6384240779281));
#37687=CARTESIAN_POINT('Ctrl Pts',(7.22505249282082,5.,82.6384240779281));
#37688=CARTESIAN_POINT('Ctrl Pts',(7.21938607633931,-5.,82.64899336385));
#37689=CARTESIAN_POINT('Ctrl Pts',(7.21938607633931,5.,82.64899336385));
#37690=CARTESIAN_POINT('Ctrl Pts',(7.21056916724215,-5.,82.6640920750187));
#37691=CARTESIAN_POINT('Ctrl Pts',(7.21056916724215,5.,82.6640920750187));
#37692=CARTESIAN_POINT('Ctrl Pts',(7.19745223709537,-5.,82.6846210078579));
#37693=CARTESIAN_POINT('Ctrl Pts',(7.19745223709537,5.,82.6846210078579));
#37694=CARTESIAN_POINT('Ctrl Pts',(7.18228134605083,-5.,82.7067255844406));
#37695=CARTESIAN_POINT('Ctrl Pts',(7.18228134605083,5.,82.7067255844406));
#37696=CARTESIAN_POINT('Ctrl Pts',(7.16516265783049,-5.,82.7302245390343));
#37697=CARTESIAN_POINT('Ctrl Pts',(7.16516265783049,5.,82.7302245390343));
#37698=CARTESIAN_POINT('Ctrl Pts',(7.14627565136447,-5.,82.754823696445));
#37699=CARTESIAN_POINT('Ctrl Pts',(7.14627565136447,5.,82.754823696445));
#37700=CARTESIAN_POINT('Ctrl Pts',(7.12583169477743,-5.,82.7801815542262));
#37701=CARTESIAN_POINT('Ctrl Pts',(7.12583169477743,5.,82.7801815542262));
#37702=CARTESIAN_POINT('Ctrl Pts',(7.1040418157563,-5.,82.8059612344958));
#37703=CARTESIAN_POINT('Ctrl Pts',(7.1040418157563,5.,82.8059612344958));
#37704=CARTESIAN_POINT('Ctrl Pts',(7.08108356350195,-5.,82.8318837326766));
#37705=CARTESIAN_POINT('Ctrl Pts',(7.08108356350195,5.,82.8318837326766));
#37706=CARTESIAN_POINT('Ctrl Pts',(7.05706240056282,-5.,82.8577907333377));
#37707=CARTESIAN_POINT('Ctrl Pts',(7.05706240056282,5.,82.8577907333377));
#37708=CARTESIAN_POINT('Ctrl Pts',(7.03202274889278,-5.,82.883625393005));
#37709=CARTESIAN_POINT('Ctrl Pts',(7.03202274889278,5.,82.883625393005));
#37710=CARTESIAN_POINT('Ctrl Pts',(7.00597054641171,-5.,82.9093943694487));
#37711=CARTESIAN_POINT('Ctrl Pts',(7.00597054641171,5.,82.9093943694487));
#37712=CARTESIAN_POINT('Ctrl Pts',(6.97889211664698,-5.,82.9351362301886));
#37713=CARTESIAN_POINT('Ctrl Pts',(6.97889211664698,5.,82.9351362301886));
#37714=CARTESIAN_POINT('Ctrl Pts',(6.95077372875796,-5.,82.9608889422872));
#37715=CARTESIAN_POINT('Ctrl Pts',(6.95077372875796,5.,82.9608889422872));
#37716=CARTESIAN_POINT('Ctrl Pts',(6.92162338094528,-5.,82.9866540667982));
#37717=CARTESIAN_POINT('Ctrl Pts',(6.92162338094528,5.,82.9866540667982));
#37718=CARTESIAN_POINT('Ctrl Pts',(6.89146708305081,-5.,83.012402258895));
#37719=CARTESIAN_POINT('Ctrl Pts',(6.89146708305081,5.,83.012402258895));
#37720=CARTESIAN_POINT('Ctrl Pts',(6.86034144534373,-5.,83.0380849627259));
#37721=CARTESIAN_POINT('Ctrl Pts',(6.86034144534373,5.,83.0380849627259));
#37722=CARTESIAN_POINT('Ctrl Pts',(6.82828768209046,-5.,83.0636440759307));
#37723=CARTESIAN_POINT('Ctrl Pts',(6.82828768209046,5.,83.0636440759307));
#37724=CARTESIAN_POINT('Ctrl Pts',(6.7953457317203,-5.,83.0890216451884));
#37725=CARTESIAN_POINT('Ctrl Pts',(6.7953457317203,5.,83.0890216451884));
#37726=CARTESIAN_POINT('Ctrl Pts',(6.76154742510777,-5.,83.1141713875575));
#37727=CARTESIAN_POINT('Ctrl Pts',(6.76154742510777,5.,83.1141713875575));
#37728=CARTESIAN_POINT('Ctrl Pts',(6.72691496206891,-5.,83.1390616951735));
#37729=CARTESIAN_POINT('Ctrl Pts',(6.72691496206891,5.,83.1390616951735));
#37730=CARTESIAN_POINT('Ctrl Pts',(6.6914637603302,-5.,83.1636716866569));
#37731=CARTESIAN_POINT('Ctrl Pts',(6.6914637603302,5.,83.1636716866569));
#37732=CARTESIAN_POINT('Ctrl Pts',(6.65520414355774,-5.,83.1879894016978));
#37733=CARTESIAN_POINT('Ctrl Pts',(6.65520414355774,5.,83.1879894016978));
#37734=CARTESIAN_POINT('Ctrl Pts',(6.61814367441389,-5.,83.2120092344991));
#37735=CARTESIAN_POINT('Ctrl Pts',(6.61814367441389,5.,83.2120092344991));
#37736=CARTESIAN_POINT('Ctrl Pts',(6.58028929200272,-5.,83.2357298380487));
#37737=CARTESIAN_POINT('Ctrl Pts',(6.58028929200272,5.,83.2357298380487));
#37738=CARTESIAN_POINT('Ctrl Pts',(6.54164989408328,-5.,83.259151858876));
#37739=CARTESIAN_POINT('Ctrl Pts',(6.54164989408328,5.,83.259151858876));
#37740=CARTESIAN_POINT('Ctrl Pts',(6.50223520925582,-5.,83.282277175565));
#37741=CARTESIAN_POINT('Ctrl Pts',(6.50223520925582,5.,83.282277175565));
#37742=CARTESIAN_POINT('Ctrl Pts',(6.46205453683623,-5.,83.3051082611947));
#37743=CARTESIAN_POINT('Ctrl Pts',(6.46205453683623,5.,83.3051082611947));
#37744=CARTESIAN_POINT('Ctrl Pts',(6.42930346455563,-5.,83.3231397091032));
#37745=CARTESIAN_POINT('Ctrl Pts',(6.42930346455563,5.,83.3231397091032));
#37746=CARTESIAN_POINT('Ctrl Pts',(6.40440139687902,-5.,83.3365328421698));
#37747=CARTESIAN_POINT('Ctrl Pts',(6.40440139687902,5.,83.3365328421698));
#37748=CARTESIAN_POINT('Ctrl Pts',(6.38764972936484,-5.,83.3454037233548));
#37749=CARTESIAN_POINT('Ctrl Pts',(6.38764972936484,5.,83.3454037233548));
#37750=CARTESIAN_POINT('Ctrl Pts',(6.37923632332122,-5.,83.3498246953952));
#37751=CARTESIAN_POINT('Ctrl Pts',(6.37923632332122,5.,83.3498246953952));
#37752=CARTESIAN_POINT('Ctrl Pts',(6.48377124583838,-4.8,83.2926771136307));
#37753=CARTESIAN_POINT('Ctrl Pts',(6.48377124583838,-3.13333333333333,83.2926771136307));
#37754=CARTESIAN_POINT('Ctrl Pts',(6.48377124583838,-1.46666666666667,83.2926771136307));
#37755=CARTESIAN_POINT('Ctrl Pts',(6.48377124583838,1.73333333333333,83.2926771136307));
#37756=CARTESIAN_POINT('Ctrl Pts',(6.48377124583837,3.26666666666667,83.2926771136307));
#37757=CARTESIAN_POINT('Ctrl Pts',(6.48377124583837,4.8,83.2926771136307));
#37758=CARTESIAN_POINT('',(7.22998432988738,0.,82.6284406437547));
#37759=CARTESIAN_POINT('Origin',(7.3531668006526,0.,82.2182109750381));
#37760=CARTESIAN_POINT('Ctrl Pts',(12.2407636766788,-5.,83.3498246953952));
#37761=CARTESIAN_POINT('Ctrl Pts',(12.2407636766788,5.,83.3498246953952));
#37762=CARTESIAN_POINT('Ctrl Pts',(12.2323502706297,-5.,83.3454037233561));
#37763=CARTESIAN_POINT('Ctrl Pts',(12.2323502706297,5.,83.3454037233561));
#37764=CARTESIAN_POINT('Ctrl Pts',(12.2155986031059,-5.,83.3365328421734));
#37765=CARTESIAN_POINT('Ctrl Pts',(12.2155986031059,5.,83.3365328421734));
#37766=CARTESIAN_POINT('Ctrl Pts',(12.190696535419,-5.,83.3231397091095));
#37767=CARTESIAN_POINT('Ctrl Pts',(12.190696535419,5.,83.3231397091095));
#37768=CARTESIAN_POINT('Ctrl Pts',(12.1579454631325,-5.,83.3051082612026));
#37769=CARTESIAN_POINT('Ctrl Pts',(12.1579454631325,5.,83.3051082612026));
#37770=CARTESIAN_POINT('Ctrl Pts',(12.1177647907155,-5.,83.2822771755727));
#37771=CARTESIAN_POINT('Ctrl Pts',(12.1177647907155,5.,83.2822771755727));
#37772=CARTESIAN_POINT('Ctrl Pts',(12.0783501058969,-5.,83.2591518588818));
#37773=CARTESIAN_POINT('Ctrl Pts',(12.0783501058969,5.,83.2591518588818));
#37774=CARTESIAN_POINT('Ctrl Pts',(12.0397107079887,-5.,83.2357298380515));
#37775=CARTESIAN_POINT('Ctrl Pts',(12.0397107079887,5.,83.2357298380515));
#37776=CARTESIAN_POINT('Ctrl Pts',(12.0018563255876,-5.,83.2120092344988));
#37777=CARTESIAN_POINT('Ctrl Pts',(12.0018563255876,5.,83.2120092344988));
#37778=CARTESIAN_POINT('Ctrl Pts',(11.9647958564502,-5.,83.1879894016949));
#37779=CARTESIAN_POINT('Ctrl Pts',(11.9647958564502,5.,83.1879894016949));
#37780=CARTESIAN_POINT('Ctrl Pts',(11.92853623968,-5.,83.1636716866526));
#37781=CARTESIAN_POINT('Ctrl Pts',(11.92853623968,5.,83.1636716866526));
#37782=CARTESIAN_POINT('Ctrl Pts',(11.89308503794,-5.,83.1390616951692));
#37783=CARTESIAN_POINT('Ctrl Pts',(11.89308503794,5.,83.1390616951692));
#37784=CARTESIAN_POINT('Ctrl Pts',(11.8584525748976,-5.,83.1141713875545));
#37785=CARTESIAN_POINT('Ctrl Pts',(11.8584525748976,5.,83.1141713875545));
#37786=CARTESIAN_POINT('Ctrl Pts',(11.8246542682811,-5.,83.0890216451873));
#37787=CARTESIAN_POINT('Ctrl Pts',(11.8246542682811,5.,83.0890216451873));
#37788=CARTESIAN_POINT('Ctrl Pts',(11.791712317908,-5.,83.0636440759316));
#37789=CARTESIAN_POINT('Ctrl Pts',(11.791712317908,5.,83.0636440759316));
#37790=CARTESIAN_POINT('Ctrl Pts',(11.7596585546537,-5.,83.0380849627281));
#37791=CARTESIAN_POINT('Ctrl Pts',(11.7596585546537,5.,83.0380849627281));
#37792=CARTESIAN_POINT('Ctrl Pts',(11.7285329169469,-5.,83.012402258898));
#37793=CARTESIAN_POINT('Ctrl Pts',(11.7285329169469,5.,83.012402258898));
#37794=CARTESIAN_POINT('Ctrl Pts',(11.6983766190536,-5.,82.9866540668011));
#37795=CARTESIAN_POINT('Ctrl Pts',(11.6983766190536,5.,82.9866540668011));
#37796=CARTESIAN_POINT('Ctrl Pts',(11.669226271242,-5.,82.960888942289));
#37797=CARTESIAN_POINT('Ctrl Pts',(11.669226271242,5.,82.960888942289));
#37798=CARTESIAN_POINT('Ctrl Pts',(11.6411078833532,-5.,82.9351362301884));
#37799=CARTESIAN_POINT('Ctrl Pts',(11.6411078833532,5.,82.9351362301884));
#37800=CARTESIAN_POINT('Ctrl Pts',(11.6140294535877,-5.,82.9093943694462));
#37801=CARTESIAN_POINT('Ctrl Pts',(11.6140294535877,5.,82.9093943694462));
#37802=CARTESIAN_POINT('Ctrl Pts',(11.5879772511054,-5.,82.883625393001));
#37803=CARTESIAN_POINT('Ctrl Pts',(11.5879772511054,5.,82.883625393001));
#37804=CARTESIAN_POINT('Ctrl Pts',(11.5629375994346,-5.,82.8577907333339));
#37805=CARTESIAN_POINT('Ctrl Pts',(11.5629375994346,5.,82.8577907333339));
#37806=CARTESIAN_POINT('Ctrl Pts',(11.5389164364961,-5.,82.8318837326744));
#37807=CARTESIAN_POINT('Ctrl Pts',(11.5389164364961,5.,82.8318837326744));
#37808=CARTESIAN_POINT('Ctrl Pts',(11.515958184244,-5.,82.8059612344964));
#37809=CARTESIAN_POINT('Ctrl Pts',(11.515958184244,5.,82.8059612344964));
#37810=CARTESIAN_POINT('Ctrl Pts',(11.4941683052261,-5.,82.7801815542291));
#37811=CARTESIAN_POINT('Ctrl Pts',(11.4941683052261,5.,82.7801815542291));
#37812=CARTESIAN_POINT('Ctrl Pts',(11.4737243486416,-5.,82.7548236964487));
#37813=CARTESIAN_POINT('Ctrl Pts',(11.4737243486416,5.,82.7548236964487));
#37814=CARTESIAN_POINT('Ctrl Pts',(11.4548373421755,-5.,82.730224539037));
#37815=CARTESIAN_POINT('Ctrl Pts',(11.4548373421755,5.,82.730224539037));
#37816=CARTESIAN_POINT('Ctrl Pts',(11.4377186539515,-5.,82.7067255844413));
#37817=CARTESIAN_POINT('Ctrl Pts',(11.4377186539515,5.,82.7067255844413));
#37818=CARTESIAN_POINT('Ctrl Pts',(11.4225477629002,-5.,82.6846210078564));
#37819=CARTESIAN_POINT('Ctrl Pts',(11.4225477629002,5.,82.6846210078564));
#37820=CARTESIAN_POINT('Ctrl Pts',(11.4094308327472,-5.,82.6640920750159));
#37821=CARTESIAN_POINT('Ctrl Pts',(11.4094308327472,5.,82.6640920750159));
#37822=CARTESIAN_POINT('Ctrl Pts',(11.4006139236494,-5.,82.6489933638476));
#37823=CARTESIAN_POINT('Ctrl Pts',(11.4006139236494,5.,82.6489933638476));
#37824=CARTESIAN_POINT('Ctrl Pts',(11.3949475071716,-5.,82.6384240779267));
#37825=CARTESIAN_POINT('Ctrl Pts',(11.3949475071716,5.,82.6384240779267));
#37826=CARTESIAN_POINT('Ctrl Pts',(11.391589654405,-5.,82.6317126575424));
#37827=CARTESIAN_POINT('Ctrl Pts',(11.391589654405,5.,82.6317126575424));
#37828=CARTESIAN_POINT('Ctrl Pts',(11.3900156701126,-5.,82.6284406437547));
#37829=CARTESIAN_POINT('Ctrl Pts',(11.3900156701126,5.,82.6284406437547));
#37830=CARTESIAN_POINT('',(11.3900156701126,0.,82.6284406437547));
#37831=CARTESIAN_POINT('Ctrl Pts',(12.1362287541399,4.8,83.2926771136423));
#37832=CARTESIAN_POINT('Ctrl Pts',(12.1362287541399,3.13333333333333,83.2926771136423));
#37833=CARTESIAN_POINT('Ctrl Pts',(12.1362287541399,1.46666666666667,83.2926771136423));
#37834=CARTESIAN_POINT('Ctrl Pts',(12.1362287541399,-1.73333333333333,83.2926771136423));
#37835=CARTESIAN_POINT('Ctrl Pts',(12.1362287541399,-3.26666666666667,83.2926771136423));
#37836=CARTESIAN_POINT('Ctrl Pts',(12.1362287541399,-4.8,83.2926771136423));
#37837=CARTESIAN_POINT('Origin',(9.31000000000013,0.,78.0000000000003));
#37838=CARTESIAN_POINT('',(10.5223925513275,0.,82.4891652120952));
#37839=CARTESIAN_POINT('',(11.2668331993474,0.,82.2182109750381));
#37840=CARTESIAN_POINT('Origin',(11.3900156701126,0.,82.6284406437547));
#37841=CARTESIAN_POINT('Ctrl Pts',(10.691719852285,-5.,82.8825995361566));
#37842=CARTESIAN_POINT('Ctrl Pts',(10.691719852285,5.,82.8825995361566));
#37843=CARTESIAN_POINT('Ctrl Pts',(10.6926173202914,-5.,82.8861177817402));
#37844=CARTESIAN_POINT('Ctrl Pts',(10.6926173202914,5.,82.8861177817402));
#37845=CARTESIAN_POINT('Ctrl Pts',(10.6943590737144,-5.,82.8934174141892));
#37846=CARTESIAN_POINT('Ctrl Pts',(10.6943590737144,5.,82.8934174141892));
#37847=CARTESIAN_POINT('Ctrl Pts',(10.6968121528999,-5.,82.9051562592437));
#37848=CARTESIAN_POINT('Ctrl Pts',(10.6968121528999,5.,82.9051562592437));
#37849=CARTESIAN_POINT('Ctrl Pts',(10.69976327314,-5.,82.9223899429559));
#37850=CARTESIAN_POINT('Ctrl Pts',(10.69976327314,5.,82.9223899429559));
#37851=CARTESIAN_POINT('Ctrl Pts',(10.7029108653431,-5.,82.9465474180549));
#37852=CARTESIAN_POINT('Ctrl Pts',(10.7029108653431,5.,82.9465474180549));
#37853=CARTESIAN_POINT('Ctrl Pts',(10.7054978364887,-5.,82.9732321669037));
#37854=CARTESIAN_POINT('Ctrl Pts',(10.7054978364887,5.,82.9732321669037));
#37855=CARTESIAN_POINT('Ctrl Pts',(10.7074889973481,-5.,83.0022370911707));
#37856=CARTESIAN_POINT('Ctrl Pts',(10.7074889973481,5.,83.0022370911707));
#37857=CARTESIAN_POINT('Ctrl Pts',(10.7088327445902,-5.,83.0332214727508));
#37858=CARTESIAN_POINT('Ctrl Pts',(10.7088327445902,5.,83.0332214727508));
#37859=CARTESIAN_POINT('Ctrl Pts',(10.7094714820479,-5.,83.0657878407809));
#37860=CARTESIAN_POINT('Ctrl Pts',(10.7094714820479,5.,83.0657878407809));
#37861=CARTESIAN_POINT('Ctrl Pts',(10.7093503253746,-5.,83.0995424858489));
#37862=CARTESIAN_POINT('Ctrl Pts',(10.7093503253746,5.,83.0995424858489));
#37863=CARTESIAN_POINT('Ctrl Pts',(10.7084259444592,-5.,83.1341575516224));
#37864=CARTESIAN_POINT('Ctrl Pts',(10.7084259444592,5.,83.1341575516224));
#37865=CARTESIAN_POINT('Ctrl Pts',(10.7066773651025,-5.,83.1694439714256));
#37866=CARTESIAN_POINT('Ctrl Pts',(10.7066773651025,5.,83.1694439714256));
#37867=CARTESIAN_POINT('Ctrl Pts',(10.7041020782155,-5.,83.2053296467487));
#37868=CARTESIAN_POINT('Ctrl Pts',(10.7041020782155,5.,83.2053296467487));
#37869=CARTESIAN_POINT('Ctrl Pts',(10.7007089120433,-5.,83.2418158609177));
#37870=CARTESIAN_POINT('Ctrl Pts',(10.7007089120433,5.,83.2418158609177));
#37871=CARTESIAN_POINT('Ctrl Pts',(10.6965121805262,-5.,83.2789409494337));
#37872=CARTESIAN_POINT('Ctrl Pts',(10.6965121805262,5.,83.2789409494337));
#37873=CARTESIAN_POINT('Ctrl Pts',(10.6915257699886,-5.,83.3167428227683));
#37874=CARTESIAN_POINT('Ctrl Pts',(10.6915257699886,5.,83.3167428227683));
#37875=CARTESIAN_POINT('Ctrl Pts',(10.6857568108328,-5.,83.355217535615));
#37876=CARTESIAN_POINT('Ctrl Pts',(10.6857568108328,5.,83.355217535615));
#37877=CARTESIAN_POINT('Ctrl Pts',(10.6792063652607,-5.,83.3943258897293));
#37878=CARTESIAN_POINT('Ctrl Pts',(10.6792063652607,5.,83.3943258897293));
#37879=CARTESIAN_POINT('Ctrl Pts',(10.6718712672631,-5.,83.4340071565451));
#37880=CARTESIAN_POINT('Ctrl Pts',(10.6718712672631,5.,83.4340071565451));
#37881=CARTESIAN_POINT('Ctrl Pts',(10.6637457413209,-5.,83.4741903350538));
#37882=CARTESIAN_POINT('Ctrl Pts',(10.6637457413209,5.,83.4741903350538));
#37883=CARTESIAN_POINT('Ctrl Pts',(10.6548231303682,-5.,83.5148053585084));
#37884=CARTESIAN_POINT('Ctrl Pts',(10.6548231303682,5.,83.5148053585084));
#37885=CARTESIAN_POINT('Ctrl Pts',(10.6450980681707,-5.,83.555796311625));
#37886=CARTESIAN_POINT('Ctrl Pts',(10.6450980681707,5.,83.555796311625));
#37887=CARTESIAN_POINT('Ctrl Pts',(10.6345672436347,-5.,83.5971247116047));
#37888=CARTESIAN_POINT('Ctrl Pts',(10.6345672436347,5.,83.5971247116047));
#37889=CARTESIAN_POINT('Ctrl Pts',(10.6232290451371,-5.,83.638764652055));
#37890=CARTESIAN_POINT('Ctrl Pts',(10.6232290451371,5.,83.638764652055));
#37891=CARTESIAN_POINT('Ctrl Pts',(10.61108369313,-5.,83.680700334919));
#37892=CARTESIAN_POINT('Ctrl Pts',(10.61108369313,5.,83.680700334919));
#37893=CARTESIAN_POINT('Ctrl Pts',(10.5981333776136,-5.,83.7229226047197));
#37894=CARTESIAN_POINT('Ctrl Pts',(10.5981333776136,5.,83.7229226047197));
#37895=CARTESIAN_POINT('Ctrl Pts',(10.5843825484055,-5.,83.7654259692172));
#37896=CARTESIAN_POINT('Ctrl Pts',(10.5843825484055,5.,83.7654259692172));
#37897=CARTESIAN_POINT('Ctrl Pts',(10.5698384371585,-5.,83.8082052043188));
#37898=CARTESIAN_POINT('Ctrl Pts',(10.5698384371585,5.,83.8082052043188));
#37899=CARTESIAN_POINT('Ctrl Pts',(10.5545097039329,-5.,83.8512554956884));
#37900=CARTESIAN_POINT('Ctrl Pts',(10.5545097039329,5.,83.8512554956884));
#37901=CARTESIAN_POINT('Ctrl Pts',(10.5384050620711,-5.,83.8945727603393));
#37902=CARTESIAN_POINT('Ctrl Pts',(10.5384050620711,5.,83.8945727603393));
#37903=CARTESIAN_POINT('Ctrl Pts',(10.5249066764272,-5.,83.9294376342919));
#37904=CARTESIAN_POINT('Ctrl Pts',(10.5249066764272,5.,83.9294376342919));
#37905=CARTESIAN_POINT('Ctrl Pts',(10.5144395258211,-5.,83.9557041100372));
#37906=CARTESIAN_POINT('Ctrl Pts',(10.5144395258211,5.,83.9557041100372));
#37907=CARTESIAN_POINT('Ctrl Pts',(10.5073090964935,-5.,83.9732673636182));
#37908=CARTESIAN_POINT('Ctrl Pts',(10.5073090964935,5.,83.9732673636182));
#37909=CARTESIAN_POINT('Ctrl Pts',(10.5037057995804,-5.,83.9820620578567));
#37910=CARTESIAN_POINT('Ctrl Pts',(10.5037057995804,5.,83.9820620578567));
#37911=CARTESIAN_POINT('Ctrl Pts',(10.5470504386678,-4.8,83.8710907174214));
#37912=CARTESIAN_POINT('Ctrl Pts',(10.5470504386678,-3.13333333333333,83.8710907174214));
#37913=CARTESIAN_POINT('Ctrl Pts',(10.5470504386678,-1.46666666666667,83.8710907174214));
#37914=CARTESIAN_POINT('Ctrl Pts',(10.5470504386678,1.73333333333333,83.8710907174214));
#37915=CARTESIAN_POINT('Ctrl Pts',(10.5470504386678,3.26666666666667,83.8710907174214));
#37916=CARTESIAN_POINT('Ctrl Pts',(10.5470504386678,4.8,83.8710907174214));
#37917=CARTESIAN_POINT('',(10.691719852285,0.,82.8825995361566));
#37918=CARTESIAN_POINT('Origin',(10.5223925513275,0.,82.4891652120952));
#37919=CARTESIAN_POINT('Ctrl Pts',(14.9938962568098,-5.,80.2143449012797));
#37920=CARTESIAN_POINT('Ctrl Pts',(14.9938962568098,5.,80.2143449012797));
#37921=CARTESIAN_POINT('Ctrl Pts',(14.9846094678237,-5.,80.2163662733741));
#37922=CARTESIAN_POINT('Ctrl Pts',(14.9846094678237,5.,80.2163662733741));
#37923=CARTESIAN_POINT('Ctrl Pts',(14.9660748535191,-5.,80.2203385484548));
#37924=CARTESIAN_POINT('Ctrl Pts',(14.9660748535191,5.,80.2203385484548));
#37925=CARTESIAN_POINT('Ctrl Pts',(14.9383898229852,-5.,80.2260855538497));
#37926=CARTESIAN_POINT('Ctrl Pts',(14.9383898229852,5.,80.2260855538497));
#37927=CARTESIAN_POINT('Ctrl Pts',(14.9017106547708,-5.,80.233324646843));
#37928=CARTESIAN_POINT('Ctrl Pts',(14.9017106547708,5.,80.233324646843));
#37929=CARTESIAN_POINT('Ctrl Pts',(14.8562549349791,-5.,80.2416626589468));
#37930=CARTESIAN_POINT('Ctrl Pts',(14.8562549349791,5.,80.2416626589468));
#37931=CARTESIAN_POINT('Ctrl Pts',(14.8111968676331,-5.,80.2492829096502));
#37932=CARTESIAN_POINT('Ctrl Pts',(14.8111968676331,5.,80.2492829096502));
#37933=CARTESIAN_POINT('Ctrl Pts',(14.7665419867659,-5.,80.256177526979));
#37934=CARTESIAN_POINT('Ctrl Pts',(14.7665419867659,5.,80.256177526979));
#37935=CARTESIAN_POINT('Ctrl Pts',(14.7222965373946,-5.,80.26233881843));
#37936=CARTESIAN_POINT('Ctrl Pts',(14.7222965373946,5.,80.26233881843));
#37937=CARTESIAN_POINT('Ctrl Pts',(14.6784669200222,-5.,80.2677605693635));
#37938=CARTESIAN_POINT('Ctrl Pts',(14.6784669200222,5.,80.2677605693635));
#37939=CARTESIAN_POINT('Ctrl Pts',(14.6350593161548,-5.,80.2724393512806));
#37940=CARTESIAN_POINT('Ctrl Pts',(14.6350593161548,5.,80.2724393512806));
#37941=CARTESIAN_POINT('Ctrl Pts',(14.5920831224637,-5.,80.2763745972856));
#37942=CARTESIAN_POINT('Ctrl Pts',(14.5920831224637,5.,80.2763745972856));
#37943=CARTESIAN_POINT('Ctrl Pts',(14.5495539352719,-5.,80.2795688335829));
#37944=CARTESIAN_POINT('Ctrl Pts',(14.5495539352719,5.,80.2795688335829));
#37945=CARTESIAN_POINT('Ctrl Pts',(14.5074969875316,-5.,80.2820281459137));
#37946=CARTESIAN_POINT('Ctrl Pts',(14.5074969875316,5.,80.2820281459137));
#37947=CARTESIAN_POINT('Ctrl Pts',(14.4659496024287,-5.,80.28376247754));
#37948=CARTESIAN_POINT('Ctrl Pts',(14.4659496024287,5.,80.28376247754));
#37949=CARTESIAN_POINT('Ctrl Pts',(14.4249659139275,-5.,80.2847868227605));
#37950=CARTESIAN_POINT('Ctrl Pts',(14.4249659139275,5.,80.2847868227605));
#37951=CARTESIAN_POINT('Ctrl Pts',(14.3846137683172,-5.,80.2851199044676));
#37952=CARTESIAN_POINT('Ctrl Pts',(14.3846137683172,5.,80.2851199044676));
#37953=CARTESIAN_POINT('Ctrl Pts',(14.3449620850361,-5.,80.2847797396321));
#37954=CARTESIAN_POINT('Ctrl Pts',(14.3449620850361,5.,80.2847797396321));
#37955=CARTESIAN_POINT('Ctrl Pts',(14.306070120279,-5.,80.283779991567));
#37956=CARTESIAN_POINT('Ctrl Pts',(14.306070120279,5.,80.283779991567));
#37957=CARTESIAN_POINT('Ctrl Pts',(14.2679766612333,-5.,80.2821264209094));
#37958=CARTESIAN_POINT('Ctrl Pts',(14.2679766612333,5.,80.2821264209094));
#37959=CARTESIAN_POINT('Ctrl Pts',(14.2306868314505,-5.,80.2798126906777));
#37960=CARTESIAN_POINT('Ctrl Pts',(14.2306868314505,5.,80.2798126906777));
#37961=CARTESIAN_POINT('Ctrl Pts',(14.1941657077385,-5.,80.2768185424287));
#37962=CARTESIAN_POINT('Ctrl Pts',(14.1941657077385,5.,80.2768185424287));
#37963=CARTESIAN_POINT('Ctrl Pts',(14.1583780225859,-5.,80.2731232227952));
#37964=CARTESIAN_POINT('Ctrl Pts',(14.1583780225859,5.,80.2731232227952));
#37965=CARTESIAN_POINT('Ctrl Pts',(14.1233240451694,-5.,80.2687178148077));
#37966=CARTESIAN_POINT('Ctrl Pts',(14.1233240451694,5.,80.2687178148077));
#37967=CARTESIAN_POINT('Ctrl Pts',(14.0890743429602,-5.,80.2636173092121));
#37968=CARTESIAN_POINT('Ctrl Pts',(14.0890743429602,5.,80.2636173092121));
#37969=CARTESIAN_POINT('Ctrl Pts',(14.0558114681554,-5.,80.2578751926453));
#37970=CARTESIAN_POINT('Ctrl Pts',(14.0558114681554,5.,80.2578751926453));
#37971=CARTESIAN_POINT('Ctrl Pts',(14.023850772022,-5.,80.2515910685876));
#37972=CARTESIAN_POINT('Ctrl Pts',(14.023850772022,5.,80.2515910685876));
#37973=CARTESIAN_POINT('Ctrl Pts',(13.9935704520791,-5.,80.244887354488));
#37974=CARTESIAN_POINT('Ctrl Pts',(13.9935704520791,5.,80.244887354488));
#37975=CARTESIAN_POINT('Ctrl Pts',(13.9653519392474,-5.,80.2378897915872));
#37976=CARTESIAN_POINT('Ctrl Pts',(13.9653519392474,5.,80.2378897915872));
#37977=CARTESIAN_POINT('Ctrl Pts',(13.9395218145325,-5.,80.2307083643255));
#37978=CARTESIAN_POINT('Ctrl Pts',(13.9395218145325,5.,80.2307083643255));
#37979=CARTESIAN_POINT('Ctrl Pts',(13.9162779194248,-5.,80.2234136895821));
#37980=CARTESIAN_POINT('Ctrl Pts',(13.9162779194248,5.,80.2234136895821));
#37981=CARTESIAN_POINT('Ctrl Pts',(13.8998185107453,-5.,80.2175148057176));
#37982=CARTESIAN_POINT('Ctrl Pts',(13.8998185107453,5.,80.2175148057176));
#37983=CARTESIAN_POINT('Ctrl Pts',(13.8886839778468,-5.,80.2130605652718));
#37984=CARTESIAN_POINT('Ctrl Pts',(13.8886839778468,5.,80.2130605652718));
#37985=CARTESIAN_POINT('Ctrl Pts',(13.8817976955151,-5.,80.2100777051323));
#37986=CARTESIAN_POINT('Ctrl Pts',(13.8817976955151,5.,80.2100777051323));
#37987=CARTESIAN_POINT('Ctrl Pts',(13.8784887436653,-5.,80.2085829347521));
#37988=CARTESIAN_POINT('Ctrl Pts',(13.8784887436653,5.,80.2085829347521));
#37989=CARTESIAN_POINT('',(13.8784887436653,0.,80.2085829347521));
#37990=CARTESIAN_POINT('Ctrl Pts',(14.877084102819,4.8,80.237761066812));
#37991=CARTESIAN_POINT('Ctrl Pts',(14.877084102819,3.13333333333333,80.237761066812));
#37992=CARTESIAN_POINT('Ctrl Pts',(14.877084102819,1.46666666666667,80.237761066812));
#37993=CARTESIAN_POINT('Ctrl Pts',(14.877084102819,-1.73333333333333,80.237761066812));
#37994=CARTESIAN_POINT('Ctrl Pts',(14.877084102819,-3.26666666666667,80.237761066812));
#37995=CARTESIAN_POINT('Ctrl Pts',(14.877084102819,-4.8,80.237761066812));
#37996=CARTESIAN_POINT('Origin',(9.31000000000061,0.,78.0000000000004));
#37997=CARTESIAN_POINT('',(13.1243263529939,0.,80.659589154899));
#37998=CARTESIAN_POINT('',(13.5204349482691,0.,79.9735089425676));
#37999=CARTESIAN_POINT('Origin',(13.8784887436653,0.,80.2085829347521));
#38000=CARTESIAN_POINT('Ctrl Pts',(13.5069332996928,-5.,80.8521358415414));
#38001=CARTESIAN_POINT('Ctrl Pts',(13.5069332996928,5.,80.8521358415414));
#38002=CARTESIAN_POINT('Ctrl Pts',(13.5098822847458,-5.,80.8542540927002));
#38003=CARTESIAN_POINT('Ctrl Pts',(13.5098822847458,5.,80.8542540927002));
#38004=CARTESIAN_POINT('Ctrl Pts',(13.5159086585781,-5.,80.8587263580464));
#38005=CARTESIAN_POINT('Ctrl Pts',(13.5159086585781,5.,80.8587263580464));
#38006=CARTESIAN_POINT('Ctrl Pts',(13.5253334104161,-5.,80.8661420261559));
#38007=CARTESIAN_POINT('Ctrl Pts',(13.5253334104161,5.,80.8661420261559));
#38008=CARTESIAN_POINT('Ctrl Pts',(13.5386716980353,-5.,80.8774468502741));
#38009=CARTESIAN_POINT('Ctrl Pts',(13.5386716980353,5.,80.8774468502741));
#38010=CARTESIAN_POINT('Ctrl Pts',(13.5566110192161,-5.,80.8939293165766));
#38011=CARTESIAN_POINT('Ctrl Pts',(13.5566110192161,5.,80.8939293165766));
#38012=CARTESIAN_POINT('Ctrl Pts',(13.5757453800031,-5.,80.9127081471622));
#38013=CARTESIAN_POINT('Ctrl Pts',(13.5757453800031,5.,80.9127081471622));
#38014=CARTESIAN_POINT('Ctrl Pts',(13.5959147036475,-5.,80.9336473146984));
#38015=CARTESIAN_POINT('Ctrl Pts',(13.5959147036475,5.,80.9336473146984));
#38016=CARTESIAN_POINT('Ctrl Pts',(13.6168604503288,-5.,80.9565189839544));
#38017=CARTESIAN_POINT('Ctrl Pts',(13.6168604503288,5.,80.9565189839544));
#38018=CARTESIAN_POINT('Ctrl Pts',(13.6382830094757,-5.,80.9810556966881));
#38019=CARTESIAN_POINT('Ctrl Pts',(13.6382830094757,5.,80.9810556966881));
#38020=CARTESIAN_POINT('Ctrl Pts',(13.6598872657035,-5.,81.0069911329731));
#38021=CARTESIAN_POINT('Ctrl Pts',(13.6598872657035,5.,81.0069911329731));
#38022=CARTESIAN_POINT('Ctrl Pts',(13.6814292842305,-5.,81.0341019923499));
#38023=CARTESIAN_POINT('Ctrl Pts',(13.6814292842305,5.,81.0341019923499));
#38024=CARTESIAN_POINT('Ctrl Pts',(13.7027714681705,-5.,81.0622569232995));
#38025=CARTESIAN_POINT('Ctrl Pts',(13.7027714681705,5.,81.0622569232995));
#38026=CARTESIAN_POINT('Ctrl Pts',(13.7238655514223,-5.,81.091402307971));
#38027=CARTESIAN_POINT('Ctrl Pts',(13.7238655514223,5.,81.091402307971));
#38028=CARTESIAN_POINT('Ctrl Pts',(13.744719121722,-5.,81.1215334547618));
#38029=CARTESIAN_POINT('Ctrl Pts',(13.744719121722,5.,81.1215334547618));
#38030=CARTESIAN_POINT('Ctrl Pts',(13.7653677857709,-5.,81.1526705295447));
#38031=CARTESIAN_POINT('Ctrl Pts',(13.7653677857709,5.,81.1526705295447));
#38032=CARTESIAN_POINT('Ctrl Pts',(13.7858465494927,-5.,81.1848336474667));
#38033=CARTESIAN_POINT('Ctrl Pts',(13.7858465494927,5.,81.1848336474667));
#38034=CARTESIAN_POINT('Ctrl Pts',(13.8061583390971,-5.,81.2180152029123));
#38035=CARTESIAN_POINT('Ctrl Pts',(13.8061583390971,5.,81.2180152029123));
#38036=CARTESIAN_POINT('Ctrl Pts',(13.8262787721302,-5.,81.2521844855136));
#38037=CARTESIAN_POINT('Ctrl Pts',(13.8262787721302,5.,81.2521844855136));
#38038=CARTESIAN_POINT('Ctrl Pts',(13.8461663877157,-5.,81.2872970095613));
#38039=CARTESIAN_POINT('Ctrl Pts',(13.8461663877157,5.,81.2872970095613));
#38040=CARTESIAN_POINT('Ctrl Pts',(13.8657711229787,-5.,81.3233020975591));
#38041=CARTESIAN_POINT('Ctrl Pts',(13.8657711229787,5.,81.3233020975591));
#38042=CARTESIAN_POINT('Ctrl Pts',(13.8850428402732,-5.,81.3601503543448));
#38043=CARTESIAN_POINT('Ctrl Pts',(13.8850428402732,5.,81.3601503543448));
#38044=CARTESIAN_POINT('Ctrl Pts',(13.9039414871764,-5.,81.3978023956762));
#38045=CARTESIAN_POINT('Ctrl Pts',(13.9039414871764,5.,81.3978023956762));
#38046=CARTESIAN_POINT('Ctrl Pts',(13.9224397909821,-5.,81.4362308703506));
#38047=CARTESIAN_POINT('Ctrl Pts',(13.9224397909821,5.,81.4362308703506));
#38048=CARTESIAN_POINT('Ctrl Pts',(13.9405198648132,-5.,81.4754169688537));
#38049=CARTESIAN_POINT('Ctrl Pts',(13.9405198648132,5.,81.4754169688537));
#38050=CARTESIAN_POINT('Ctrl Pts',(13.9581717227552,-5.,81.515348447469));
#38051=CARTESIAN_POINT('Ctrl Pts',(13.9581717227552,5.,81.515348447469));
#38052=CARTESIAN_POINT('Ctrl Pts',(13.9753911574206,-5.,81.55601688499));
#38053=CARTESIAN_POINT('Ctrl Pts',(13.9753911574206,5.,81.55601688499));
#38054=CARTESIAN_POINT('Ctrl Pts',(13.9921780472216,-5.,81.5974152138281));
#38055=CARTESIAN_POINT('Ctrl Pts',(13.9921780472216,5.,81.5974152138281));
#38056=CARTESIAN_POINT('Ctrl Pts',(14.0085345739351,-5.,81.6395347836759));
#38057=CARTESIAN_POINT('Ctrl Pts',(14.0085345739351,5.,81.6395347836759));
#38058=CARTESIAN_POINT('Ctrl Pts',(14.0244642769442,-5.,81.6823663399542));
#38059=CARTESIAN_POINT('Ctrl Pts',(14.0244642769442,5.,81.6823663399542));
#38060=CARTESIAN_POINT('Ctrl Pts',(14.0399712065494,-5.,81.7259011540809));
#38061=CARTESIAN_POINT('Ctrl Pts',(14.0399712065494,5.,81.7259011540809));
#38062=CARTESIAN_POINT('Ctrl Pts',(14.052041552205,-5.,81.7612857920673));
#38063=CARTESIAN_POINT('Ctrl Pts',(14.052041552205,5.,81.7612857920673));
#38064=CARTESIAN_POINT('Ctrl Pts',(14.0609070147714,-5.,81.7881352345583));
#38065=CARTESIAN_POINT('Ctrl Pts',(14.0609070147714,5.,81.7881352345583));
#38066=CARTESIAN_POINT('Ctrl Pts',(14.0667342307623,-5.,81.8061728189791));
#38067=CARTESIAN_POINT('Ctrl Pts',(14.0667342307623,5.,81.8061728189791));
#38068=CARTESIAN_POINT('Ctrl Pts',(14.0696270656537,-5.,81.8152261002327));
#38069=CARTESIAN_POINT('Ctrl Pts',(14.0696270656537,5.,81.8152261002327));
#38070=CARTESIAN_POINT('Ctrl Pts',(14.0314999829639,-4.8,81.7023557245181));
#38071=CARTESIAN_POINT('Ctrl Pts',(14.0314999829639,-3.13333333333333,81.7023557245181));
#38072=CARTESIAN_POINT('Ctrl Pts',(14.0314999829639,-1.46666666666667,81.7023557245181));
#38073=CARTESIAN_POINT('Ctrl Pts',(14.0314999829639,1.73333333333333,81.7023557245181));
#38074=CARTESIAN_POINT('Ctrl Pts',(14.0314999829639,3.26666666666667,81.7023557245181));
#38075=CARTESIAN_POINT('Ctrl Pts',(14.0314999829639,4.8,81.7023557245181));
#38076=CARTESIAN_POINT('',(13.5069332996928,0.,80.8521358415414));
#38077=CARTESIAN_POINT('Origin',(13.1243263529939,0.,80.659589154899));
#38078=CARTESIAN_POINT('Ctrl Pts',(3.21153406965502,-5.,77.8632034487949));
#38079=CARTESIAN_POINT('Ctrl Pts',(3.21153406965502,5.,77.8632034487949));
#38080=CARTESIAN_POINT('Ctrl Pts',(3.21956944675077,-5.,77.8581277114052));
#38081=CARTESIAN_POINT('Ctrl Pts',(3.21956944675077,5.,77.8581277114052));
#38082=CARTESIAN_POINT('Ctrl Pts',(3.23562768892862,-5.,77.8480557822981));
#38083=CARTESIAN_POINT('Ctrl Pts',(3.23562768892862,5.,77.8480557822981));
#38084=CARTESIAN_POINT('Ctrl Pts',(3.2596775161963,-5.,77.833186525534));
#38085=CARTESIAN_POINT('Ctrl Pts',(3.2596775161963,5.,77.833186525534));
#38086=CARTESIAN_POINT('Ctrl Pts',(3.29166874426794,-5.,77.8138389888443));
#38087=CARTESIAN_POINT('Ctrl Pts',(3.29166874426794,5.,77.8138389888443));
#38088=CARTESIAN_POINT('Ctrl Pts',(3.33153138063963,-5.,77.7904570486231));
#38089=CARTESIAN_POINT('Ctrl Pts',(3.33153138063963,5.,77.7904570486231));
#38090=CARTESIAN_POINT('Ctrl Pts',(3.37126583481311,-5.,77.7678855886958));
#38091=CARTESIAN_POINT('Ctrl Pts',(3.37126583481311,5.,77.7678855886958));
#38092=CARTESIAN_POINT('Ctrl Pts',(3.41086959886361,-5.,77.7461338990146));
#38093=CARTESIAN_POINT('Ctrl Pts',(3.41086959886361,5.,77.7461338990146));
#38094=CARTESIAN_POINT('Ctrl Pts',(3.45033943537775,-5.,77.7252113440577));
#38095=CARTESIAN_POINT('Ctrl Pts',(3.45033943537775,5.,77.7252113440577));
#38096=CARTESIAN_POINT('Ctrl Pts',(3.48967145537702,-5.,77.7051259527562));
#38097=CARTESIAN_POINT('Ctrl Pts',(3.48967145537702,5.,77.7051259527562));
#38098=CARTESIAN_POINT('Ctrl Pts',(3.52886102276024,-5.,77.6858830610395));
#38099=CARTESIAN_POINT('Ctrl Pts',(3.52886102276024,5.,77.6858830610395));
#38100=CARTESIAN_POINT('Ctrl Pts',(3.56789950143585,-5.,77.6674864154709));
#38101=CARTESIAN_POINT('Ctrl Pts',(3.56789950143585,5.,77.6674864154709));
#38102=CARTESIAN_POINT('Ctrl Pts',(3.60677137164422,-5.,77.6499389764635));
#38103=CARTESIAN_POINT('Ctrl Pts',(3.60677137164422,5.,77.6499389764635));
#38104=CARTESIAN_POINT('Ctrl Pts',(3.64545084072427,-5.,77.6332436554839));
#38105=CARTESIAN_POINT('Ctrl Pts',(3.64545084072427,5.,77.6332436554839));
#38106=CARTESIAN_POINT('Ctrl Pts',(3.68389943556033,-5.,77.6174038742161));
#38107=CARTESIAN_POINT('Ctrl Pts',(3.68389943556033,5.,77.6174038742161));
#38108=CARTESIAN_POINT('Ctrl Pts',(3.72206115851557,-5.,77.6024240575425));
#38109=CARTESIAN_POINT('Ctrl Pts',(3.72206115851557,5.,77.6024240575425));
#38110=CARTESIAN_POINT('Ctrl Pts',(3.75986585132557,-5.,77.5883098164954));
#38111=CARTESIAN_POINT('Ctrl Pts',(3.75986585132557,5.,77.5883098164954));
#38112=CARTESIAN_POINT('Ctrl Pts',(3.79724258873478,-5.,77.5750677924921));
#38113=CARTESIAN_POINT('Ctrl Pts',(3.79724258873478,5.,77.5750677924921));
#38114=CARTESIAN_POINT('Ctrl Pts',(3.834131015004,-5.,77.5627054130235));
#38115=CARTESIAN_POINT('Ctrl Pts',(3.834131015004,5.,77.5627054130235));
#38116=CARTESIAN_POINT('Ctrl Pts',(3.87049271184419,-5.,77.5512305308539));
#38117=CARTESIAN_POINT('Ctrl Pts',(3.87049271184419,5.,77.5512305308539));
#38118=CARTESIAN_POINT('Ctrl Pts',(3.90632503206606,-5.,77.5406508531519));
#38119=CARTESIAN_POINT('Ctrl Pts',(3.90632503206606,5.,77.5406508531519));
#38120=CARTESIAN_POINT('Ctrl Pts',(3.94166772153233,-5.,77.5309734721948));
#38121=CARTESIAN_POINT('Ctrl Pts',(3.94166772153233,5.,77.5309734721948));
#38122=CARTESIAN_POINT('Ctrl Pts',(3.97656101893436,-5.,77.5222058275747));
#38123=CARTESIAN_POINT('Ctrl Pts',(3.97656101893436,5.,77.5222058275747));
#38124=CARTESIAN_POINT('Ctrl Pts',(4.01100772111374,-5.,77.5143563905724));
#38125=CARTESIAN_POINT('Ctrl Pts',(4.01100772111374,5.,77.5143563905724));
#38126=CARTESIAN_POINT('Ctrl Pts',(4.04493638920223,-5.,77.5074352099941));
#38127=CARTESIAN_POINT('Ctrl Pts',(4.04493638920223,5.,77.5074352099941));
#38128=CARTESIAN_POINT('Ctrl Pts',(4.07815718673909,-5.,77.5014544613682));
#38129=CARTESIAN_POINT('Ctrl Pts',(4.07815718673909,5.,77.5014544613682));
#38130=CARTESIAN_POINT('Ctrl Pts',(4.11033971406609,-5.,77.4964284045146));
#38131=CARTESIAN_POINT('Ctrl Pts',(4.11033971406609,5.,77.4964284045146));
#38132=CARTESIAN_POINT('Ctrl Pts',(4.1410867125286,-5.,77.4923713558191));
#38133=CARTESIAN_POINT('Ctrl Pts',(4.1410867125286,5.,77.4923713558191));
#38134=CARTESIAN_POINT('Ctrl Pts',(4.16999674826609,-5.,77.4892956142181));
#38135=CARTESIAN_POINT('Ctrl Pts',(4.16999674826609,5.,77.4892956142181));
#38136=CARTESIAN_POINT('Ctrl Pts',(4.19672531862458,-5.,77.487209525431));
#38137=CARTESIAN_POINT('Ctrl Pts',(4.19672531862458,5.,77.487209525431));
#38138=CARTESIAN_POINT('Ctrl Pts',(4.22106236102637,-5.,77.4861143970901));
#38139=CARTESIAN_POINT('Ctrl Pts',(4.22106236102637,5.,77.4861143970901));
#38140=CARTESIAN_POINT('Ctrl Pts',(4.23854668300876,-5.,77.4860280854099));
#38141=CARTESIAN_POINT('Ctrl Pts',(4.23854668300876,5.,77.4860280854099));
#38142=CARTESIAN_POINT('Ctrl Pts',(4.25053316137149,-5.,77.4864054677697));
#38143=CARTESIAN_POINT('Ctrl Pts',(4.25053316137149,5.,77.4864054677697));
#38144=CARTESIAN_POINT('Ctrl Pts',(4.25802434832342,-5.,77.4868531921852));
#38145=CARTESIAN_POINT('Ctrl Pts',(4.25802434832342,5.,77.4868531921852));
#38146=CARTESIAN_POINT('Ctrl Pts',(4.2616449875437,-5.,77.4871260887099));
#38147=CARTESIAN_POINT('Ctrl Pts',(4.2616449875437,5.,77.4871260887099));
#38148=CARTESIAN_POINT('',(4.2616449875437,0.,77.4871260887099));
#38149=CARTESIAN_POINT('Ctrl Pts',(3.3132927884967,4.8,77.8012473408872));
#38150=CARTESIAN_POINT('Ctrl Pts',(3.3132927884967,3.13333333333333,77.8012473408872));
#38151=CARTESIAN_POINT('Ctrl Pts',(3.3132927884967,1.46666666666667,77.8012473408872));
#38152=CARTESIAN_POINT('Ctrl Pts',(3.3132927884967,-1.73333333333333,77.8012473408872));
#38153=CARTESIAN_POINT('Ctrl Pts',(3.3132927884967,-3.26666666666667,77.8012473408872));
#38154=CARTESIAN_POINT('Ctrl Pts',(3.3132927884967,-4.8,77.8012473408872));
#38155=CARTESIAN_POINT('Origin',(9.3100000000004,0.,78.0000000000001));
#38156=CARTESIAN_POINT('',(4.81607260887647,0.,76.805380142761));
#38157=CARTESIAN_POINT('',(4.67850553742098,0.,77.5855617740846));
#38158=CARTESIAN_POINT('Origin',(4.2616449875437,0.,77.4871260887099));
#38159=CARTESIAN_POINT('Ctrl Pts',(4.39068483903982,-5.,76.7553047249138));
#38160=CARTESIAN_POINT('Ctrl Pts',(4.39068483903982,5.,76.7553047249138));
#38161=CARTESIAN_POINT('Ctrl Pts',(4.38718921497661,-5.,76.754322832203));
#38162=CARTESIAN_POINT('Ctrl Pts',(4.38718921497661,5.,76.754322832203));
#38163=CARTESIAN_POINT('Ctrl Pts',(4.37999667111321,-5.,76.752181418671));
#38164=CARTESIAN_POINT('Ctrl Pts',(4.37999667111321,5.,76.752181418671));
#38165=CARTESIAN_POINT('Ctrl Pts',(4.36860399348183,-5.,76.7484364250207));
#38166=CARTESIAN_POINT('Ctrl Pts',(4.36860399348183,5.,76.7484364250207));
#38167=CARTESIAN_POINT('Ctrl Pts',(4.3522036254681,-5.,76.7423753282649));
#38168=CARTESIAN_POINT('Ctrl Pts',(4.3522036254681,5.,76.7423753282649));
#38169=CARTESIAN_POINT('Ctrl Pts',(4.32970884225672,-5.,76.7330224855494));
#38170=CARTESIAN_POINT('Ctrl Pts',(4.32970884225672,5.,76.7330224855494));
#38171=CARTESIAN_POINT('Ctrl Pts',(4.30530568630539,-5.,76.7219204938829));
#38172=CARTESIAN_POINT('Ctrl Pts',(4.30530568630539,5.,76.7219204938829));
#38173=CARTESIAN_POINT('Ctrl Pts',(4.27919110463543,-5.,76.7091424276514));
#38174=CARTESIAN_POINT('Ctrl Pts',(4.27919110463543,5.,76.7091424276514));
#38175=CARTESIAN_POINT('Ctrl Pts',(4.25168596944519,-5.,76.6948139561091));
#38176=CARTESIAN_POINT('Ctrl Pts',(4.25168596944519,5.,76.6948139561091));
#38177=CARTESIAN_POINT('Ctrl Pts',(4.22316329868605,-5.,76.6790839349482));
#38178=CARTESIAN_POINT('Ctrl Pts',(4.22316329868605,5.,76.6790839349482));
#38179=CARTESIAN_POINT('Ctrl Pts',(4.19399149688978,-5.,76.6621016876446));
#38180=CARTESIAN_POINT('Ctrl Pts',(4.19399149688978,5.,76.6621016876446));
#38181=CARTESIAN_POINT('Ctrl Pts',(4.16447616102936,-5.,76.6439936173946));
#38182=CARTESIAN_POINT('Ctrl Pts',(4.16447616102936,5.,76.6439936173946));
#38183=CARTESIAN_POINT('Ctrl Pts',(4.13479151474963,-5.,76.6248360933485));
#38184=CARTESIAN_POINT('Ctrl Pts',(4.13479151474963,5.,76.6248360933485));
#38185=CARTESIAN_POINT('Ctrl Pts',(4.1050012517344,-5.,76.6046629918244));
#38186=CARTESIAN_POINT('Ctrl Pts',(4.1050012517344,5.,76.6046629918244));
#38187=CARTESIAN_POINT('Ctrl Pts',(4.075099846465,-5.,76.5834813166402));
#38188=CARTESIAN_POINT('Ctrl Pts',(4.075099846465,5.,76.5834813166402));
#38189=CARTESIAN_POINT('Ctrl Pts',(4.04504694245075,-5.,76.561284296277));
#38190=CARTESIAN_POINT('Ctrl Pts',(4.04504694245075,5.,76.561284296277));
#38191=CARTESIAN_POINT('Ctrl Pts',(4.01480276509665,-5.,76.5380650014064));
#38192=CARTESIAN_POINT('Ctrl Pts',(4.01480276509665,5.,76.5380650014064));
#38193=CARTESIAN_POINT('Ctrl Pts',(3.98436716593925,-5.,76.5138315797934));
#38194=CARTESIAN_POINT('Ctrl Pts',(3.98436716593925,5.,76.5138315797934));
#38195=CARTESIAN_POINT('Ctrl Pts',(3.95377356055623,-5.,76.4886045504577));
#38196=CARTESIAN_POINT('Ctrl Pts',(3.95377356055623,5.,76.4886045504577));
#38197=CARTESIAN_POINT('Ctrl Pts',(3.92307612443753,-5.,76.4624115358435));
#38198=CARTESIAN_POINT('Ctrl Pts',(3.92307612443753,5.,76.4624115358435));
#38199=CARTESIAN_POINT('Ctrl Pts',(3.89233923402299,-5.,76.4352830347124));
#38200=CARTESIAN_POINT('Ctrl Pts',(3.89233923402299,5.,76.4352830347124));
#38201=CARTESIAN_POINT('Ctrl Pts',(3.86162689742974,-5.,76.4072483152511));
#38202=CARTESIAN_POINT('Ctrl Pts',(3.86162689742974,5.,76.4072483152511));
#38203=CARTESIAN_POINT('Ctrl Pts',(3.83099022182655,-5.,76.3783306878011));
#38204=CARTESIAN_POINT('Ctrl Pts',(3.83099022182655,5.,76.3783306878011));
#38205=CARTESIAN_POINT('Ctrl Pts',(3.80046418983392,-5.,76.3485465262618));
#38206=CARTESIAN_POINT('Ctrl Pts',(3.80046418983392,5.,76.3485465262618));
#38207=CARTESIAN_POINT('Ctrl Pts',(3.77007204284776,-5.,76.3179073881124));
#38208=CARTESIAN_POINT('Ctrl Pts',(3.77007204284776,5.,76.3179073881124));
#38209=CARTESIAN_POINT('Ctrl Pts',(3.73982735215308,-5.,76.2864213632901));
#38210=CARTESIAN_POINT('Ctrl Pts',(3.73982735215308,5.,76.2864213632901));
#38211=CARTESIAN_POINT('Ctrl Pts',(3.70973695162212,-5.,76.2540949261254));
#38212=CARTESIAN_POINT('Ctrl Pts',(3.70973695162212,5.,76.2540949261254));
#38213=CARTESIAN_POINT('Ctrl Pts',(3.67980337276852,-5.,76.2209346763969));
#38214=CARTESIAN_POINT('Ctrl Pts',(3.67980337276852,5.,76.2209346763969));
#38215=CARTESIAN_POINT('Ctrl Pts',(3.65002752397655,-5.,76.1869494889609));
#38216=CARTESIAN_POINT('Ctrl Pts',(3.65002752397655,5.,76.1869494889609));
#38217=CARTESIAN_POINT('Ctrl Pts',(3.62040924457333,-5.,76.1521492708398));
#38218=CARTESIAN_POINT('Ctrl Pts',(3.62040924457333,5.,76.1521492708398));
#38219=CARTESIAN_POINT('Ctrl Pts',(3.59094771387985,-5.,76.1165436095273));
#38220=CARTESIAN_POINT('Ctrl Pts',(3.59094771387985,5.,76.1165436095273));
#38221=CARTESIAN_POINT('Ctrl Pts',(3.56750304019246,-5.,76.0874212277101));
#38222=CARTESIAN_POINT('Ctrl Pts',(3.56750304019246,5.,76.0874212277101));
#38223=CARTESIAN_POINT('Ctrl Pts',(3.54998918028979,-5.,76.0652231715713));
#38224=CARTESIAN_POINT('Ctrl Pts',(3.54998918028979,5.,76.0652231715713));
#38225=CARTESIAN_POINT('Ctrl Pts',(3.53834417123289,-5.,76.0502664119026));
#38226=CARTESIAN_POINT('Ctrl Pts',(3.53834417123289,5.,76.0502664119026));
#38227=CARTESIAN_POINT('Ctrl Pts',(3.53252939109094,-5.,76.0427485181531));
#38228=CARTESIAN_POINT('Ctrl Pts',(3.53252939109094,5.,76.0427485181531));
#38229=CARTESIAN_POINT('Ctrl Pts',(3.60696107145242,-4.8,76.1357717469497));
#38230=CARTESIAN_POINT('Ctrl Pts',(3.60696107145242,-3.13333333333333,76.1357717469497));
#38231=CARTESIAN_POINT('Ctrl Pts',(3.60696107145242,-1.46666666666667,76.1357717469497));
#38232=CARTESIAN_POINT('Ctrl Pts',(3.60696107145242,1.73333333333333,76.1357717469497));
#38233=CARTESIAN_POINT('Ctrl Pts',(3.60696107145241,3.26666666666667,76.1357717469497));
#38234=CARTESIAN_POINT('Ctrl Pts',(3.60696107145241,4.8,76.1357717469497));
#38235=CARTESIAN_POINT('',(4.39068483903982,0.,76.7553047249138));
#38236=CARTESIAN_POINT('Origin',(4.81607260887647,0.,76.805380142761));
#38237=CARTESIAN_POINT('Ctrl Pts',(14.0696270656537,-5.,74.1847738997673));
#38238=CARTESIAN_POINT('Ctrl Pts',(14.0696270656537,5.,74.1847738997673));
#38239=CARTESIAN_POINT('Ctrl Pts',(14.0667342307623,-5.,74.1938271809842));
#38240=CARTESIAN_POINT('Ctrl Pts',(14.0667342307623,5.,74.1938271809842));
#38241=CARTESIAN_POINT('Ctrl Pts',(14.0609070147712,-5.,74.211864765341));
#38242=CARTESIAN_POINT('Ctrl Pts',(14.0609070147712,5.,74.211864765341));
#38243=CARTESIAN_POINT('Ctrl Pts',(14.0520415522048,-5.,74.238714207763));
#38244=CARTESIAN_POINT('Ctrl Pts',(14.0520415522048,5.,74.238714207763));
#38245=CARTESIAN_POINT('Ctrl Pts',(14.0399712065491,-5.,74.2740988457103));
#38246=CARTESIAN_POINT('Ctrl Pts',(14.0399712065491,5.,74.2740988457103));
#38247=CARTESIAN_POINT('Ctrl Pts',(14.0244642769439,-5.,74.3176336598548));
#38248=CARTESIAN_POINT('Ctrl Pts',(14.0244642769439,5.,74.3176336598548));
#38249=CARTESIAN_POINT('Ctrl Pts',(14.008534573935,-5.,74.3604652161928));
#38250=CARTESIAN_POINT('Ctrl Pts',(14.008534573935,5.,74.3604652161928));
#38251=CARTESIAN_POINT('Ctrl Pts',(13.9921780472215,-5.,74.4025847861155));
#38252=CARTESIAN_POINT('Ctrl Pts',(13.9921780472215,5.,74.4025847861155));
#38253=CARTESIAN_POINT('Ctrl Pts',(13.9753911574206,-5.,74.4439831150199));
#38254=CARTESIAN_POINT('Ctrl Pts',(13.9753911574206,5.,74.4439831150199));
#38255=CARTESIAN_POINT('Ctrl Pts',(13.9581717227553,-5.,74.4846515525832));
#38256=CARTESIAN_POINT('Ctrl Pts',(13.9581717227553,5.,74.4846515525832));
#38257=CARTESIAN_POINT('Ctrl Pts',(13.9405198648132,-5.,74.5245830312134));
#38258=CARTESIAN_POINT('Ctrl Pts',(13.9405198648132,5.,74.5245830312134));
#38259=CARTESIAN_POINT('Ctrl Pts',(13.922439790982,-5.,74.5637691297076));
#38260=CARTESIAN_POINT('Ctrl Pts',(13.922439790982,5.,74.5637691297076));
#38261=CARTESIAN_POINT('Ctrl Pts',(13.9039414871763,-5.,74.6021976043591));
#38262=CARTESIAN_POINT('Ctrl Pts',(13.9039414871763,5.,74.6021976043591));
#38263=CARTESIAN_POINT('Ctrl Pts',(13.8850428402731,-5.,74.6398496456646));
#38264=CARTESIAN_POINT('Ctrl Pts',(13.8850428402731,5.,74.6398496456646));
#38265=CARTESIAN_POINT('Ctrl Pts',(13.8657711229787,-5.,74.6766979024311));
#38266=CARTESIAN_POINT('Ctrl Pts',(13.8657711229787,5.,74.6766979024311));
#38267=CARTESIAN_POINT('Ctrl Pts',(13.8461663877159,-5.,74.7127029904214));
#38268=CARTESIAN_POINT('Ctrl Pts',(13.8461663877159,5.,74.7127029904214));
#38269=CARTESIAN_POINT('Ctrl Pts',(13.8262787721306,-5.,74.7478155144712));
#38270=CARTESIAN_POINT('Ctrl Pts',(13.8262787721306,5.,74.7478155144712));
#38271=CARTESIAN_POINT('Ctrl Pts',(13.8061583390975,-5.,74.78198479708));
#38272=CARTESIAN_POINT('Ctrl Pts',(13.8061583390975,5.,74.78198479708));
#38273=CARTESIAN_POINT('Ctrl Pts',(13.785846549493,-5.,74.8151663525327));
#38274=CARTESIAN_POINT('Ctrl Pts',(13.785846549493,5.,74.8151663525327));
#38275=CARTESIAN_POINT('Ctrl Pts',(13.7653677857709,-5.,74.8473294704568));
#38276=CARTESIAN_POINT('Ctrl Pts',(13.7653677857709,5.,74.8473294704568));
#38277=CARTESIAN_POINT('Ctrl Pts',(13.7447191217217,-5.,74.8784665452351));
#38278=CARTESIAN_POINT('Ctrl Pts',(13.7447191217217,5.,74.8784665452351));
#38279=CARTESIAN_POINT('Ctrl Pts',(13.7238655514216,-5.,74.9085976920185));
#38280=CARTESIAN_POINT('Ctrl Pts',(13.7238655514216,5.,74.9085976920185));
#38281=CARTESIAN_POINT('Ctrl Pts',(13.7027714681697,-5.,74.9377430766853));
#38282=CARTESIAN_POINT('Ctrl Pts',(13.7027714681697,5.,74.9377430766853));
#38283=CARTESIAN_POINT('Ctrl Pts',(13.6814292842299,-5.,74.9658980076382));
#38284=CARTESIAN_POINT('Ctrl Pts',(13.6814292842299,5.,74.9658980076382));
#38285=CARTESIAN_POINT('Ctrl Pts',(13.6598872657036,-5.,74.9930088670283));
#38286=CARTESIAN_POINT('Ctrl Pts',(13.6598872657036,5.,74.9930088670283));
#38287=CARTESIAN_POINT('Ctrl Pts',(13.6382830094766,-5.,75.0189443033331));
#38288=CARTESIAN_POINT('Ctrl Pts',(13.6382830094766,5.,75.0189443033331));
#38289=CARTESIAN_POINT('Ctrl Pts',(13.6168604503304,-5.,75.0434810160819));
#38290=CARTESIAN_POINT('Ctrl Pts',(13.6168604503304,5.,75.0434810160819));
#38291=CARTESIAN_POINT('Ctrl Pts',(13.5959147036489,-5.,75.0663526853374));
#38292=CARTESIAN_POINT('Ctrl Pts',(13.5959147036489,5.,75.0663526853374));
#38293=CARTESIAN_POINT('Ctrl Pts',(13.5757453800036,-5.,75.0872918528514));
#38294=CARTESIAN_POINT('Ctrl Pts',(13.5757453800036,5.,75.0872918528514));
#38295=CARTESIAN_POINT('Ctrl Pts',(13.556611019215,-5.,75.1060706833974));
#38296=CARTESIAN_POINT('Ctrl Pts',(13.556611019215,5.,75.1060706833974));
#38297=CARTESIAN_POINT('Ctrl Pts',(13.5386716980329,-5.,75.1225531496632));
#38298=CARTESIAN_POINT('Ctrl Pts',(13.5386716980329,5.,75.1225531496632));
#38299=CARTESIAN_POINT('Ctrl Pts',(13.5253334104135,-5.,75.1338579737778));
#38300=CARTESIAN_POINT('Ctrl Pts',(13.5253334104135,5.,75.1338579737778));
#38301=CARTESIAN_POINT('Ctrl Pts',(13.5159086585763,-5.,75.1412736419094));
#38302=CARTESIAN_POINT('Ctrl Pts',(13.5159086585763,5.,75.1412736419094));
#38303=CARTESIAN_POINT('Ctrl Pts',(13.5098822847451,-5.,75.145745907283));
#38304=CARTESIAN_POINT('Ctrl Pts',(13.5098822847451,5.,75.145745907283));
#38305=CARTESIAN_POINT('Ctrl Pts',(13.5069332996928,-5.,75.1478641584586));
#38306=CARTESIAN_POINT('Ctrl Pts',(13.5069332996928,5.,75.1478641584586));
#38307=CARTESIAN_POINT('',(13.5069332996928,0.,75.1478641584586));
#38308=CARTESIAN_POINT('Ctrl Pts',(14.0314999829165,4.8,74.2976442754215));
#38309=CARTESIAN_POINT('Ctrl Pts',(14.0314999829165,3.13333333333333,74.2976442754215));
#38310=CARTESIAN_POINT('Ctrl Pts',(14.0314999829165,1.46666666666667,74.2976442754215));
#38311=CARTESIAN_POINT('Ctrl Pts',(14.0314999829165,-1.73333333333333,74.2976442754215));
#38312=CARTESIAN_POINT('Ctrl Pts',(14.0314999829165,-3.26666666666667,74.2976442754215));
#38313=CARTESIAN_POINT('Ctrl Pts',(14.0314999829165,-4.8,74.2976442754215));
#38314=CARTESIAN_POINT('Origin',(9.31000000000134,0.,77.9999999999992));
#38315=CARTESIAN_POINT('',(13.5204349482691,0.,76.0264910574324));
#38316=CARTESIAN_POINT('',(13.1243263529939,0.,75.340410845101));
#38317=CARTESIAN_POINT('Origin',(13.5069332996928,0.,75.1478641584586));
#38318=CARTESIAN_POINT('Ctrl Pts',(13.8784887436653,-5.,75.7914170652479));
#38319=CARTESIAN_POINT('Ctrl Pts',(13.8784887436653,5.,75.7914170652479));
#38320=CARTESIAN_POINT('Ctrl Pts',(13.8817976955159,-5.,75.7899222948501));
#38321=CARTESIAN_POINT('Ctrl Pts',(13.8817976955159,5.,75.7899222948501));
#38322=CARTESIAN_POINT('Ctrl Pts',(13.8886839778489,-5.,75.7869394346819));
#38323=CARTESIAN_POINT('Ctrl Pts',(13.8886839778489,5.,75.7869394346819));
#38324=CARTESIAN_POINT('Ctrl Pts',(13.8998185107484,-5.,75.7824851942128));
#38325=CARTESIAN_POINT('Ctrl Pts',(13.8998185107484,5.,75.7824851942128));
#38326=CARTESIAN_POINT('Ctrl Pts',(13.9162779194277,-5.,75.7765863103522));
#38327=CARTESIAN_POINT('Ctrl Pts',(13.9162779194277,5.,75.7765863103522));
#38328=CARTESIAN_POINT('Ctrl Pts',(13.9395218145337,-5.,75.7692916356475));
#38329=CARTESIAN_POINT('Ctrl Pts',(13.9395218145337,5.,75.7692916356475));
#38330=CARTESIAN_POINT('Ctrl Pts',(13.9653519392467,-5.,75.762110208427));
#38331=CARTESIAN_POINT('Ctrl Pts',(13.9653519392467,5.,75.762110208427));
#38332=CARTESIAN_POINT('Ctrl Pts',(13.9935704520776,-5.,75.7551126455491));
#38333=CARTESIAN_POINT('Ctrl Pts',(13.9935704520776,5.,75.7551126455491));
#38334=CARTESIAN_POINT('Ctrl Pts',(14.0238507720205,-5.,75.7484089314496));
#38335=CARTESIAN_POINT('Ctrl Pts',(14.0238507720205,5.,75.7484089314496));
#38336=CARTESIAN_POINT('Ctrl Pts',(14.0558114681545,-5.,75.7421248073761));
#38337=CARTESIAN_POINT('Ctrl Pts',(14.0558114681545,5.,75.7421248073761));
#38338=CARTESIAN_POINT('Ctrl Pts',(14.0890743429601,-5.,75.7363826907892));
#38339=CARTESIAN_POINT('Ctrl Pts',(14.0890743429601,5.,75.7363826907892));
#38340=CARTESIAN_POINT('Ctrl Pts',(14.1233240451699,-5.,75.7312821851806));
#38341=CARTESIAN_POINT('Ctrl Pts',(14.1233240451699,5.,75.7312821851806));
#38342=CARTESIAN_POINT('Ctrl Pts',(14.1583780225866,-5.,75.7268767771904));
#38343=CARTESIAN_POINT('Ctrl Pts',(14.1583780225866,5.,75.7268767771904));
#38344=CARTESIAN_POINT('Ctrl Pts',(14.1941657077391,-5.,75.7231814575622));
#38345=CARTESIAN_POINT('Ctrl Pts',(14.1941657077391,5.,75.7231814575622));
#38346=CARTESIAN_POINT('Ctrl Pts',(14.2306868314508,-5.,75.7201873093207));
#38347=CARTESIAN_POINT('Ctrl Pts',(14.2306868314508,5.,75.7201873093207));
#38348=CARTESIAN_POINT('Ctrl Pts',(14.2679766612333,-5.,75.7178735790925));
#38349=CARTESIAN_POINT('Ctrl Pts',(14.2679766612333,5.,75.7178735790925));
#38350=CARTESIAN_POINT('Ctrl Pts',(14.3060701202788,-5.,75.7162200084309));
#38351=CARTESIAN_POINT('Ctrl Pts',(14.3060701202788,5.,75.7162200084309));
#38352=CARTESIAN_POINT('Ctrl Pts',(14.3449620850358,-5.,75.7152202603571));
#38353=CARTESIAN_POINT('Ctrl Pts',(14.3449620850358,5.,75.7152202603571));
#38354=CARTESIAN_POINT('Ctrl Pts',(14.384613768317,-5.,75.7148800955132));
#38355=CARTESIAN_POINT('Ctrl Pts',(14.384613768317,5.,75.7148800955132));
#38356=CARTESIAN_POINT('Ctrl Pts',(14.4249659139274,-5.,75.7152131772188));
#38357=CARTESIAN_POINT('Ctrl Pts',(14.4249659139274,5.,75.7152131772188));
#38358=CARTESIAN_POINT('Ctrl Pts',(14.4659496024287,-5.,75.7162375224487));
#38359=CARTESIAN_POINT('Ctrl Pts',(14.4659496024287,5.,75.7162375224487));
#38360=CARTESIAN_POINT('Ctrl Pts',(14.5074969875316,-5.,75.7179718540974));
#38361=CARTESIAN_POINT('Ctrl Pts',(14.5074969875316,5.,75.7179718540974));
#38362=CARTESIAN_POINT('Ctrl Pts',(14.5495539352719,-5.,75.7204311664575));
#38363=CARTESIAN_POINT('Ctrl Pts',(14.5495539352719,5.,75.7204311664575));
#38364=CARTESIAN_POINT('Ctrl Pts',(14.5920831224634,-5.,75.7236254027807));
#38365=CARTESIAN_POINT('Ctrl Pts',(14.5920831224634,5.,75.7236254027807));
#38366=CARTESIAN_POINT('Ctrl Pts',(14.6350593161544,-5.,75.7275606487953));
#38367=CARTESIAN_POINT('Ctrl Pts',(14.6350593161544,5.,75.7275606487953));
#38368=CARTESIAN_POINT('Ctrl Pts',(14.6784669200218,-5.,75.7322394306956));
#38369=CARTESIAN_POINT('Ctrl Pts',(14.6784669200218,5.,75.7322394306956));
#38370=CARTESIAN_POINT('Ctrl Pts',(14.7222965373945,-5.,75.7376611815812));
#38371=CARTESIAN_POINT('Ctrl Pts',(14.7222965373945,5.,75.7376611815812));
#38372=CARTESIAN_POINT('Ctrl Pts',(14.7665419867663,-5.,75.7438224729572));
#38373=CARTESIAN_POINT('Ctrl Pts',(14.7665419867663,5.,75.7438224729572));
#38374=CARTESIAN_POINT('Ctrl Pts',(14.8111968676342,-5.,75.7507170902014));
#38375=CARTESIAN_POINT('Ctrl Pts',(14.8111968676342,5.,75.7507170902014));
#38376=CARTESIAN_POINT('Ctrl Pts',(14.8562549349808,-5.,75.7583373408378));
#38377=CARTESIAN_POINT('Ctrl Pts',(14.8562549349808,5.,75.7583373408378));
#38378=CARTESIAN_POINT('Ctrl Pts',(14.9017106547726,-5.,75.7666753529216));
#38379=CARTESIAN_POINT('Ctrl Pts',(14.9017106547726,5.,75.7666753529216));
#38380=CARTESIAN_POINT('Ctrl Pts',(14.9383898229867,-5.,75.7739144459592));
#38381=CARTESIAN_POINT('Ctrl Pts',(14.9383898229867,5.,75.7739144459592));
#38382=CARTESIAN_POINT('Ctrl Pts',(14.96607485352,-5.,75.7796614514317));
#38383=CARTESIAN_POINT('Ctrl Pts',(14.96607485352,5.,75.7796614514317));
#38384=CARTESIAN_POINT('Ctrl Pts',(14.984609467824,-5.,75.7836337265846));
#38385=CARTESIAN_POINT('Ctrl Pts',(14.984609467824,5.,75.7836337265846));
#38386=CARTESIAN_POINT('Ctrl Pts',(14.9938962568098,-5.,75.7856550987203));
#38387=CARTESIAN_POINT('Ctrl Pts',(14.9938962568098,5.,75.7856550987203));
#38388=CARTESIAN_POINT('Ctrl Pts',(14.8770841027247,-4.8,75.7622389329533));
#38389=CARTESIAN_POINT('Ctrl Pts',(14.8770841027247,-3.13333333333333,75.7622389329533));
#38390=CARTESIAN_POINT('Ctrl Pts',(14.8770841027247,-1.46666666666667,75.7622389329533));
#38391=CARTESIAN_POINT('Ctrl Pts',(14.8770841027247,1.73333333333333,75.7622389329533));
#38392=CARTESIAN_POINT('Ctrl Pts',(14.8770841027247,3.26666666666667,75.7622389329533));
#38393=CARTESIAN_POINT('Ctrl Pts',(14.8770841027247,4.8,75.7622389329533));
#38394=CARTESIAN_POINT('',(13.8784887436653,0.,75.7914170652479));
#38395=CARTESIAN_POINT('Origin',(13.5204349482691,0.,76.0264910574324));
#38396=CARTESIAN_POINT('Ctrl Pts',(10.5037057995804,-5.,72.0179379421433));
#38397=CARTESIAN_POINT('Ctrl Pts',(10.5037057995804,5.,72.0179379421433));
#38398=CARTESIAN_POINT('Ctrl Pts',(10.507309096492,-5.,72.0267326363238));
#38399=CARTESIAN_POINT('Ctrl Pts',(10.507309096492,5.,72.0267326363238));
#38400=CARTESIAN_POINT('Ctrl Pts',(10.514439525817,-5.,72.0442958898031));
#38401=CARTESIAN_POINT('Ctrl Pts',(10.514439525817,5.,72.0442958898031));
#38402=CARTESIAN_POINT('Ctrl Pts',(10.5249066764203,-5.,72.070562365439));
#38403=CARTESIAN_POINT('Ctrl Pts',(10.5249066764203,5.,72.070562365439));
#38404=CARTESIAN_POINT('Ctrl Pts',(10.5384050620625,-5.,72.1054272393282));
#38405=CARTESIAN_POINT('Ctrl Pts',(10.5384050620625,5.,72.1054272393282));
#38406=CARTESIAN_POINT('Ctrl Pts',(10.554509703925,-5.,72.1487445040063));
#38407=CARTESIAN_POINT('Ctrl Pts',(10.554509703925,5.,72.1487445040063));
#38408=CARTESIAN_POINT('Ctrl Pts',(10.5698384371529,-5.,72.1917947954702));
#38409=CARTESIAN_POINT('Ctrl Pts',(10.5698384371529,5.,72.1917947954702));
#38410=CARTESIAN_POINT('Ctrl Pts',(10.584382548403,-5.,72.2345740306915));
#38411=CARTESIAN_POINT('Ctrl Pts',(10.584382548403,5.,72.2345740306915));
#38412=CARTESIAN_POINT('Ctrl Pts',(10.598133377614,-5.,72.2770773952961));
#38413=CARTESIAN_POINT('Ctrl Pts',(10.598133377614,5.,72.2770773952961));
#38414=CARTESIAN_POINT('Ctrl Pts',(10.6110836931323,-5.,72.3192996651659));
#38415=CARTESIAN_POINT('Ctrl Pts',(10.6110836931323,5.,72.3192996651659));
#38416=CARTESIAN_POINT('Ctrl Pts',(10.6232290451402,-5.,72.3612353480546));
#38417=CARTESIAN_POINT('Ctrl Pts',(10.6232290451402,5.,72.3612353480546));
#38418=CARTESIAN_POINT('Ctrl Pts',(10.6345672436375,-5.,72.4028752884915));
#38419=CARTESIAN_POINT('Ctrl Pts',(10.6345672436375,5.,72.4028752884915));
#38420=CARTESIAN_POINT('Ctrl Pts',(10.6450980681725,-5.,72.4442036884342));
#38421=CARTESIAN_POINT('Ctrl Pts',(10.6450980681725,5.,72.4442036884342));
#38422=CARTESIAN_POINT('Ctrl Pts',(10.6548231303688,-5.,72.4851946415082));
#38423=CARTESIAN_POINT('Ctrl Pts',(10.6548231303688,5.,72.4851946415082));
#38424=CARTESIAN_POINT('Ctrl Pts',(10.6637457413204,-5.,72.5258096649296));
#38425=CARTESIAN_POINT('Ctrl Pts',(10.6637457413204,5.,72.5258096649296));
#38426=CARTESIAN_POINT('Ctrl Pts',(10.6718712672619,-5.,72.5659928434235));
#38427=CARTESIAN_POINT('Ctrl Pts',(10.6718712672619,5.,72.5659928434235));
#38428=CARTESIAN_POINT('Ctrl Pts',(10.6792063652593,-5.,72.6056741102406));
#38429=CARTESIAN_POINT('Ctrl Pts',(10.6792063652593,5.,72.6056741102406));
#38430=CARTESIAN_POINT('Ctrl Pts',(10.6857568108318,-5.,72.6447824643664));
#38431=CARTESIAN_POINT('Ctrl Pts',(10.6857568108318,5.,72.6447824643664));
#38432=CARTESIAN_POINT('Ctrl Pts',(10.6915257699882,-5.,72.6832571772262));
#38433=CARTESIAN_POINT('Ctrl Pts',(10.6915257699882,5.,72.6832571772262));
#38434=CARTESIAN_POINT('Ctrl Pts',(10.6965121805263,-5.,72.721059050569));
#38435=CARTESIAN_POINT('Ctrl Pts',(10.6965121805263,5.,72.721059050569));
#38436=CARTESIAN_POINT('Ctrl Pts',(10.7007089120438,-5.,72.7581841390844));
#38437=CARTESIAN_POINT('Ctrl Pts',(10.7007089120438,5.,72.7581841390844));
#38438=CARTESIAN_POINT('Ctrl Pts',(10.704102078216,-5.,72.794670353247));
#38439=CARTESIAN_POINT('Ctrl Pts',(10.704102078216,5.,72.794670353247));
#38440=CARTESIAN_POINT('Ctrl Pts',(10.7066773651029,-5.,72.8305560285639));
#38441=CARTESIAN_POINT('Ctrl Pts',(10.7066773651029,5.,72.8305560285639));
#38442=CARTESIAN_POINT('Ctrl Pts',(10.7084259444594,-5.,72.8658424483676));
#38443=CARTESIAN_POINT('Ctrl Pts',(10.7084259444594,5.,72.8658424483676));
#38444=CARTESIAN_POINT('Ctrl Pts',(10.7093503253745,-5.,72.9004575141518));
#38445=CARTESIAN_POINT('Ctrl Pts',(10.7093503253745,5.,72.9004575141518));
#38446=CARTESIAN_POINT('Ctrl Pts',(10.7094714820477,-5.,72.9342121592384));
#38447=CARTESIAN_POINT('Ctrl Pts',(10.7094714820477,5.,72.9342121592384));
#38448=CARTESIAN_POINT('Ctrl Pts',(10.7088327445899,-5.,72.966778527284));
#38449=CARTESIAN_POINT('Ctrl Pts',(10.7088327445899,5.,72.966778527284));
#38450=CARTESIAN_POINT('Ctrl Pts',(10.707488997348,-5.,72.9977629088648));
#38451=CARTESIAN_POINT('Ctrl Pts',(10.707488997348,5.,72.9977629088648));
#38452=CARTESIAN_POINT('Ctrl Pts',(10.7054978364887,-5.,73.0267678331103));
#38453=CARTESIAN_POINT('Ctrl Pts',(10.7054978364887,5.,73.0267678331103));
#38454=CARTESIAN_POINT('Ctrl Pts',(10.7029108653431,-5.,73.0534525819188));
#38455=CARTESIAN_POINT('Ctrl Pts',(10.7029108653431,5.,73.0534525819188));
#38456=CARTESIAN_POINT('Ctrl Pts',(10.6997632731399,-5.,73.0776100569794));
#38457=CARTESIAN_POINT('Ctrl Pts',(10.6997632731399,5.,73.0776100569794));
#38458=CARTESIAN_POINT('Ctrl Pts',(10.6968121528997,-5.,73.0948437406871));
#38459=CARTESIAN_POINT('Ctrl Pts',(10.6968121528997,5.,73.0948437406871));
#38460=CARTESIAN_POINT('Ctrl Pts',(10.6943590737142,-5.,73.1065825857645));
#38461=CARTESIAN_POINT('Ctrl Pts',(10.6943590737142,5.,73.1065825857645));
#38462=CARTESIAN_POINT('Ctrl Pts',(10.6926173202913,-5.,73.1138822182422));
#38463=CARTESIAN_POINT('Ctrl Pts',(10.6926173202913,5.,73.1138822182422));
#38464=CARTESIAN_POINT('Ctrl Pts',(10.691719852285,-5.,73.1174004638434));
#38465=CARTESIAN_POINT('Ctrl Pts',(10.691719852285,5.,73.1174004638434));
#38466=CARTESIAN_POINT('',(10.691719852285,0.,73.1174004638434));
#38467=CARTESIAN_POINT('Ctrl Pts',(10.5470504387829,4.8,72.1289092826028));
#38468=CARTESIAN_POINT('Ctrl Pts',(10.5470504387829,3.13333333333333,72.1289092826028));
#38469=CARTESIAN_POINT('Ctrl Pts',(10.5470504387829,1.46666666666667,72.1289092826028));
#38470=CARTESIAN_POINT('Ctrl Pts',(10.5470504387829,-1.73333333333333,72.1289092826028));
#38471=CARTESIAN_POINT('Ctrl Pts',(10.5470504387829,-3.26666666666667,72.1289092826028));
#38472=CARTESIAN_POINT('Ctrl Pts',(10.5470504387829,-4.8,72.1289092826028));
#38473=CARTESIAN_POINT('Origin',(9.31000000000015,0.,77.9999999999997));
#38474=CARTESIAN_POINT('',(11.2668331993474,0.,73.7817890249619));
#38475=CARTESIAN_POINT('',(10.5223925513275,0.,73.5108347879048));
#38476=CARTESIAN_POINT('Origin',(10.691719852285,0.,73.1174004638434));
#38477=CARTESIAN_POINT('Ctrl Pts',(11.3900156701126,-5.,73.3715593562453));
#38478=CARTESIAN_POINT('Ctrl Pts',(11.3900156701126,5.,73.3715593562453));
#38479=CARTESIAN_POINT('Ctrl Pts',(11.3915896544057,-5.,73.3682873424408));
#38480=CARTESIAN_POINT('Ctrl Pts',(11.3915896544057,5.,73.3682873424408));
#38481=CARTESIAN_POINT('Ctrl Pts',(11.3949475071735,-5.,73.361575922029));
#38482=CARTESIAN_POINT('Ctrl Pts',(11.3949475071735,5.,73.361575922029));
#38483=CARTESIAN_POINT('Ctrl Pts',(11.4006139236521,-5.,73.3510066360857));
#38484=CARTESIAN_POINT('Ctrl Pts',(11.4006139236521,5.,73.3510066360857));
#38485=CARTESIAN_POINT('Ctrl Pts',(11.4094308327498,-5.,73.3359079249211));
#38486=CARTESIAN_POINT('Ctrl Pts',(11.4094308327498,5.,73.3359079249211));
#38487=CARTESIAN_POINT('Ctrl Pts',(11.4225477629013,-5.,73.3153789921175));
#38488=CARTESIAN_POINT('Ctrl Pts',(11.4225477629013,5.,73.3153789921175));
#38489=CARTESIAN_POINT('Ctrl Pts',(11.4377186539509,-5.,73.2932744155724));
#38490=CARTESIAN_POINT('Ctrl Pts',(11.4377186539509,5.,73.2932744155724));
#38491=CARTESIAN_POINT('Ctrl Pts',(11.454837342174,-5.,73.2697754609989));
#38492=CARTESIAN_POINT('Ctrl Pts',(11.454837342174,5.,73.2697754609989));
#38493=CARTESIAN_POINT('Ctrl Pts',(11.47372434864,-5.,73.2451763035876));
#38494=CARTESIAN_POINT('Ctrl Pts',(11.47372434864,5.,73.2451763035876));
#38495=CARTESIAN_POINT('Ctrl Pts',(11.4941683052251,-5.,73.2198184457917));
#38496=CARTESIAN_POINT('Ctrl Pts',(11.4941683052251,5.,73.2198184457917));
#38497=CARTESIAN_POINT('Ctrl Pts',(11.5159581842438,-5.,73.1940387655048));
#38498=CARTESIAN_POINT('Ctrl Pts',(11.5159581842438,5.,73.1940387655048));
#38499=CARTESIAN_POINT('Ctrl Pts',(11.5389164364967,-5.,73.1681162673142));
#38500=CARTESIAN_POINT('Ctrl Pts',(11.5389164364967,5.,73.1681162673142));
#38501=CARTESIAN_POINT('Ctrl Pts',(11.5629375994355,-5.,73.1422092666525));
#38502=CARTESIAN_POINT('Ctrl Pts',(11.5629375994355,5.,73.1422092666525));
#38503=CARTESIAN_POINT('Ctrl Pts',(11.5879772511062,-5.,73.116374606991));
#38504=CARTESIAN_POINT('Ctrl Pts',(11.5879772511062,5.,73.116374606991));
#38505=CARTESIAN_POINT('Ctrl Pts',(11.6140294535881,-5.,73.0906056305532));
#38506=CARTESIAN_POINT('Ctrl Pts',(11.6140294535881,5.,73.0906056305532));
#38507=CARTESIAN_POINT('Ctrl Pts',(11.6411078833532,-5.,73.0648637698139));
#38508=CARTESIAN_POINT('Ctrl Pts',(11.6411078833532,5.,73.0648637698139));
#38509=CARTESIAN_POINT('Ctrl Pts',(11.6692262712418,-5.,73.039111057708));
#38510=CARTESIAN_POINT('Ctrl Pts',(11.6692262712418,5.,73.039111057708));
#38511=CARTESIAN_POINT('Ctrl Pts',(11.6983766190533,-5.,73.0133459331853));
#38512=CARTESIAN_POINT('Ctrl Pts',(11.6983766190533,5.,73.0133459331853));
#38513=CARTESIAN_POINT('Ctrl Pts',(11.7285329169467,-5.,72.9875977410784));
#38514=CARTESIAN_POINT('Ctrl Pts',(11.7285329169467,5.,72.9875977410784));
#38515=CARTESIAN_POINT('Ctrl Pts',(11.7596585546536,-5.,72.9619150372466));
#38516=CARTESIAN_POINT('Ctrl Pts',(11.7596585546536,5.,72.9619150372466));
#38517=CARTESIAN_POINT('Ctrl Pts',(11.7917123179081,-5.,72.9363559240547));
#38518=CARTESIAN_POINT('Ctrl Pts',(11.7917123179081,5.,72.9363559240547));
#38519=CARTESIAN_POINT('Ctrl Pts',(11.8246542682811,-5.,72.9109783548261));
#38520=CARTESIAN_POINT('Ctrl Pts',(11.8246542682811,5.,72.9109783548261));
#38521=CARTESIAN_POINT('Ctrl Pts',(11.8584525748975,-5.,72.8858286124943));
#38522=CARTESIAN_POINT('Ctrl Pts',(11.8584525748975,5.,72.8858286124943));
#38523=CARTESIAN_POINT('Ctrl Pts',(11.8930850379397,-5.,72.8609383049106));
#38524=CARTESIAN_POINT('Ctrl Pts',(11.8930850379397,5.,72.8609383049106));
#38525=CARTESIAN_POINT('Ctrl Pts',(11.9285362396797,-5.,72.8363283134386));
#38526=CARTESIAN_POINT('Ctrl Pts',(11.9285362396797,5.,72.8363283134386));
#38527=CARTESIAN_POINT('Ctrl Pts',(11.9647958564499,-5.,72.8120105983759));
#38528=CARTESIAN_POINT('Ctrl Pts',(11.9647958564499,5.,72.8120105983759));
#38529=CARTESIAN_POINT('Ctrl Pts',(12.0018563255875,-5.,72.7879907655145));
#38530=CARTESIAN_POINT('Ctrl Pts',(12.0018563255875,5.,72.7879907655145));
#38531=CARTESIAN_POINT('Ctrl Pts',(12.0397107079891,-5.,72.7642701618722));
#38532=CARTESIAN_POINT('Ctrl Pts',(12.0397107079891,5.,72.7642701618722));
#38533=CARTESIAN_POINT('Ctrl Pts',(12.0783501058978,-5.,72.7408481409417));
#38534=CARTESIAN_POINT('Ctrl Pts',(12.0783501058978,5.,72.7408481409417));
#38535=CARTESIAN_POINT('Ctrl Pts',(12.1177647907168,-5.,72.7177228241715));
#38536=CARTESIAN_POINT('Ctrl Pts',(12.1177647907168,5.,72.7177228241715));
#38537=CARTESIAN_POINT('Ctrl Pts',(12.1579454631339,-5.,72.6948917385186));
#38538=CARTESIAN_POINT('Ctrl Pts',(12.1579454631339,5.,72.6948917385186));
#38539=CARTESIAN_POINT('Ctrl Pts',(12.1906965354202,-5.,72.6768602906647));
#38540=CARTESIAN_POINT('Ctrl Pts',(12.1906965354202,5.,72.6768602906647));
#38541=CARTESIAN_POINT('Ctrl Pts',(12.2155986031066,-5.,72.6634671576927));
#38542=CARTESIAN_POINT('Ctrl Pts',(12.2155986031066,5.,72.6634671576927));
#38543=CARTESIAN_POINT('Ctrl Pts',(12.2323502706299,-5.,72.6545962765953));
#38544=CARTESIAN_POINT('Ctrl Pts',(12.2323502706299,5.,72.6545962765953));
#38545=CARTESIAN_POINT('Ctrl Pts',(12.2407636766788,-5.,72.6501753046048));
#38546=CARTESIAN_POINT('Ctrl Pts',(12.2407636766788,5.,72.6501753046048));
#38547=CARTESIAN_POINT('Ctrl Pts',(12.1362287539071,-4.8,72.7073228862334));
#38548=CARTESIAN_POINT('Ctrl Pts',(12.1362287539071,-3.13333333333333,72.7073228862334));
#38549=CARTESIAN_POINT('Ctrl Pts',(12.1362287539071,-1.46666666666667,72.7073228862334));
#38550=CARTESIAN_POINT('Ctrl Pts',(12.1362287539071,1.73333333333333,72.7073228862334));
#38551=CARTESIAN_POINT('Ctrl Pts',(12.1362287539072,3.26666666666667,72.7073228862334));
#38552=CARTESIAN_POINT('Ctrl Pts',(12.1362287539072,4.8,72.7073228862334));
#38553=CARTESIAN_POINT('',(11.3900156701126,0.,73.3715593562453));
#38554=CARTESIAN_POINT('Origin',(11.2668331993474,0.,73.7817890249619));
#38555=CARTESIAN_POINT('Ctrl Pts',(6.37923632332121,-5.,72.6501753046048));
#38556=CARTESIAN_POINT('Ctrl Pts',(6.37923632332121,5.,72.6501753046048));
#38557=CARTESIAN_POINT('Ctrl Pts',(6.38764972936496,-5.,72.6545962765957));
#38558=CARTESIAN_POINT('Ctrl Pts',(6.38764972936496,5.,72.6545962765957));
#38559=CARTESIAN_POINT('Ctrl Pts',(6.40440139687937,-5.,72.6634671576939));
#38560=CARTESIAN_POINT('Ctrl Pts',(6.40440139687937,5.,72.6634671576939));
#38561=CARTESIAN_POINT('Ctrl Pts',(6.42930346455622,-5.,72.6768602906668));
#38562=CARTESIAN_POINT('Ctrl Pts',(6.42930346455622,5.,72.6768602906668));
#38563=CARTESIAN_POINT('Ctrl Pts',(6.462054536837,-5.,72.6948917385213));
#38564=CARTESIAN_POINT('Ctrl Pts',(6.462054536837,5.,72.6948917385213));
#38565=CARTESIAN_POINT('Ctrl Pts',(6.50223520925657,-5.,72.7177228241743));
#38566=CARTESIAN_POINT('Ctrl Pts',(6.50223520925657,5.,72.7177228241743));
#38567=CARTESIAN_POINT('Ctrl Pts',(6.54164989408384,-5.,72.7408481409439));
#38568=CARTESIAN_POINT('Ctrl Pts',(6.54164989408384,5.,72.7408481409439));
#38569=CARTESIAN_POINT('Ctrl Pts',(6.58028929200299,-5.,72.7642701618733));
#38570=CARTESIAN_POINT('Ctrl Pts',(6.58028929200299,5.,72.7642701618733));
#38571=CARTESIAN_POINT('Ctrl Pts',(6.61814367441384,-5.,72.7879907655144));
#38572=CARTESIAN_POINT('Ctrl Pts',(6.61814367441384,5.,72.7879907655144));
#38573=CARTESIAN_POINT('Ctrl Pts',(6.65520414355746,-5.,72.8120105983748));
#38574=CARTESIAN_POINT('Ctrl Pts',(6.65520414355746,5.,72.8120105983748));
#38575=CARTESIAN_POINT('Ctrl Pts',(6.6914637603298,-5.,72.8363283134371));
#38576=CARTESIAN_POINT('Ctrl Pts',(6.6914637603298,5.,72.8363283134371));
#38577=CARTESIAN_POINT('Ctrl Pts',(6.72691496206853,-5.,72.860938304909));
#38578=CARTESIAN_POINT('Ctrl Pts',(6.72691496206853,5.,72.860938304909));
#38579=CARTESIAN_POINT('Ctrl Pts',(6.76154742510752,-5.,72.8858286124932));
#38580=CARTESIAN_POINT('Ctrl Pts',(6.76154742510752,5.,72.8858286124932));
#38581=CARTESIAN_POINT('Ctrl Pts',(6.79534573172022,-5.,72.9109783548257));
#38582=CARTESIAN_POINT('Ctrl Pts',(6.79534573172022,5.,72.9109783548257));
#38583=CARTESIAN_POINT('Ctrl Pts',(6.82828768209052,-5.,72.9363559240551));
#38584=CARTESIAN_POINT('Ctrl Pts',(6.82828768209052,5.,72.9363559240551));
#38585=CARTESIAN_POINT('Ctrl Pts',(6.86034144534386,-5.,72.9619150372476));
#38586=CARTESIAN_POINT('Ctrl Pts',(6.86034144534386,5.,72.9619150372476));
#38587=CARTESIAN_POINT('Ctrl Pts',(6.89146708305094,-5.,72.9875977410796));
#38588=CARTESIAN_POINT('Ctrl Pts',(6.89146708305094,5.,72.9875977410796));
#38589=CARTESIAN_POINT('Ctrl Pts',(6.92162338094535,-5.,73.0133459331862));
#38590=CARTESIAN_POINT('Ctrl Pts',(6.92162338094535,5.,73.0133459331862));
#38591=CARTESIAN_POINT('Ctrl Pts',(6.95077372875798,-5.,73.0391110577085));
#38592=CARTESIAN_POINT('Ctrl Pts',(6.95077372875798,5.,73.0391110577085));
#38593=CARTESIAN_POINT('Ctrl Pts',(6.97889211664697,-5.,73.0648637698137));
#38594=CARTESIAN_POINT('Ctrl Pts',(6.97889211664697,5.,73.0648637698137));
#38595=CARTESIAN_POINT('Ctrl Pts',(7.0059705464117,-5.,73.0906056305525));
#38596=CARTESIAN_POINT('Ctrl Pts',(7.0059705464117,5.,73.0906056305525));
#38597=CARTESIAN_POINT('Ctrl Pts',(7.03202274889284,-5.,73.1163746069901));
#38598=CARTESIAN_POINT('Ctrl Pts',(7.03202274889284,5.,73.1163746069901));
#38599=CARTESIAN_POINT('Ctrl Pts',(7.05706240056292,-5.,73.1422092666518));
#38600=CARTESIAN_POINT('Ctrl Pts',(7.05706240056292,5.,73.1422092666518));
#38601=CARTESIAN_POINT('Ctrl Pts',(7.08108356350204,-5.,73.1681162673139));
#38602=CARTESIAN_POINT('Ctrl Pts',(7.08108356350204,5.,73.1681162673139));
#38603=CARTESIAN_POINT('Ctrl Pts',(7.10404181575629,-5.,73.1940387655049));
#38604=CARTESIAN_POINT('Ctrl Pts',(7.10404181575629,5.,73.1940387655049));
#38605=CARTESIAN_POINT('Ctrl Pts',(7.12583169477727,-5.,73.2198184457921));
#38606=CARTESIAN_POINT('Ctrl Pts',(7.12583169477727,5.,73.2198184457921));
#38607=CARTESIAN_POINT('Ctrl Pts',(7.14627565136417,-5.,73.2451763035882));
#38608=CARTESIAN_POINT('Ctrl Pts',(7.14627565136417,5.,73.2451763035882));
#38609=CARTESIAN_POINT('Ctrl Pts',(7.16516265783021,-5.,73.2697754609995));
#38610=CARTESIAN_POINT('Ctrl Pts',(7.16516265783021,5.,73.2697754609995));
#38611=CARTESIAN_POINT('Ctrl Pts',(7.18228134605072,-5.,73.2932744155726));
#38612=CARTESIAN_POINT('Ctrl Pts',(7.18228134605072,5.,73.2932744155726));
#38613=CARTESIAN_POINT('Ctrl Pts',(7.19745223709556,-5.,73.3153789921172));
#38614=CARTESIAN_POINT('Ctrl Pts',(7.19745223709556,5.,73.3153789921172));
#38615=CARTESIAN_POINT('Ctrl Pts',(7.21056916724262,-5.,73.3359079249202));
#38616=CARTESIAN_POINT('Ctrl Pts',(7.21056916724262,5.,73.3359079249202));
#38617=CARTESIAN_POINT('Ctrl Pts',(7.21938607633981,-5.,73.3510066360849));
#38618=CARTESIAN_POINT('Ctrl Pts',(7.21938607633981,5.,73.3510066360849));
#38619=CARTESIAN_POINT('Ctrl Pts',(7.22505249282115,-5.,73.3615759220285));
#38620=CARTESIAN_POINT('Ctrl Pts',(7.22505249282115,5.,73.3615759220285));
#38621=CARTESIAN_POINT('Ctrl Pts',(7.22841034559228,-5.,73.3682873424406));
#38622=CARTESIAN_POINT('Ctrl Pts',(7.22841034559228,5.,73.3682873424406));
#38623=CARTESIAN_POINT('Ctrl Pts',(7.22998432988738,-5.,73.3715593562453));
#38624=CARTESIAN_POINT('Ctrl Pts',(7.22998432988738,5.,73.3715593562453));
#38625=CARTESIAN_POINT('',(7.22998432988738,0.,73.3715593562453));
#38626=CARTESIAN_POINT('Ctrl Pts',(6.48377124607659,4.8,72.7073228862421));
#38627=CARTESIAN_POINT('Ctrl Pts',(6.48377124607659,3.13333333333333,72.7073228862421));
#38628=CARTESIAN_POINT('Ctrl Pts',(6.48377124607659,1.46666666666667,72.7073228862421));
#38629=CARTESIAN_POINT('Ctrl Pts',(6.48377124607659,-1.73333333333333,72.7073228862421));
#38630=CARTESIAN_POINT('Ctrl Pts',(6.48377124607658,-3.26666666666667,72.7073228862421));
#38631=CARTESIAN_POINT('Ctrl Pts',(6.48377124607658,-4.8,72.7073228862421));
#38632=CARTESIAN_POINT('Origin',(9.30999999999986,0.,77.9999999999997));
#38633=CARTESIAN_POINT('',(8.09760744867254,0.,73.5108347879048));
#38634=CARTESIAN_POINT('',(7.3531668006526,0.,73.7817890249619));
#38635=CARTESIAN_POINT('Origin',(7.22998432988738,0.,73.3715593562453));
#38636=CARTESIAN_POINT('Ctrl Pts',(7.92828014771504,-5.,73.1174004638434));
#38637=CARTESIAN_POINT('Ctrl Pts',(7.92828014771504,5.,73.1174004638434));
#38638=CARTESIAN_POINT('Ctrl Pts',(7.92738267970718,-5.,73.1138822182422));
#38639=CARTESIAN_POINT('Ctrl Pts',(7.92738267970718,5.,73.1138822182422));
#38640=CARTESIAN_POINT('Ctrl Pts',(7.92564092628179,-5.,73.1065825857644));
#38641=CARTESIAN_POINT('Ctrl Pts',(7.92564092628179,5.,73.1065825857644));
#38642=CARTESIAN_POINT('Ctrl Pts',(7.92318784709425,-5.,73.094843740687));
#38643=CARTESIAN_POINT('Ctrl Pts',(7.92318784709425,5.,73.094843740687));
#38644=CARTESIAN_POINT('Ctrl Pts',(7.92023672685439,-5.,73.0776100569793));
#38645=CARTESIAN_POINT('Ctrl Pts',(7.92023672685439,5.,73.0776100569793));
#38646=CARTESIAN_POINT('Ctrl Pts',(7.91708913465458,-5.,73.0534525819187));
#38647=CARTESIAN_POINT('Ctrl Pts',(7.91708913465458,5.,73.0534525819187));
#38648=CARTESIAN_POINT('Ctrl Pts',(7.91450216351248,-5.,73.0267678331104));
#38649=CARTESIAN_POINT('Ctrl Pts',(7.91450216351248,5.,73.0267678331104));
#38650=CARTESIAN_POINT('Ctrl Pts',(7.91251100265505,-5.,72.9977629088649));
#38651=CARTESIAN_POINT('Ctrl Pts',(7.91251100265505,5.,72.9977629088649));
#38652=CARTESIAN_POINT('Ctrl Pts',(7.91116725541302,-5.,72.9667785272839));
#38653=CARTESIAN_POINT('Ctrl Pts',(7.91116725541302,5.,72.9667785272839));
#38654=CARTESIAN_POINT('Ctrl Pts',(7.91052851795384,-5.,72.9342121592381));
#38655=CARTESIAN_POINT('Ctrl Pts',(7.91052851795384,5.,72.9342121592381));
#38656=CARTESIAN_POINT('Ctrl Pts',(7.91064967462551,-5.,72.9004575141517));
#38657=CARTESIAN_POINT('Ctrl Pts',(7.91064967462551,5.,72.9004575141517));
#38658=CARTESIAN_POINT('Ctrl Pts',(7.91157405553992,-5.,72.865842448368));
#38659=CARTESIAN_POINT('Ctrl Pts',(7.91157405553992,5.,72.865842448368));
#38660=CARTESIAN_POINT('Ctrl Pts',(7.91332263489659,-5.,72.8305560285648));
#38661=CARTESIAN_POINT('Ctrl Pts',(7.91332263489659,5.,72.8305560285648));
#38662=CARTESIAN_POINT('Ctrl Pts',(7.91589792178415,-5.,72.7946703532482));
#38663=CARTESIAN_POINT('Ctrl Pts',(7.91589792178415,5.,72.7946703532482));
#38664=CARTESIAN_POINT('Ctrl Pts',(7.91929108795688,-5.,72.7581841390853));
#38665=CARTESIAN_POINT('Ctrl Pts',(7.91929108795688,5.,72.7581841390853));
#38666=CARTESIAN_POINT('Ctrl Pts',(7.92348781947401,-5.,72.7210590505692));
#38667=CARTESIAN_POINT('Ctrl Pts',(7.92348781947401,5.,72.7210590505692));
#38668=CARTESIAN_POINT('Ctrl Pts',(7.92847423001087,-5.,72.6832571772255));
#38669=CARTESIAN_POINT('Ctrl Pts',(7.92847423001087,5.,72.6832571772255));
#38670=CARTESIAN_POINT('Ctrl Pts',(7.93424318916555,-5.,72.644782464365));
#38671=CARTESIAN_POINT('Ctrl Pts',(7.93424318916555,5.,72.644782464365));
#38672=CARTESIAN_POINT('Ctrl Pts',(7.94079363473673,-5.,72.605674110239));
#38673=CARTESIAN_POINT('Ctrl Pts',(7.94079363473673,5.,72.605674110239));
#38674=CARTESIAN_POINT('Ctrl Pts',(7.94812873273426,-5.,72.5659928434222));
#38675=CARTESIAN_POINT('Ctrl Pts',(7.94812873273426,5.,72.5659928434222));
#38676=CARTESIAN_POINT('Ctrl Pts',(7.95625425867768,-5.,72.525809664929));
#38677=CARTESIAN_POINT('Ctrl Pts',(7.95625425867768,5.,72.525809664929));
#38678=CARTESIAN_POINT('Ctrl Pts',(7.96517686963318,-5.,72.4851946415088));
#38679=CARTESIAN_POINT('Ctrl Pts',(7.96517686963318,5.,72.4851946415088));
#38680=CARTESIAN_POINT('Ctrl Pts',(7.97490193183421,-5.,72.4442036884359));
#38681=CARTESIAN_POINT('Ctrl Pts',(7.97490193183421,5.,72.4442036884359));
#38682=CARTESIAN_POINT('Ctrl Pts',(7.98543275637321,-5.,72.4028752884941));
#38683=CARTESIAN_POINT('Ctrl Pts',(7.98543275637321,5.,72.4028752884941));
#38684=CARTESIAN_POINT('Ctrl Pts',(7.99677095487184,-5.,72.3612353480572));
#38685=CARTESIAN_POINT('Ctrl Pts',(7.99677095487184,5.,72.3612353480572));
#38686=CARTESIAN_POINT('Ctrl Pts',(8.00891630687688,-5.,72.3192996651676));
#38687=CARTESIAN_POINT('Ctrl Pts',(8.00891630687688,5.,72.3192996651676));
#38688=CARTESIAN_POINT('Ctrl Pts',(8.0218666223877,-5.,72.2770773952963));
#38689=CARTESIAN_POINT('Ctrl Pts',(8.0218666223877,5.,72.2770773952963));
#38690=CARTESIAN_POINT('Ctrl Pts',(8.03561745158717,-5.,72.2345740306898));
#38691=CARTESIAN_POINT('Ctrl Pts',(8.03561745158717,5.,72.2345740306898));
#38692=CARTESIAN_POINT('Ctrl Pts',(8.05016156282452,-5.,72.1917947954671));
#38693=CARTESIAN_POINT('Ctrl Pts',(8.05016156282452,5.,72.1917947954671));
#38694=CARTESIAN_POINT('Ctrl Pts',(8.06549029604253,-5.,72.1487445040024));
#38695=CARTESIAN_POINT('Ctrl Pts',(8.06549029604253,5.,72.1487445040024));
#38696=CARTESIAN_POINT('Ctrl Pts',(8.0815949379022,-5.,72.1054272393244));
#38697=CARTESIAN_POINT('Ctrl Pts',(8.0815949379022,5.,72.1054272393244));
#38698=CARTESIAN_POINT('Ctrl Pts',(8.09509332355121,-5.,72.0705623654361));
#38699=CARTESIAN_POINT('Ctrl Pts',(8.09509332355121,5.,72.0705623654361));
#38700=CARTESIAN_POINT('Ctrl Pts',(8.10556047416611,-5.,72.0442958898015));
#38701=CARTESIAN_POINT('Ctrl Pts',(8.10556047416611,5.,72.0442958898015));
#38702=CARTESIAN_POINT('Ctrl Pts',(8.11269090350187,-5.,72.0267326363232));
#38703=CARTESIAN_POINT('Ctrl Pts',(8.11269090350187,5.,72.0267326363232));
#38704=CARTESIAN_POINT('Ctrl Pts',(8.11629420041963,-5.,72.0179379421433));
#38705=CARTESIAN_POINT('Ctrl Pts',(8.11629420041963,5.,72.0179379421433));
#38706=CARTESIAN_POINT('Ctrl Pts',(8.07294956118024,-4.8,72.1289092826106));
#38707=CARTESIAN_POINT('Ctrl Pts',(8.07294956118024,-3.13333333333333,72.1289092826106));
#38708=CARTESIAN_POINT('Ctrl Pts',(8.07294956118024,-1.46666666666667,72.1289092826106));
#38709=CARTESIAN_POINT('Ctrl Pts',(8.07294956118024,1.73333333333333,72.1289092826106));
#38710=CARTESIAN_POINT('Ctrl Pts',(8.07294956118024,3.26666666666667,72.1289092826106));
#38711=CARTESIAN_POINT('Ctrl Pts',(8.07294956118024,4.8,72.1289092826106));
#38712=CARTESIAN_POINT('',(7.92828014771504,0.,73.1174004638434));
#38713=CARTESIAN_POINT('Origin',(8.09760744867254,0.,73.5108347879048));
#38714=CARTESIAN_POINT('Ctrl Pts',(3.62610374319018,-5.,75.7856550987203));
#38715=CARTESIAN_POINT('Ctrl Pts',(3.62610374319018,5.,75.7856550987203));
#38716=CARTESIAN_POINT('Ctrl Pts',(3.63539053217141,-5.,75.7836337265843));
#38717=CARTESIAN_POINT('Ctrl Pts',(3.63539053217141,5.,75.7836337265843));
#38718=CARTESIAN_POINT('Ctrl Pts',(3.65392514646738,-5.,75.7796614514307));
#38719=CARTESIAN_POINT('Ctrl Pts',(3.65392514646738,5.,75.7796614514307));
#38720=CARTESIAN_POINT('Ctrl Pts',(3.68161017699202,-5.,75.7739144459574));
#38721=CARTESIAN_POINT('Ctrl Pts',(3.68161017699202,5.,75.7739144459574));
#38722=CARTESIAN_POINT('Ctrl Pts',(3.71828934520109,-5.,75.7666753529192));
#38723=CARTESIAN_POINT('Ctrl Pts',(3.71828934520109,5.,75.7666753529192));
#38724=CARTESIAN_POINT('Ctrl Pts',(3.76374506499515,-5.,75.7583373408352));
#38725=CARTESIAN_POINT('Ctrl Pts',(3.76374506499515,5.,75.7583373408352));
#38726=CARTESIAN_POINT('Ctrl Pts',(3.80880313234912,-5.,75.7507170901994));
#38727=CARTESIAN_POINT('Ctrl Pts',(3.80880313234912,5.,75.7507170901994));
#38728=CARTESIAN_POINT('Ctrl Pts',(3.85345801322648,-5.,75.7438224729561));
#38729=CARTESIAN_POINT('Ctrl Pts',(3.85345801322648,5.,75.7438224729561));
#38730=CARTESIAN_POINT('Ctrl Pts',(3.89770346260673,-5.,75.7376611815813));
#38731=CARTESIAN_POINT('Ctrl Pts',(3.89770346260673,5.,75.7376611815813));
#38732=CARTESIAN_POINT('Ctrl Pts',(3.94153307998487,-5.,75.7322394306968));
#38733=CARTESIAN_POINT('Ctrl Pts',(3.94153307998487,5.,75.7322394306968));
#38734=CARTESIAN_POINT('Ctrl Pts',(3.98494068385426,-5.,75.7275606487971));
#38735=CARTESIAN_POINT('Ctrl Pts',(3.98494068385426,5.,75.7275606487971));
#38736=CARTESIAN_POINT('Ctrl Pts',(4.02791687754424,-5.,75.7236254027825));
#38737=CARTESIAN_POINT('Ctrl Pts',(4.02791687754424,5.,75.7236254027825));
#38738=CARTESIAN_POINT('Ctrl Pts',(4.07044606473286,-5.,75.7204311664588));
#38739=CARTESIAN_POINT('Ctrl Pts',(4.07044606473286,5.,75.7204311664588));
#38740=CARTESIAN_POINT('Ctrl Pts',(4.11250301246975,-5.,75.7179718540979));
#38741=CARTESIAN_POINT('Ctrl Pts',(4.11250301246975,5.,75.7179718540979));
#38742=CARTESIAN_POINT('Ctrl Pts',(4.1540503975699,-5.,75.7162375224483));
#38743=CARTESIAN_POINT('Ctrl Pts',(4.1540503975699,5.,75.7162375224483));
#38744=CARTESIAN_POINT('Ctrl Pts',(4.19503408607005,-5.,75.7152131772181));
#38745=CARTESIAN_POINT('Ctrl Pts',(4.19503408607005,5.,75.7152131772181));
#38746=CARTESIAN_POINT('Ctrl Pts',(4.23538623168054,-5.,75.7148800955126));
#38747=CARTESIAN_POINT('Ctrl Pts',(4.23538623168054,5.,75.7148800955126));
#38748=CARTESIAN_POINT('Ctrl Pts',(4.27503791496266,-5.,75.7152202603568));
#38749=CARTESIAN_POINT('Ctrl Pts',(4.27503791496266,5.,75.7152202603568));
#38750=CARTESIAN_POINT('Ctrl Pts',(4.31392987972073,-5.,75.7162200084309));
#38751=CARTESIAN_POINT('Ctrl Pts',(4.31392987972073,5.,75.7162200084309));
#38752=CARTESIAN_POINT('Ctrl Pts',(4.35202333876694,-5.,75.7178735790926));
#38753=CARTESIAN_POINT('Ctrl Pts',(4.35202333876694,5.,75.7178735790926));
#38754=CARTESIAN_POINT('Ctrl Pts',(4.38931316854928,-5.,75.7201873093206));
#38755=CARTESIAN_POINT('Ctrl Pts',(4.38931316854928,5.,75.7201873093206));
#38756=CARTESIAN_POINT('Ctrl Pts',(4.4258342922605,-5.,75.7231814575618));
#38757=CARTESIAN_POINT('Ctrl Pts',(4.4258342922605,5.,75.7231814575618));
#38758=CARTESIAN_POINT('Ctrl Pts',(4.46162197741249,-5.,75.7268767771899));
#38759=CARTESIAN_POINT('Ctrl Pts',(4.46162197741249,5.,75.7268767771899));
#38760=CARTESIAN_POINT('Ctrl Pts',(4.49667595482926,-5.,75.7312821851802));
#38761=CARTESIAN_POINT('Ctrl Pts',(4.49667595482926,5.,75.7312821851802));
#38762=CARTESIAN_POINT('Ctrl Pts',(4.53092565703999,-5.,75.7363826907893));
#38763=CARTESIAN_POINT('Ctrl Pts',(4.53092565703999,5.,75.7363826907893));
#38764=CARTESIAN_POINT('Ctrl Pts',(4.56418853184706,-5.,75.7421248073767));
#38765=CARTESIAN_POINT('Ctrl Pts',(4.56418853184706,5.,75.7421248073767));
#38766=CARTESIAN_POINT('Ctrl Pts',(4.59614922798229,-5.,75.7484089314505));
#38767=CARTESIAN_POINT('Ctrl Pts',(4.59614922798229,5.,75.7484089314505));
#38768=CARTESIAN_POINT('Ctrl Pts',(4.62642954792518,-5.,75.7551126455498));
#38769=CARTESIAN_POINT('Ctrl Pts',(4.62642954792518,5.,75.7551126455498));
#38770=CARTESIAN_POINT('Ctrl Pts',(4.6546480607543,-5.,75.7621102084272));
#38771=CARTESIAN_POINT('Ctrl Pts',(4.6546480607543,5.,75.7621102084272));
#38772=CARTESIAN_POINT('Ctrl Pts',(4.68047818546433,-5.,75.7692916356471));
#38773=CARTESIAN_POINT('Ctrl Pts',(4.68047818546433,5.,75.7692916356471));
#38774=CARTESIAN_POINT('Ctrl Pts',(4.70372208056759,-5.,75.7765863103517));
#38775=CARTESIAN_POINT('Ctrl Pts',(4.70372208056759,5.,75.7765863103517));
#38776=CARTESIAN_POINT('Ctrl Pts',(4.72018148924664,-5.,75.7824851942125));
#38777=CARTESIAN_POINT('Ctrl Pts',(4.72018148924664,5.,75.7824851942125));
#38778=CARTESIAN_POINT('Ctrl Pts',(4.73131602214788,-5.,75.7869394346818));
#38779=CARTESIAN_POINT('Ctrl Pts',(4.73131602214788,5.,75.7869394346818));
#38780=CARTESIAN_POINT('Ctrl Pts',(4.73820230448285,-5.,75.7899222948501));
#38781=CARTESIAN_POINT('Ctrl Pts',(4.73820230448285,5.,75.7899222948501));
#38782=CARTESIAN_POINT('Ctrl Pts',(4.7415112563347,-5.,75.7914170652479));
#38783=CARTESIAN_POINT('Ctrl Pts',(4.7415112563347,5.,75.7914170652479));
#38784=CARTESIAN_POINT('',(4.7415112563347,0.,75.7914170652479));
#38785=CARTESIAN_POINT('Ctrl Pts',(3.74291589727827,4.8,75.7622389329459));
#38786=CARTESIAN_POINT('Ctrl Pts',(3.74291589727827,3.13333333333333,75.7622389329459));
#38787=CARTESIAN_POINT('Ctrl Pts',(3.74291589727827,1.46666666666667,75.7622389329459));
#38788=CARTESIAN_POINT('Ctrl Pts',(3.74291589727827,-1.73333333333333,75.7622389329459));
#38789=CARTESIAN_POINT('Ctrl Pts',(3.74291589727829,-3.26666666666667,75.7622389329459));
#38790=CARTESIAN_POINT('Ctrl Pts',(3.74291589727829,-4.8,75.7622389329459));
#38791=CARTESIAN_POINT('Origin',(9.30999999999911,0.,77.9999999999995));
#38792=CARTESIAN_POINT('',(5.49567364700612,0.,75.340410845101));
#38793=CARTESIAN_POINT('',(5.09956505173093,0.,76.0264910574324));
#38794=CARTESIAN_POINT('Origin',(4.7415112563347,0.,75.7914170652479));
#38795=CARTESIAN_POINT('Ctrl Pts',(5.11306670030725,-5.,75.1478641584586));
#38796=CARTESIAN_POINT('Ctrl Pts',(5.11306670030725,5.,75.1478641584586));
#38797=CARTESIAN_POINT('Ctrl Pts',(5.11011771525268,-5.,75.1457459072827));
#38798=CARTESIAN_POINT('Ctrl Pts',(5.11011771525268,5.,75.1457459072827));
#38799=CARTESIAN_POINT('Ctrl Pts',(5.10409134141779,-5.,75.1412736419087));
#38800=CARTESIAN_POINT('Ctrl Pts',(5.10409134141779,5.,75.1412736419087));
#38801=CARTESIAN_POINT('Ctrl Pts',(5.09466658957769,-5.,75.1338579737766));
#38802=CARTESIAN_POINT('Ctrl Pts',(5.09466658957769,5.,75.1338579737766));
#38803=CARTESIAN_POINT('Ctrl Pts',(5.08132830195882,-5.,75.1225531496621));
#38804=CARTESIAN_POINT('Ctrl Pts',(5.08132830195882,5.,75.1225531496621));
#38805=CARTESIAN_POINT('Ctrl Pts',(5.06338898078153,-5.,75.1060706833968));
#38806=CARTESIAN_POINT('Ctrl Pts',(5.06338898078153,5.,75.1060706833968));
#38807=CARTESIAN_POINT('Ctrl Pts',(5.04425461999816,-5.,75.0872918528516));
#38808=CARTESIAN_POINT('Ctrl Pts',(5.04425461999816,5.,75.0872918528516));
#38809=CARTESIAN_POINT('Ctrl Pts',(5.02408529635579,-5.,75.0663526853382));
#38810=CARTESIAN_POINT('Ctrl Pts',(5.02408529635579,5.,75.0663526853382));
#38811=CARTESIAN_POINT('Ctrl Pts',(5.0031395496744,-5.,75.0434810160829));
#38812=CARTESIAN_POINT('Ctrl Pts',(5.0031395496744,5.,75.0434810160829));
#38813=CARTESIAN_POINT('Ctrl Pts',(4.98171699052613,-5.,75.0189443033335));
#38814=CARTESIAN_POINT('Ctrl Pts',(4.98171699052613,5.,75.0189443033335));
#38815=CARTESIAN_POINT('Ctrl Pts',(4.96011273429656,-5.,74.9930088670284));
#38816=CARTESIAN_POINT('Ctrl Pts',(4.96011273429656,5.,74.9930088670284));
#38817=CARTESIAN_POINT('Ctrl Pts',(4.93857071576856,-5.,74.9658980076381));
#38818=CARTESIAN_POINT('Ctrl Pts',(4.93857071576856,5.,74.9658980076381));
#38819=CARTESIAN_POINT('Ctrl Pts',(4.9172285318284,-5.,74.9377430766853));
#38820=CARTESIAN_POINT('Ctrl Pts',(4.9172285318284,5.,74.9377430766853));
#38821=CARTESIAN_POINT('Ctrl Pts',(4.89613444857711,-5.,74.9085976920187));
#38822=CARTESIAN_POINT('Ctrl Pts',(4.89613444857711,5.,74.9085976920187));
#38823=CARTESIAN_POINT('Ctrl Pts',(4.87528087827799,-5.,74.8784665452354));
#38824=CARTESIAN_POINT('Ctrl Pts',(4.87528087827799,5.,74.8784665452354));
#38825=CARTESIAN_POINT('Ctrl Pts',(4.85463221422931,-5.,74.847329470457));
#38826=CARTESIAN_POINT('Ctrl Pts',(4.85463221422931,5.,74.847329470457));
#38827=CARTESIAN_POINT('Ctrl Pts',(4.8341534505069,-5.,74.8151663525323));
#38828=CARTESIAN_POINT('Ctrl Pts',(4.8341534505069,5.,74.8151663525323));
#38829=CARTESIAN_POINT('Ctrl Pts',(4.81384166090143,-5.,74.7819847970791));
#38830=CARTESIAN_POINT('Ctrl Pts',(4.81384166090143,5.,74.7819847970791));
#38831=CARTESIAN_POINT('Ctrl Pts',(4.79372122786737,-5.,74.7478155144698));
#38832=CARTESIAN_POINT('Ctrl Pts',(4.79372122786737,5.,74.7478155144698));
#38833=CARTESIAN_POINT('Ctrl Pts',(4.77383361228174,-5.,74.7127029904203));
#38834=CARTESIAN_POINT('Ctrl Pts',(4.77383361228174,5.,74.7127029904203));
#38835=CARTESIAN_POINT('Ctrl Pts',(4.75422887701992,-5.,74.6766979024307));
#38836=CARTESIAN_POINT('Ctrl Pts',(4.75422887701992,5.,74.6766979024307));
#38837=CARTESIAN_POINT('Ctrl Pts',(4.7349571597282,-5.,74.6398496456652));
#38838=CARTESIAN_POINT('Ctrl Pts',(4.7349571597282,5.,74.6398496456652));
#38839=CARTESIAN_POINT('Ctrl Pts',(4.7160585128285,-5.,74.6021976043606));
#38840=CARTESIAN_POINT('Ctrl Pts',(4.7160585128285,5.,74.6021976043606));
#38841=CARTESIAN_POINT('Ctrl Pts',(4.69756020902596,-5.,74.5637691297098));
#38842=CARTESIAN_POINT('Ctrl Pts',(4.69756020902596,5.,74.5637691297098));
#38843=CARTESIAN_POINT('Ctrl Pts',(4.67948013519603,-5.,74.5245830312156));
#38844=CARTESIAN_POINT('Ctrl Pts',(4.67948013519603,5.,74.5245830312156));
#38845=CARTESIAN_POINT('Ctrl Pts',(4.66182827725193,-5.,74.4846515525847));
#38846=CARTESIAN_POINT('Ctrl Pts',(4.66182827725193,5.,74.4846515525847));
#38847=CARTESIAN_POINT('Ctrl Pts',(4.64460884258076,-5.,74.4439831150201));
#38848=CARTESIAN_POINT('Ctrl Pts',(4.64460884258076,5.,74.4439831150201));
#38849=CARTESIAN_POINT('Ctrl Pts',(4.62782195277069,-5.,74.402584786114));
#38850=CARTESIAN_POINT('Ctrl Pts',(4.62782195277069,5.,74.402584786114));
#38851=CARTESIAN_POINT('Ctrl Pts',(4.611465426047,-5.,74.3604652161898));
#38852=CARTESIAN_POINT('Ctrl Pts',(4.611465426047,5.,74.3604652161898));
#38853=CARTESIAN_POINT('Ctrl Pts',(4.59553572302984,-5.,74.3176336598508));
#38854=CARTESIAN_POINT('Ctrl Pts',(4.59553572302984,5.,74.3176336598508));
#38855=CARTESIAN_POINT('Ctrl Pts',(4.58002879342221,-5.,74.2740988457063));
#38856=CARTESIAN_POINT('Ctrl Pts',(4.58002879342221,5.,74.2740988457063));
#38857=CARTESIAN_POINT('Ctrl Pts',(4.5679584477719,-5.,74.2387142077601));
#38858=CARTESIAN_POINT('Ctrl Pts',(4.5679584477719,5.,74.2387142077601));
#38859=CARTESIAN_POINT('Ctrl Pts',(4.55909298521491,-5.,74.2118647653393));
#38860=CARTESIAN_POINT('Ctrl Pts',(4.55909298521491,5.,74.2118647653393));
#38861=CARTESIAN_POINT('Ctrl Pts',(4.55326576923269,-5.,74.1938271809836));
#38862=CARTESIAN_POINT('Ctrl Pts',(4.55326576923269,5.,74.1938271809836));
#38863=CARTESIAN_POINT('Ctrl Pts',(4.55037293434634,-5.,74.1847738997673));
#38864=CARTESIAN_POINT('Ctrl Pts',(4.55037293434634,5.,74.1847738997673));
#38865=CARTESIAN_POINT('Ctrl Pts',(4.58850001706627,-4.8,74.2976442754434));
#38866=CARTESIAN_POINT('Ctrl Pts',(4.58850001706627,-3.13333333333333,74.2976442754434));
#38867=CARTESIAN_POINT('Ctrl Pts',(4.58850001706627,-1.46666666666667,74.2976442754434));
#38868=CARTESIAN_POINT('Ctrl Pts',(4.58850001706627,1.73333333333333,74.2976442754434));
#38869=CARTESIAN_POINT('Ctrl Pts',(4.58850001706627,3.26666666666667,74.2976442754434));
#38870=CARTESIAN_POINT('Ctrl Pts',(4.58850001706627,4.8,74.2976442754434));
#38871=CARTESIAN_POINT('',(5.11306670030725,0.,75.1478641584586));
#38872=CARTESIAN_POINT('Origin',(5.49567364700612,0.,75.340410845101));
#38873=CARTESIAN_POINT('Ctrl Pts',(4.7262351906713,-5.,73.9751894239903));
#38874=CARTESIAN_POINT('Ctrl Pts',(4.7262351906713,5.,73.9751894239903));
#38875=CARTESIAN_POINT('Ctrl Pts',(4.73565326772794,-5.,73.9764662244033));
#38876=CARTESIAN_POINT('Ctrl Pts',(4.73565326772794,5.,73.9764662244033));
#38877=CARTESIAN_POINT('Ctrl Pts',(4.75442870611518,-5.,73.9790727181826));
#38878=CARTESIAN_POINT('Ctrl Pts',(4.75442870611518,5.,73.9790727181826));
#38879=CARTESIAN_POINT('Ctrl Pts',(4.78240971662693,-5.,73.9831411376458));
#38880=CARTESIAN_POINT('Ctrl Pts',(4.78240971662693,5.,73.9831411376458));
#38881=CARTESIAN_POINT('Ctrl Pts',(4.81935277595994,-5.,73.9888836296986));
#38882=CARTESIAN_POINT('Ctrl Pts',(4.81935277595994,5.,73.9888836296986));
#38883=CARTESIAN_POINT('Ctrl Pts',(4.86491894851451,-5.,73.9965952330726));
#38884=CARTESIAN_POINT('Ctrl Pts',(4.86491894851451,5.,73.9965952330726));
#38885=CARTESIAN_POINT('Ctrl Pts',(4.90986596114075,-5.,74.0048453064445));
#38886=CARTESIAN_POINT('Ctrl Pts',(4.90986596114075,5.,74.0048453064445));
#38887=CARTESIAN_POINT('Ctrl Pts',(4.95418592117643,-5.,74.0136393542666));
#38888=CARTESIAN_POINT('Ctrl Pts',(4.95418592117643,5.,74.0136393542666));
#38889=CARTESIAN_POINT('Ctrl Pts',(4.99787032923525,-5.,74.0229824691756));
#38890=CARTESIAN_POINT('Ctrl Pts',(4.99787032923525,5.,74.0229824691756));
#38891=CARTESIAN_POINT('Ctrl Pts',(5.04091104528079,-5.,74.0328783019017));
#38892=CARTESIAN_POINT('Ctrl Pts',(5.04091104528079,5.,74.0328783019017));
#38893=CARTESIAN_POINT('Ctrl Pts',(5.08330108798191,-5.,74.0433279599757));
#38894=CARTESIAN_POINT('Ctrl Pts',(5.08330108798191,5.,74.0433279599757));
#38895=CARTESIAN_POINT('Ctrl Pts',(5.12503143346602,-5.,74.0543287622593));
#38896=CARTESIAN_POINT('Ctrl Pts',(5.12503143346602,5.,74.0543287622593));
#38897=CARTESIAN_POINT('Ctrl Pts',(5.16608828999564,-5.,74.0658730006512));
#38898=CARTESIAN_POINT('Ctrl Pts',(5.16608828999564,5.,74.0658730006512));
#38899=CARTESIAN_POINT('Ctrl Pts',(5.20645002779749,-5.,74.077946326262));
#38900=CARTESIAN_POINT('Ctrl Pts',(5.20645002779749,5.,74.077946326262));
#38901=CARTESIAN_POINT('Ctrl Pts',(5.24608497534436,-5.,74.0905266302121));
#38902=CARTESIAN_POINT('Ctrl Pts',(5.24608497534436,5.,74.0905266302121));
#38903=CARTESIAN_POINT('Ctrl Pts',(5.28494739170145,-5.,74.1035813075707));
#38904=CARTESIAN_POINT('Ctrl Pts',(5.28494739170145,5.,74.1035813075707));
#38905=CARTESIAN_POINT('Ctrl Pts',(5.32297992581768,-5.,74.1170695597742));
#38906=CARTESIAN_POINT('Ctrl Pts',(5.32297992581768,5.,74.1170695597742));
#38907=CARTESIAN_POINT('Ctrl Pts',(5.36012397677248,-5.,74.1309508845677));
#38908=CARTESIAN_POINT('Ctrl Pts',(5.36012397677248,5.,74.1309508845677));
#38909=CARTESIAN_POINT('Ctrl Pts',(5.39632853508533,-5.,74.145192175818));
#38910=CARTESIAN_POINT('Ctrl Pts',(5.39632853508533,5.,74.145192175818));
#38911=CARTESIAN_POINT('Ctrl Pts',(5.43155912297689,-5.,74.1597747542928));
#38912=CARTESIAN_POINT('Ctrl Pts',(5.43155912297689,5.,74.1597747542928));
#38913=CARTESIAN_POINT('Ctrl Pts',(5.46580875850843,-5.,74.1747028224456));
#38914=CARTESIAN_POINT('Ctrl Pts',(5.46580875850843,5.,74.1747028224456));
#38915=CARTESIAN_POINT('Ctrl Pts',(5.49910332995037,-5.,74.1900073614232));
#38916=CARTESIAN_POINT('Ctrl Pts',(5.49910332995037,5.,74.1900073614232));
#38917=CARTESIAN_POINT('Ctrl Pts',(5.53146887985283,-5.,74.2057199352147));
#38918=CARTESIAN_POINT('Ctrl Pts',(5.53146887985283,5.,74.2057199352147));
#38919=CARTESIAN_POINT('Ctrl Pts',(5.5629021054891,-5.,74.2218488309718));
#38920=CARTESIAN_POINT('Ctrl Pts',(5.5629021054891,5.,74.2218488309718));
#38921=CARTESIAN_POINT('Ctrl Pts',(5.59334182226426,-5.,74.2383558265072));
#38922=CARTESIAN_POINT('Ctrl Pts',(5.59334182226426,5.,74.2383558265072));
#38923=CARTESIAN_POINT('Ctrl Pts',(5.6226347807329,-5.,74.2551282242929));
#38924=CARTESIAN_POINT('Ctrl Pts',(5.6226347807329,5.,74.2551282242929));
#38925=CARTESIAN_POINT('Ctrl Pts',(5.65051871403349,-5.,74.2719645711806));
#38926=CARTESIAN_POINT('Ctrl Pts',(5.65051871403349,5.,74.2719645711806));
#38927=CARTESIAN_POINT('Ctrl Pts',(5.67668010198173,-5.,74.2886204812191));
#38928=CARTESIAN_POINT('Ctrl Pts',(5.67668010198173,5.,74.2886204812191));
#38929=CARTESIAN_POINT('Ctrl Pts',(5.70080352279343,-5.,74.3048473392295));
#38930=CARTESIAN_POINT('Ctrl Pts',(5.70080352279343,5.,74.3048473392295));
#38931=CARTESIAN_POINT('Ctrl Pts',(5.72261970760114,-5.,74.3204300963653));
#38932=CARTESIAN_POINT('Ctrl Pts',(5.72261970760114,5.,74.3204300963653));
#38933=CARTESIAN_POINT('Ctrl Pts',(5.74196689861132,-5.,74.335234728705));
#38934=CARTESIAN_POINT('Ctrl Pts',(5.74196689861132,5.,74.335234728705));
#38935=CARTESIAN_POINT('Ctrl Pts',(5.75541614638509,-5.,74.3464073156572));
#38936=CARTESIAN_POINT('Ctrl Pts',(5.75541614638509,5.,74.3464073156572));
#38937=CARTESIAN_POINT('Ctrl Pts',(5.76435574482978,-5.,74.3544011670878));
#38938=CARTESIAN_POINT('Ctrl Pts',(5.76435574482978,5.,74.3544011670878));
#38939=CARTESIAN_POINT('Ctrl Pts',(5.7698065352688,-5.,74.3595593860371));
#38940=CARTESIAN_POINT('Ctrl Pts',(5.7698065352688,5.,74.3595593860371));
#38941=CARTESIAN_POINT('Ctrl Pts',(5.77240469132477,-5.,74.3620957389297));
#38942=CARTESIAN_POINT('Ctrl Pts',(5.77240469132477,5.,74.3620957389297));
#38943=CARTESIAN_POINT('',(5.77240469132477,0.,74.3620957389297));
#38944=CARTESIAN_POINT('Ctrl Pts',(4.84401151027683,4.8,73.9931375354699));
#38945=CARTESIAN_POINT('Ctrl Pts',(4.84401151027683,3.13333333333333,73.9931375354699));
#38946=CARTESIAN_POINT('Ctrl Pts',(4.84401151027683,1.46666666666667,73.9931375354699));
#38947=CARTESIAN_POINT('Ctrl Pts',(4.84401151027683,-1.73333333333333,73.9931375354699));
#38948=CARTESIAN_POINT('Ctrl Pts',(4.84401151027683,-3.26666666666667,73.9931375354699));
#38949=CARTESIAN_POINT('Ctrl Pts',(4.84401151027683,-4.8,73.9931375354699));
#38950=CARTESIAN_POINT('Origin',(9.30999999999964,0.,77.9999999999996));
#38951=CARTESIAN_POINT('',(6.63533873676838,0.,74.1962272508773));
#38952=CARTESIAN_POINT('',(6.02846516020394,0.,74.7054546451438));
#38953=CARTESIAN_POINT('Origin',(5.77240469132477,0.,74.3620957389297));
#38954=CARTESIAN_POINT('Ctrl Pts',(6.34166065765632,-5.,73.8844332675354));
#38955=CARTESIAN_POINT('Ctrl Pts',(6.34166065765632,5.,73.8844332675354));
#38956=CARTESIAN_POINT('Ctrl Pts',(6.33961400273085,-5.,73.8814341502491));
#38957=CARTESIAN_POINT('Ctrl Pts',(6.33961400273085,5.,73.8814341502491));
#38958=CARTESIAN_POINT('Ctrl Pts',(6.33548066854957,-5.,73.8751704542422));
#38959=CARTESIAN_POINT('Ctrl Pts',(6.33548066854957,5.,73.8751704542422));
#38960=CARTESIAN_POINT('Ctrl Pts',(6.32916060666778,-5.,73.8649785506499));
#38961=CARTESIAN_POINT('Ctrl Pts',(6.32916060666778,5.,73.8649785506499));
#38962=CARTESIAN_POINT('Ctrl Pts',(6.32049319378265,-5.,73.8497935278061));
#38963=CARTESIAN_POINT('Ctrl Pts',(6.32049319378265,5.,73.8497935278061));
#38964=CARTESIAN_POINT('Ctrl Pts',(6.30927308152859,-5.,73.8281694666761));
#38965=CARTESIAN_POINT('Ctrl Pts',(6.30927308152859,5.,73.8281694666761));
#38966=CARTESIAN_POINT('Ctrl Pts',(6.2977154022156,-5.,73.8039788013597));
#38967=CARTESIAN_POINT('Ctrl Pts',(6.2977154022156,5.,73.8039788013597));
#38968=CARTESIAN_POINT('Ctrl Pts',(6.28592405469892,-5.,73.7774041051942));
#38969=CARTESIAN_POINT('Ctrl Pts',(6.28592405469892,5.,73.7774041051942));
#38970=CARTESIAN_POINT('Ctrl Pts',(6.27406406270235,-5.,73.7487478990875));
#38971=CARTESIAN_POINT('Ctrl Pts',(6.27406406270235,5.,73.7487478990875));
#38972=CARTESIAN_POINT('Ctrl Pts',(6.26232549196199,-5.,73.7183639844318));
#38973=CARTESIAN_POINT('Ctrl Pts',(6.26232549196199,5.,73.7183639844318));
#38974=CARTESIAN_POINT('Ctrl Pts',(6.2508945734459,-5.,73.6866035555112));
#38975=CARTESIAN_POINT('Ctrl Pts',(6.2508945734459,5.,73.6866035555112));
#38976=CARTESIAN_POINT('Ctrl Pts',(6.23992415761167,-5.,73.6537598767373));
#38977=CARTESIAN_POINT('Ctrl Pts',(6.23992415761167,5.,73.6537598767373));
#38978=CARTESIAN_POINT('Ctrl Pts',(6.22949861837158,-5.,73.6200034390727));
#38979=CARTESIAN_POINT('Ctrl Pts',(6.22949861837158,5.,73.6200034390727));
#38980=CARTESIAN_POINT('Ctrl Pts',(6.21964497263984,-5.,73.5854011347937));
#38981=CARTESIAN_POINT('Ctrl Pts',(6.21964497263984,5.,73.5854011347937));
#38982=CARTESIAN_POINT('Ctrl Pts',(6.21035448565475,-5.,73.5499547774018));
#38983=CARTESIAN_POINT('Ctrl Pts',(6.21035448565475,5.,73.5499547774018));
#38984=CARTESIAN_POINT('Ctrl Pts',(6.20160059519737,-5.,73.5136332389612));
#38985=CARTESIAN_POINT('Ctrl Pts',(6.20160059519737,5.,73.5136332389612));
#38986=CARTESIAN_POINT('Ctrl Pts',(6.19335728624555,-5.,73.4764056446824));
#38987=CARTESIAN_POINT('Ctrl Pts',(6.19335728624555,5.,73.4764056446824));
#38988=CARTESIAN_POINT('Ctrl Pts',(6.18561920778822,-5.,73.4382781406853));
#38989=CARTESIAN_POINT('Ctrl Pts',(6.18561920778822,5.,73.4382781406853));
#38990=CARTESIAN_POINT('Ctrl Pts',(6.17839876827287,-5.,73.3992879245705));
#38991=CARTESIAN_POINT('Ctrl Pts',(6.17839876827287,5.,73.3992879245705));
#38992=CARTESIAN_POINT('Ctrl Pts',(6.17171971316999,-5.,73.3594909796912));
#38993=CARTESIAN_POINT('Ctrl Pts',(6.17171971316999,5.,73.3594909796912));
#38994=CARTESIAN_POINT('Ctrl Pts',(6.16561175346892,-5.,73.3189520498319));
#38995=CARTESIAN_POINT('Ctrl Pts',(6.16561175346892,5.,73.3189520498319));
#38996=CARTESIAN_POINT('Ctrl Pts',(6.16010510900493,-5.,73.2777346993489));
#38997=CARTESIAN_POINT('Ctrl Pts',(6.16010510900493,5.,73.2777346993489));
#38998=CARTESIAN_POINT('Ctrl Pts',(6.15522394653979,-5.,73.235889636054));
#38999=CARTESIAN_POINT('Ctrl Pts',(6.15522394653979,5.,73.235889636054));
#39000=CARTESIAN_POINT('Ctrl Pts',(6.15098453937228,-5.,73.1934518894766));
#39001=CARTESIAN_POINT('Ctrl Pts',(6.15098453937228,5.,73.1934518894766));
#39002=CARTESIAN_POINT('Ctrl Pts',(6.14739726243605,-5.,73.1504452524406));
#39003=CARTESIAN_POINT('Ctrl Pts',(6.14739726243605,5.,73.1504452524406));
#39004=CARTESIAN_POINT('Ctrl Pts',(6.14446731182389,-5.,73.1068846456515));
#39005=CARTESIAN_POINT('Ctrl Pts',(6.14446731182389,5.,73.1068846456515));
#39006=CARTESIAN_POINT('Ctrl Pts',(6.14219576096471,-5.,73.0627794214626));
#39007=CARTESIAN_POINT('Ctrl Pts',(6.14219576096471,5.,73.0627794214626));
#39008=CARTESIAN_POINT('Ctrl Pts',(6.14058030685598,-5.,73.0181362628236));
#39009=CARTESIAN_POINT('Ctrl Pts',(6.14058030685598,5.,73.0181362628236));
#39010=CARTESIAN_POINT('Ctrl Pts',(6.13961594071856,-5.,72.9729625521674));
#39011=CARTESIAN_POINT('Ctrl Pts',(6.13961594071856,5.,72.9729625521674));
#39012=CARTESIAN_POINT('Ctrl Pts',(6.13929617136756,-5.,72.927265775435));
#39013=CARTESIAN_POINT('Ctrl Pts',(6.13929617136756,5.,72.927265775435));
#39014=CARTESIAN_POINT('Ctrl Pts',(6.13961420741408,-5.,72.8810527495506));
#39015=CARTESIAN_POINT('Ctrl Pts',(6.13961420741408,5.,72.8810527495506));
#39016=CARTESIAN_POINT('Ctrl Pts',(6.14037405162642,-5.,72.8436737650304));
#39017=CARTESIAN_POINT('Ctrl Pts',(6.14037405162642,5.,72.8436737650304));
#39018=CARTESIAN_POINT('Ctrl Pts',(6.14122629204115,-5.,72.815411375335));
#39019=CARTESIAN_POINT('Ctrl Pts',(6.14122629204115,5.,72.815411375335));
#39020=CARTESIAN_POINT('Ctrl Pts',(6.14191971738286,-5.,72.7964685651683));
#39021=CARTESIAN_POINT('Ctrl Pts',(6.14191971738286,5.,72.7964685651683));
#39022=CARTESIAN_POINT('Ctrl Pts',(6.14229774633381,-5.,72.7869718558099));
#39023=CARTESIAN_POINT('Ctrl Pts',(6.14229774633381,5.,72.7869718558099));
#39024=CARTESIAN_POINT('Ctrl Pts',(6.13952154251132,-4.8,72.9060755452598));
#39025=CARTESIAN_POINT('Ctrl Pts',(6.13952154251132,-3.13333333333333,72.9060755452598));
#39026=CARTESIAN_POINT('Ctrl Pts',(6.13952154251132,-1.46666666666667,72.9060755452598));
#39027=CARTESIAN_POINT('Ctrl Pts',(6.13952154251132,1.73333333333333,72.9060755452598));
#39028=CARTESIAN_POINT('Ctrl Pts',(6.13952154251132,3.26666666666667,72.9060755452598));
#39029=CARTESIAN_POINT('Ctrl Pts',(6.13952154251132,4.8,72.9060755452598));
#39030=CARTESIAN_POINT('',(6.34166065765632,0.,73.8844332675354));
#39031=CARTESIAN_POINT('Origin',(6.63533873676838,0.,74.1962272508773));
#39032=CARTESIAN_POINT('Ctrl Pts',(8.38573080884383,-5.,71.9704289984876));
#39033=CARTESIAN_POINT('Ctrl Pts',(8.38573080884383,5.,71.9704289984876));
#39034=CARTESIAN_POINT('Ctrl Pts',(8.39212476293556,-5.,71.9774609075814));
#39035=CARTESIAN_POINT('Ctrl Pts',(8.39212476293556,5.,71.9774609075814));
#39036=CARTESIAN_POINT('Ctrl Pts',(8.40483216124376,-5.,71.991526216807));
#39037=CARTESIAN_POINT('Ctrl Pts',(8.40483216124376,5.,71.991526216807));
#39038=CARTESIAN_POINT('Ctrl Pts',(8.42365172920544,-5.,72.0126286537798));
#39039=CARTESIAN_POINT('Ctrl Pts',(8.42365172920544,5.,72.0126286537798));
#39040=CARTESIAN_POINT('Ctrl Pts',(8.44826055176072,-5.,72.040774198702));
#39041=CARTESIAN_POINT('Ctrl Pts',(8.44826055176072,5.,72.040774198702));
#39042=CARTESIAN_POINT('Ctrl Pts',(8.47820934194863,-5.,72.0759710007559));
#39043=CARTESIAN_POINT('Ctrl Pts',(8.47820934194863,5.,72.0759710007559));
#39044=CARTESIAN_POINT('Ctrl Pts',(8.5073377062906,-5.,72.1111823064372));
#39045=CARTESIAN_POINT('Ctrl Pts',(8.5073377062906,5.,72.1111823064372));
#39046=CARTESIAN_POINT('Ctrl Pts',(8.5356360604508,-5.,72.1464072590907));
#39047=CARTESIAN_POINT('Ctrl Pts',(8.5356360604508,5.,72.1464072590907));
#39048=CARTESIAN_POINT('Ctrl Pts',(8.56309462002684,-5.,72.1816442965978));
#39049=CARTESIAN_POINT('Ctrl Pts',(8.56309462002684,5.,72.1816442965978));
#39050=CARTESIAN_POINT('Ctrl Pts',(8.58970480273757,-5.,72.2168909832624));
#39051=CARTESIAN_POINT('Ctrl Pts',(8.58970480273757,5.,72.2168909832624));
#39052=CARTESIAN_POINT('Ctrl Pts',(8.61546054866421,-5.,72.2521436799883));
#39053=CARTESIAN_POINT('Ctrl Pts',(8.61546054866421,5.,72.2521436799883));
#39054=CARTESIAN_POINT('Ctrl Pts',(8.6403566685235,-5.,72.2873945324713));
#39055=CARTESIAN_POINT('Ctrl Pts',(8.6403566685235,5.,72.2873945324713));
#39056=CARTESIAN_POINT('Ctrl Pts',(8.66438755190754,-5.,72.322628770807));
#39057=CARTESIAN_POINT('Ctrl Pts',(8.66438755190754,5.,72.322628770807));
#39058=CARTESIAN_POINT('Ctrl Pts',(8.68754585274241,-5.,72.3578214997599));
#39059=CARTESIAN_POINT('Ctrl Pts',(8.68754585274241,5.,72.3578214997599));
#39060=CARTESIAN_POINT('Ctrl Pts',(8.7098215205491,-5.,72.3929354248824));
#39061=CARTESIAN_POINT('Ctrl Pts',(8.7098215205491,5.,72.3929354248824));
#39062=CARTESIAN_POINT('Ctrl Pts',(8.73120047378673,-5.,72.4279161676434));
#39063=CARTESIAN_POINT('Ctrl Pts',(8.73120047378673,5.,72.4279161676434));
#39064=CARTESIAN_POINT('Ctrl Pts',(8.75166500381177,-5.,72.4626956099856));
#39065=CARTESIAN_POINT('Ctrl Pts',(8.75166500381177,5.,72.4626956099856));
#39066=CARTESIAN_POINT('Ctrl Pts',(8.77119625406051,-5.,72.4972050574356));
#39067=CARTESIAN_POINT('Ctrl Pts',(8.77119625406051,5.,72.4972050574356));
#39068=CARTESIAN_POINT('Ctrl Pts',(8.78977642921376,-5.,72.5313863609611));
#39069=CARTESIAN_POINT('Ctrl Pts',(8.78977642921376,5.,72.5313863609611));
#39070=CARTESIAN_POINT('Ctrl Pts',(8.80739112453777,-5.,72.5652030495491));
#39071=CARTESIAN_POINT('Ctrl Pts',(8.80739112453777,5.,72.5652030495491));
#39072=CARTESIAN_POINT('Ctrl Pts',(8.82403229027104,-5.,72.5986538545611));
#39073=CARTESIAN_POINT('Ctrl Pts',(8.82403229027104,5.,72.5986538545611));
#39074=CARTESIAN_POINT('Ctrl Pts',(8.83969984368247,-5.,72.6317791495918));
#39075=CARTESIAN_POINT('Ctrl Pts',(8.83969984368247,5.,72.6317791495918));
#39076=CARTESIAN_POINT('Ctrl Pts',(8.85439344558271,-5.,72.6646198538891));
#39077=CARTESIAN_POINT('Ctrl Pts',(8.85439344558271,5.,72.6646198538891));
#39078=CARTESIAN_POINT('Ctrl Pts',(8.86810523905958,-5.,72.697180192828));
#39079=CARTESIAN_POINT('Ctrl Pts',(8.86810523905958,5.,72.697180192828));
#39080=CARTESIAN_POINT('Ctrl Pts',(8.88081292274355,-5.,72.7293915578161));
#39081=CARTESIAN_POINT('Ctrl Pts',(8.88081292274355,5.,72.7293915578161));
#39082=CARTESIAN_POINT('Ctrl Pts',(8.892471541323,-5.,72.7610691106936));
#39083=CARTESIAN_POINT('Ctrl Pts',(8.892471541323,5.,72.7610691106936));
#39084=CARTESIAN_POINT('Ctrl Pts',(8.90300967831155,-5.,72.7918899475057));
#39085=CARTESIAN_POINT('Ctrl Pts',(8.90300967831155,5.,72.7918899475057));
#39086=CARTESIAN_POINT('Ctrl Pts',(8.91234425157306,-5.,72.8214653308615));
#39087=CARTESIAN_POINT('Ctrl Pts',(8.91234425157306,5.,72.8214653308615));
#39088=CARTESIAN_POINT('Ctrl Pts',(8.92039344075756,-5.,72.8494020612689));
#39089=CARTESIAN_POINT('Ctrl Pts',(8.92039344075756,5.,72.8494020612689));
#39090=CARTESIAN_POINT('Ctrl Pts',(8.92708920468011,-5.,72.875362319063));
#39091=CARTESIAN_POINT('Ctrl Pts',(8.92708920468011,5.,72.875362319063));
#39092=CARTESIAN_POINT('Ctrl Pts',(8.93239377860217,-5.,72.8991394600597));
#39093=CARTESIAN_POINT('Ctrl Pts',(8.93239377860217,5.,72.8991394600597));
#39094=CARTESIAN_POINT('Ctrl Pts',(8.93551489966184,-5.,72.9163431680377));
#39095=CARTESIAN_POINT('Ctrl Pts',(8.93551489966184,5.,72.9163431680377));
#39096=CARTESIAN_POINT('Ctrl Pts',(8.9372246807253,-5.,72.928213076623));
#39097=CARTESIAN_POINT('Ctrl Pts',(8.9372246807253,5.,72.928213076623));
#39098=CARTESIAN_POINT('Ctrl Pts',(8.93808458922835,-5.,72.9356682021451));
#39099=CARTESIAN_POINT('Ctrl Pts',(8.93808458922835,5.,72.9356682021451));
#39100=CARTESIAN_POINT('Ctrl Pts',(8.93844455602745,-5.,72.9392812237066));
#39101=CARTESIAN_POINT('Ctrl Pts',(8.93844455602745,5.,72.9392812237066));
#39102=CARTESIAN_POINT('',(8.93844455602745,0.,72.9392812237066));
#39103=CARTESIAN_POINT('Ctrl Pts',(8.46441588028027,4.8,72.0598832085154));
#39104=CARTESIAN_POINT('Ctrl Pts',(8.46441588028027,3.13333333333333,72.0598832085154));
#39105=CARTESIAN_POINT('Ctrl Pts',(8.46441588028027,1.46666666666667,72.0598832085154));
#39106=CARTESIAN_POINT('Ctrl Pts',(8.46441588028027,-1.73333333333333,72.0598832085154));
#39107=CARTESIAN_POINT('Ctrl Pts',(8.46441588028027,-3.26666666666667,72.0598832085153));
#39108=CARTESIAN_POINT('Ctrl Pts',(8.46441588028027,-4.8,72.0598832085153));
#39109=CARTESIAN_POINT('Origin',(9.31,0.,77.9999999999998));
#39110=CARTESIAN_POINT('',(9.70610859527519,0.,73.3669019025333));
#39111=CARTESIAN_POINT('',(8.91389140472481,0.,73.3669019025333));
#39112=CARTESIAN_POINT('Origin',(8.93844455602745,0.,72.9392812237066));
#39113=CARTESIAN_POINT('Ctrl Pts',(9.68155544397255,-5.,72.9392812237066));
#39114=CARTESIAN_POINT('Ctrl Pts',(9.68155544397255,5.,72.9392812237066));
#39115=CARTESIAN_POINT('Ctrl Pts',(9.6819154107701,-5.,72.9356682021447));
#39116=CARTESIAN_POINT('Ctrl Pts',(9.6819154107701,5.,72.9356682021447));
#39117=CARTESIAN_POINT('Ctrl Pts',(9.68277531927063,-5.,72.9282130766218));
#39118=CARTESIAN_POINT('Ctrl Pts',(9.68277531927063,5.,72.9282130766218));
#39119=CARTESIAN_POINT('Ctrl Pts',(9.68448510033203,-5.,72.9163431680359));
#39120=CARTESIAN_POINT('Ctrl Pts',(9.68448510033203,5.,72.9163431680359));
#39121=CARTESIAN_POINT('Ctrl Pts',(9.68760622139204,-5.,72.8991394600578));
#39122=CARTESIAN_POINT('Ctrl Pts',(9.68760622139204,5.,72.8991394600578));
#39123=CARTESIAN_POINT('Ctrl Pts',(9.69291079531749,-5.,72.875362319062));
#39124=CARTESIAN_POINT('Ctrl Pts',(9.69291079531749,5.,72.875362319062));
#39125=CARTESIAN_POINT('Ctrl Pts',(9.69960655924369,-5.,72.8494020612693));
#39126=CARTESIAN_POINT('Ctrl Pts',(9.69960655924369,5.,72.8494020612693));
#39127=CARTESIAN_POINT('Ctrl Pts',(9.70765574843018,-5.,72.8214653308631));
#39128=CARTESIAN_POINT('Ctrl Pts',(9.70765574843018,5.,72.8214653308631));
#39129=CARTESIAN_POINT('Ctrl Pts',(9.7169903216916,-5.,72.7918899475077));
#39130=CARTESIAN_POINT('Ctrl Pts',(9.7169903216916,5.,72.7918899475077));
#39131=CARTESIAN_POINT('Ctrl Pts',(9.72752845867869,-5.,72.7610691106953));
#39132=CARTESIAN_POINT('Ctrl Pts',(9.72752845867869,5.,72.7610691106953));
#39133=CARTESIAN_POINT('Ctrl Pts',(9.73918707725648,-5.,72.7293915578165));
#39134=CARTESIAN_POINT('Ctrl Pts',(9.73918707725648,5.,72.7293915578165));
#39135=CARTESIAN_POINT('Ctrl Pts',(9.75189476093958,-5.,72.6971801928267));
#39136=CARTESIAN_POINT('Ctrl Pts',(9.75189476093958,5.,72.6971801928267));
#39137=CARTESIAN_POINT('Ctrl Pts',(9.76560655441652,-5.,72.6646198538862));
#39138=CARTESIAN_POINT('Ctrl Pts',(9.76560655441652,5.,72.6646198538862));
#39139=CARTESIAN_POINT('Ctrl Pts',(9.78030015631738,-5.,72.6317791495885));
#39140=CARTESIAN_POINT('Ctrl Pts',(9.78030015631738,5.,72.6317791495885));
#39141=CARTESIAN_POINT('Ctrl Pts',(9.79596770972936,-5.,72.5986538545587));
#39142=CARTESIAN_POINT('Ctrl Pts',(9.79596770972936,5.,72.5986538545587));
#39143=CARTESIAN_POINT('Ctrl Pts',(9.81260887546254,-5.,72.5652030495487));
#39144=CARTESIAN_POINT('Ctrl Pts',(9.81260887546254,5.,72.5652030495487));
#39145=CARTESIAN_POINT('Ctrl Pts',(9.83022357078552,-5.,72.5313863609631));
#39146=CARTESIAN_POINT('Ctrl Pts',(9.83022357078552,5.,72.5313863609631));
#39147=CARTESIAN_POINT('Ctrl Pts',(9.84880374593723,-5.,72.4972050574394));
#39148=CARTESIAN_POINT('Ctrl Pts',(9.84880374593723,5.,72.4972050574394));
#39149=CARTESIAN_POINT('Ctrl Pts',(9.86833499618467,-5.,72.46269560999));
#39150=CARTESIAN_POINT('Ctrl Pts',(9.86833499618467,5.,72.46269560999));
#39151=CARTESIAN_POINT('Ctrl Pts',(9.88879952620961,-5.,72.4279161676469));
#39152=CARTESIAN_POINT('Ctrl Pts',(9.88879952620961,5.,72.4279161676469));
#39153=CARTESIAN_POINT('Ctrl Pts',(9.91017847944898,-5.,72.3929354248836));
#39154=CARTESIAN_POINT('Ctrl Pts',(9.91017847944898,5.,72.3929354248836));
#39155=CARTESIAN_POINT('Ctrl Pts',(9.9324541472595,-5.,72.3578214997584));
#39156=CARTESIAN_POINT('Ctrl Pts',(9.9324541472595,5.,72.3578214997584));
#39157=CARTESIAN_POINT('Ctrl Pts',(9.95561244809927,-5.,72.322628770803));
#39158=CARTESIAN_POINT('Ctrl Pts',(9.95561244809927,5.,72.322628770803));
#39159=CARTESIAN_POINT('Ctrl Pts',(9.97964333148752,-5.,72.2873945324658));
#39160=CARTESIAN_POINT('Ctrl Pts',(9.97964333148752,5.,72.2873945324658));
#39161=CARTESIAN_POINT('Ctrl Pts',(10.0045394513483,-5.,72.2521436799828));
#39162=CARTESIAN_POINT('Ctrl Pts',(10.0045394513483,5.,72.2521436799828));
#39163=CARTESIAN_POINT('Ctrl Pts',(10.0302951972721,-5.,72.2168909832587));
#39164=CARTESIAN_POINT('Ctrl Pts',(10.0302951972721,5.,72.2168909832587));
#39165=CARTESIAN_POINT('Ctrl Pts',(10.0569053799749,-5.,72.1816442965973));
#39166=CARTESIAN_POINT('Ctrl Pts',(10.0569053799749,5.,72.1816442965973));
#39167=CARTESIAN_POINT('Ctrl Pts',(10.0843639395388,-5.,72.1464072590943));
#39168=CARTESIAN_POINT('Ctrl Pts',(10.0843639395388,5.,72.1464072590943));
#39169=CARTESIAN_POINT('Ctrl Pts',(10.1126622936855,-5.,72.1111823064446));
#39170=CARTESIAN_POINT('Ctrl Pts',(10.1126622936855,5.,72.1111823064446));
#39171=CARTESIAN_POINT('Ctrl Pts',(10.1417906580168,-5.,72.0759710007657));
#39172=CARTESIAN_POINT('Ctrl Pts',(10.1417906580168,5.,72.0759710007657));
#39173=CARTESIAN_POINT('Ctrl Pts',(10.1717394482016,-5.,72.0407741987119));
#39174=CARTESIAN_POINT('Ctrl Pts',(10.1717394482016,5.,72.0407741987119));
#39175=CARTESIAN_POINT('Ctrl Pts',(10.1963482707641,-5.,72.0126286537873));
#39176=CARTESIAN_POINT('Ctrl Pts',(10.1963482707641,5.,72.0126286537873));
#39177=CARTESIAN_POINT('Ctrl Pts',(10.2151678387382,-5.,71.9915262168113));
#39178=CARTESIAN_POINT('Ctrl Pts',(10.2151678387382,5.,71.9915262168113));
#39179=CARTESIAN_POINT('Ctrl Pts',(10.2278752370579,-5.,71.9774609075829));
#39180=CARTESIAN_POINT('Ctrl Pts',(10.2278752370579,5.,71.9774609075829));
#39181=CARTESIAN_POINT('Ctrl Pts',(10.2342691911562,-5.,71.9704289984876));
#39182=CARTESIAN_POINT('Ctrl Pts',(10.2342691911562,5.,71.9704289984876));
#39183=CARTESIAN_POINT('Ctrl Pts',(10.1555841196958,-4.8,72.059883208512));
#39184=CARTESIAN_POINT('Ctrl Pts',(10.1555841196958,-3.13333333333333,72.059883208512));
#39185=CARTESIAN_POINT('Ctrl Pts',(10.1555841196958,-1.46666666666667,72.059883208512));
#39186=CARTESIAN_POINT('Ctrl Pts',(10.1555841196958,1.73333333333333,72.059883208512));
#39187=CARTESIAN_POINT('Ctrl Pts',(10.1555841196958,3.26666666666667,72.059883208512));
#39188=CARTESIAN_POINT('Ctrl Pts',(10.1555841196958,4.8,72.059883208512));
#39189=CARTESIAN_POINT('',(9.68155544397255,0.,72.9392812237066));
#39190=CARTESIAN_POINT('Origin',(9.70610859527519,0.,73.3669019025333));
#39191=CARTESIAN_POINT('Ctrl Pts',(12.4777022536662,-5.,72.7869718558099));
#39192=CARTESIAN_POINT('Ctrl Pts',(12.4777022536662,5.,72.7869718558099));
#39193=CARTESIAN_POINT('Ctrl Pts',(12.4780802826126,-5.,72.7964685651569));
#39194=CARTESIAN_POINT('Ctrl Pts',(12.4780802826126,5.,72.7964685651569));
#39195=CARTESIAN_POINT('Ctrl Pts',(12.4787737079463,-5.,72.8154113753035));
#39196=CARTESIAN_POINT('Ctrl Pts',(12.4787737079463,5.,72.8154113753035));
#39197=CARTESIAN_POINT('Ctrl Pts',(12.4796259483525,-5.,72.8436737649773));
#39198=CARTESIAN_POINT('Ctrl Pts',(12.4796259483525,5.,72.8436737649773));
#39199=CARTESIAN_POINT('Ctrl Pts',(12.4803857925599,-5.,72.8810527494849));
#39200=CARTESIAN_POINT('Ctrl Pts',(12.4803857925599,5.,72.8810527494849));
#39201=CARTESIAN_POINT('Ctrl Pts',(12.4807038286085,-5.,72.9272657753747));
#39202=CARTESIAN_POINT('Ctrl Pts',(12.4807038286085,5.,72.9272657753747));
#39203=CARTESIAN_POINT('Ctrl Pts',(12.4803840592649,-5.,72.9729625521258));
#39204=CARTESIAN_POINT('Ctrl Pts',(12.4803840592649,5.,72.9729625521258));
#39205=CARTESIAN_POINT('Ctrl Pts',(12.4794196931369,-5.,73.0181362628057));
#39206=CARTESIAN_POINT('Ctrl Pts',(12.4794196931369,5.,73.0181362628057));
#39207=CARTESIAN_POINT('Ctrl Pts',(12.4778042390365,-5.,73.0627794214657));
#39208=CARTESIAN_POINT('Ctrl Pts',(12.4778042390365,5.,73.0627794214657));
#39209=CARTESIAN_POINT('Ctrl Pts',(12.4755326881828,-5.,73.106884645668));
#39210=CARTESIAN_POINT('Ctrl Pts',(12.4755326881828,5.,73.106884645668));
#39211=CARTESIAN_POINT('Ctrl Pts',(12.4726027375726,-5.,73.1504452524619));
#39212=CARTESIAN_POINT('Ctrl Pts',(12.4726027375726,5.,73.1504452524619));
#39213=CARTESIAN_POINT('Ctrl Pts',(12.4690154606353,-5.,73.1934518894953));
#39214=CARTESIAN_POINT('Ctrl Pts',(12.4690154606353,5.,73.1934518894953));
#39215=CARTESIAN_POINT('Ctrl Pts',(12.4647760534649,-5.,73.2358896360656));
#39216=CARTESIAN_POINT('Ctrl Pts',(12.4647760534649,5.,73.2358896360656));
#39217=CARTESIAN_POINT('Ctrl Pts',(12.4598948909964,-5.,73.2777346993523));
#39218=CARTESIAN_POINT('Ctrl Pts',(12.4598948909964,5.,73.2777346993523));
#39219=CARTESIAN_POINT('Ctrl Pts',(12.4543882465297,-5.,73.3189520498286));
#39220=CARTESIAN_POINT('Ctrl Pts',(12.4543882465297,5.,73.3189520498286));
#39221=CARTESIAN_POINT('Ctrl Pts',(12.4482802868274,-5.,73.3594909796843));
#39222=CARTESIAN_POINT('Ctrl Pts',(12.4482802868274,5.,73.3594909796843));
#39223=CARTESIAN_POINT('Ctrl Pts',(12.4416012317246,-5.,73.3992879245629));
#39224=CARTESIAN_POINT('Ctrl Pts',(12.4416012317246,5.,73.3992879245629));
#39225=CARTESIAN_POINT('Ctrl Pts',(12.4343807922101,-5.,73.4382781406794));
#39226=CARTESIAN_POINT('Ctrl Pts',(12.4343807922101,5.,73.4382781406794));
#39227=CARTESIAN_POINT('Ctrl Pts',(12.4266427137538,-5.,73.4764056446796));
#39228=CARTESIAN_POINT('Ctrl Pts',(12.4266427137538,5.,73.4764056446796));
#39229=CARTESIAN_POINT('Ctrl Pts',(12.4183994048028,-5.,73.5136332389618));
#39230=CARTESIAN_POINT('Ctrl Pts',(12.4183994048028,5.,73.5136332389618));
#39231=CARTESIAN_POINT('Ctrl Pts',(12.4096455143457,-5.,73.5499547774051));
#39232=CARTESIAN_POINT('Ctrl Pts',(12.4096455143457,5.,73.5499547774051));
#39233=CARTESIAN_POINT('Ctrl Pts',(12.4003550273604,-5.,73.5854011347984));
#39234=CARTESIAN_POINT('Ctrl Pts',(12.4003550273604,5.,73.5854011347984));
#39235=CARTESIAN_POINT('Ctrl Pts',(12.3905013816283,-5.,73.6200034390768));
#39236=CARTESIAN_POINT('Ctrl Pts',(12.3905013816283,5.,73.6200034390768));
#39237=CARTESIAN_POINT('Ctrl Pts',(12.380075842388,-5.,73.6537598767393));
#39238=CARTESIAN_POINT('Ctrl Pts',(12.380075842388,5.,73.6537598767393));
#39239=CARTESIAN_POINT('Ctrl Pts',(12.3691054265541,-5.,73.6866035555106));
#39240=CARTESIAN_POINT('Ctrl Pts',(12.3691054265541,5.,73.6866035555106));
#39241=CARTESIAN_POINT('Ctrl Pts',(12.3576745080387,-5.,73.7183639844293));
#39242=CARTESIAN_POINT('Ctrl Pts',(12.3576745080387,5.,73.7183639844293));
#39243=CARTESIAN_POINT('Ctrl Pts',(12.3459359372991,-5.,73.7487478990847));
#39244=CARTESIAN_POINT('Ctrl Pts',(12.3459359372991,5.,73.7487478990847));
#39245=CARTESIAN_POINT('Ctrl Pts',(12.3340759453026,-5.,73.7774041051921));
#39246=CARTESIAN_POINT('Ctrl Pts',(12.3340759453026,5.,73.7774041051921));
#39247=CARTESIAN_POINT('Ctrl Pts',(12.322284597785,-5.,73.8039788013593));
#39248=CARTESIAN_POINT('Ctrl Pts',(12.322284597785,5.,73.8039788013593));
#39249=CARTESIAN_POINT('Ctrl Pts',(12.3107269184702,-5.,73.8281694666772));
#39250=CARTESIAN_POINT('Ctrl Pts',(12.3107269184702,5.,73.8281694666772));
#39251=CARTESIAN_POINT('Ctrl Pts',(12.2995068062144,-5.,73.8497935278081));
#39252=CARTESIAN_POINT('Ctrl Pts',(12.2995068062144,5.,73.8497935278081));
#39253=CARTESIAN_POINT('Ctrl Pts',(12.2908393933291,-5.,73.8649785506518));
#39254=CARTESIAN_POINT('Ctrl Pts',(12.2908393933291,5.,73.8649785506518));
#39255=CARTESIAN_POINT('Ctrl Pts',(12.2845193314483,-5.,73.8751704542434));
#39256=CARTESIAN_POINT('Ctrl Pts',(12.2845193314483,5.,73.8751704542434));
#39257=CARTESIAN_POINT('Ctrl Pts',(12.2803859972684,-5.,73.8814341502495));
#39258=CARTESIAN_POINT('Ctrl Pts',(12.2803859972684,5.,73.8814341502495));
#39259=CARTESIAN_POINT('Ctrl Pts',(12.2783393423437,-5.,73.8844332675354));
#39260=CARTESIAN_POINT('Ctrl Pts',(12.2783393423437,5.,73.8844332675354));
#39261=CARTESIAN_POINT('',(12.2783393423437,0.,73.8844332675354));
#39262=CARTESIAN_POINT('Ctrl Pts',(12.4804784574649,4.8,72.906075545245));
#39263=CARTESIAN_POINT('Ctrl Pts',(12.4804784574649,3.13333333333333,72.906075545245));
#39264=CARTESIAN_POINT('Ctrl Pts',(12.4804784574649,1.46666666666667,72.906075545245));
#39265=CARTESIAN_POINT('Ctrl Pts',(12.4804784574649,-1.73333333333333,72.906075545245));
#39266=CARTESIAN_POINT('Ctrl Pts',(12.4804784574649,-3.26666666666667,72.906075545245));
#39267=CARTESIAN_POINT('Ctrl Pts',(12.4804784574649,-4.8,72.906075545245));
#39268=CARTESIAN_POINT('Origin',(9.3099999999996,0.,78.0000000000005));
#39269=CARTESIAN_POINT('',(12.5915348397961,0.,74.7054546451438));
#39270=CARTESIAN_POINT('',(11.9846612632316,0.,74.1962272508773));
#39271=CARTESIAN_POINT('Origin',(12.2783393423437,0.,73.8844332675354));
#39272=CARTESIAN_POINT('Ctrl Pts',(12.8475953086752,-5.,74.3620957389297));
#39273=CARTESIAN_POINT('Ctrl Pts',(12.8475953086752,5.,74.3620957389297));
#39274=CARTESIAN_POINT('Ctrl Pts',(12.8501934647285,-5.,74.3595593860371));
#39275=CARTESIAN_POINT('Ctrl Pts',(12.8501934647285,5.,74.3595593860371));
#39276=CARTESIAN_POINT('Ctrl Pts',(12.8556442551632,-5.,74.3544011670879));
#39277=CARTESIAN_POINT('Ctrl Pts',(12.8556442551632,5.,74.3544011670879));
#39278=CARTESIAN_POINT('Ctrl Pts',(12.8645838536043,-5.,74.3464073156575));
#39279=CARTESIAN_POINT('Ctrl Pts',(12.8645838536043,5.,74.3464073156575));
#39280=CARTESIAN_POINT('Ctrl Pts',(12.8780331013787,-5.,74.3352347287054));
#39281=CARTESIAN_POINT('Ctrl Pts',(12.8780331013787,5.,74.3352347287054));
#39282=CARTESIAN_POINT('Ctrl Pts',(12.8973802923948,-5.,74.3204300963656));
#39283=CARTESIAN_POINT('Ctrl Pts',(12.8973802923948,5.,74.3204300963656));
#39284=CARTESIAN_POINT('Ctrl Pts',(12.9191964772087,-5.,74.3048473392293));
#39285=CARTESIAN_POINT('Ctrl Pts',(12.9191964772087,5.,74.3048473392293));
#39286=CARTESIAN_POINT('Ctrl Pts',(12.9433198980238,-5.,74.2886204812186));
#39287=CARTESIAN_POINT('Ctrl Pts',(12.9433198980238,5.,74.2886204812186));
#39288=CARTESIAN_POINT('Ctrl Pts',(12.9694812859721,-5.,74.2719645711802));
#39289=CARTESIAN_POINT('Ctrl Pts',(12.9694812859721,5.,74.2719645711802));
#39290=CARTESIAN_POINT('Ctrl Pts',(12.9973652192703,-5.,74.2551282242927));
#39291=CARTESIAN_POINT('Ctrl Pts',(12.9973652192703,5.,74.2551282242927));
#39292=CARTESIAN_POINT('Ctrl Pts',(13.0266581777359,-5.,74.2383558265071));
#39293=CARTESIAN_POINT('Ctrl Pts',(13.0266581777359,5.,74.2383558265071));
#39294=CARTESIAN_POINT('Ctrl Pts',(13.0570978945092,-5.,74.221848830972));
#39295=CARTESIAN_POINT('Ctrl Pts',(13.0570978945092,5.,74.221848830972));
#39296=CARTESIAN_POINT('Ctrl Pts',(13.0885311201451,-5.,74.2057199352152));
#39297=CARTESIAN_POINT('Ctrl Pts',(13.0885311201451,5.,74.2057199352152));
#39298=CARTESIAN_POINT('Ctrl Pts',(13.1208966700483,-5.,74.1900073614239));
#39299=CARTESIAN_POINT('Ctrl Pts',(13.1208966700483,5.,74.1900073614239));
#39300=CARTESIAN_POINT('Ctrl Pts',(13.1541912414913,-5.,74.1747028224464));
#39301=CARTESIAN_POINT('Ctrl Pts',(13.1541912414913,5.,74.1747028224464));
#39302=CARTESIAN_POINT('Ctrl Pts',(13.1884408770234,-5.,74.1597747542931));
#39303=CARTESIAN_POINT('Ctrl Pts',(13.1884408770234,5.,74.1597747542931));
#39304=CARTESIAN_POINT('Ctrl Pts',(13.2236714649144,-5.,74.145192175817));
#39305=CARTESIAN_POINT('Ctrl Pts',(13.2236714649144,5.,74.145192175817));
#39306=CARTESIAN_POINT('Ctrl Pts',(13.259876023226,-5.,74.1309508845651));
#39307=CARTESIAN_POINT('Ctrl Pts',(13.259876023226,5.,74.1309508845651));
#39308=CARTESIAN_POINT('Ctrl Pts',(13.2970200741795,-5.,74.1170695597709));
#39309=CARTESIAN_POINT('Ctrl Pts',(13.2970200741795,5.,74.1170695597709));
#39310=CARTESIAN_POINT('Ctrl Pts',(13.3350526082954,-5.,74.103581307568));
#39311=CARTESIAN_POINT('Ctrl Pts',(13.3350526082954,5.,74.103581307568));
#39312=CARTESIAN_POINT('Ctrl Pts',(13.3739150246539,-5.,74.0905266302112));
#39313=CARTESIAN_POINT('Ctrl Pts',(13.3739150246539,5.,74.0905266302112));
#39314=CARTESIAN_POINT('Ctrl Pts',(13.4135499722042,-5.,74.0779463262631));
#39315=CARTESIAN_POINT('Ctrl Pts',(13.4135499722042,5.,74.0779463262631));
#39316=CARTESIAN_POINT('Ctrl Pts',(13.4539117100106,-5.,74.065873000654));
#39317=CARTESIAN_POINT('Ctrl Pts',(13.4539117100106,5.,74.065873000654));
#39318=CARTESIAN_POINT('Ctrl Pts',(13.4949685665442,-5.,74.0543287622629));
#39319=CARTESIAN_POINT('Ctrl Pts',(13.4949685665442,5.,74.0543287622629));
#39320=CARTESIAN_POINT('Ctrl Pts',(13.5366989120298,-5.,74.0433279599792));
#39321=CARTESIAN_POINT('Ctrl Pts',(13.5366989120298,5.,74.0433279599792));
#39322=CARTESIAN_POINT('Ctrl Pts',(13.5790889547283,-5.,74.0328783019039));
#39323=CARTESIAN_POINT('Ctrl Pts',(13.5790889547283,5.,74.0328783019039));
#39324=CARTESIAN_POINT('Ctrl Pts',(13.6221296707664,-5.,74.0229824691757));
#39325=CARTESIAN_POINT('Ctrl Pts',(13.6221296707664,5.,74.0229824691757));
#39326=CARTESIAN_POINT('Ctrl Pts',(13.6658140788138,-5.,74.0136393542647));
#39327=CARTESIAN_POINT('Ctrl Pts',(13.6658140788138,5.,74.0136393542647));
#39328=CARTESIAN_POINT('Ctrl Pts',(13.7101340388369,-5.,74.0048453064413));
#39329=CARTESIAN_POINT('Ctrl Pts',(13.7101340388369,5.,74.0048453064413));
#39330=CARTESIAN_POINT('Ctrl Pts',(13.7550810514531,-5.,73.9965952330688));
#39331=CARTESIAN_POINT('Ctrl Pts',(13.7550810514531,5.,73.9965952330688));
#39332=CARTESIAN_POINT('Ctrl Pts',(13.8006472240049,-5.,73.9888836296951));
#39333=CARTESIAN_POINT('Ctrl Pts',(13.8006472240049,5.,73.9888836296951));
#39334=CARTESIAN_POINT('Ctrl Pts',(13.8375902833446,-5.,73.9831411376432));
#39335=CARTESIAN_POINT('Ctrl Pts',(13.8375902833446,5.,73.9831411376432));
#39336=CARTESIAN_POINT('Ctrl Pts',(13.8655712938679,-5.,73.9790727181811));
#39337=CARTESIAN_POINT('Ctrl Pts',(13.8655712938679,5.,73.9790727181811));
#39338=CARTESIAN_POINT('Ctrl Pts',(13.8843467322659,-5.,73.9764662244028));
#39339=CARTESIAN_POINT('Ctrl Pts',(13.8843467322659,5.,73.9764662244028));
#39340=CARTESIAN_POINT('Ctrl Pts',(13.8937648093287,-5.,73.9751894239903));
#39341=CARTESIAN_POINT('Ctrl Pts',(13.8937648093287,5.,73.9751894239903));
#39342=CARTESIAN_POINT('Ctrl Pts',(13.7759884897161,-4.8,73.993137535462));
#39343=CARTESIAN_POINT('Ctrl Pts',(13.7759884897161,-3.13333333333333,73.993137535462));
#39344=CARTESIAN_POINT('Ctrl Pts',(13.7759884897161,-1.46666666666667,73.993137535462));
#39345=CARTESIAN_POINT('Ctrl Pts',(13.7759884897161,1.73333333333333,73.993137535462));
#39346=CARTESIAN_POINT('Ctrl Pts',(13.7759884897161,3.26666666666667,73.993137535462));
#39347=CARTESIAN_POINT('Ctrl Pts',(13.7759884897161,4.8,73.993137535462));
#39348=CARTESIAN_POINT('',(12.8475953086752,0.,74.3620957389297));
#39349=CARTESIAN_POINT('Origin',(12.5915348397961,0.,74.7054546451438));
#39350=CARTESIAN_POINT('Ctrl Pts',(15.0874706089091,-5.,76.0427485181531));
#39351=CARTESIAN_POINT('Ctrl Pts',(15.0874706089091,5.,76.0427485181531));
#39352=CARTESIAN_POINT('Ctrl Pts',(15.0816558287596,-5.,76.0502664118982));
#39353=CARTESIAN_POINT('Ctrl Pts',(15.0816558287596,5.,76.0502664118982));
#39354=CARTESIAN_POINT('Ctrl Pts',(15.0700108196895,-5.,76.0652231715592));
#39355=CARTESIAN_POINT('Ctrl Pts',(15.0700108196895,5.,76.0652231715592));
#39356=CARTESIAN_POINT('Ctrl Pts',(15.0524969597726,-5.,76.0874212276898));
#39357=CARTESIAN_POINT('Ctrl Pts',(15.0524969597726,5.,76.0874212276898));
#39358=CARTESIAN_POINT('Ctrl Pts',(15.029052286077,-5.,76.1165436095022));
#39359=CARTESIAN_POINT('Ctrl Pts',(15.029052286077,5.,76.1165436095022));
#39360=CARTESIAN_POINT('Ctrl Pts',(14.999590755387,-5.,76.1521492708168));
#39361=CARTESIAN_POINT('Ctrl Pts',(14.999590755387,5.,76.1521492708168));
#39362=CARTESIAN_POINT('Ctrl Pts',(14.9699724759961,-5.,76.186949488945));
#39363=CARTESIAN_POINT('Ctrl Pts',(14.9699724759961,5.,76.186949488945));
#39364=CARTESIAN_POINT('Ctrl Pts',(14.9401966272196,-5.,76.22093467639));
#39365=CARTESIAN_POINT('Ctrl Pts',(14.9401966272196,5.,76.22093467639));
#39366=CARTESIAN_POINT('Ctrl Pts',(14.9102630483799,-5.,76.2540949261266));
#39367=CARTESIAN_POINT('Ctrl Pts',(14.9102630483799,5.,76.2540949261266));
#39368=CARTESIAN_POINT('Ctrl Pts',(14.8801726478579,-5.,76.2864213632965));
#39369=CARTESIAN_POINT('Ctrl Pts',(14.8801726478579,5.,76.2864213632965));
#39370=CARTESIAN_POINT('Ctrl Pts',(14.8499279571665,-5.,76.3179073881206));
#39371=CARTESIAN_POINT('Ctrl Pts',(14.8499279571665,5.,76.3179073881206));
#39372=CARTESIAN_POINT('Ctrl Pts',(14.8195358101786,-5.,76.3485465262688));
#39373=CARTESIAN_POINT('Ctrl Pts',(14.8195358101786,5.,76.3485465262688));
#39374=CARTESIAN_POINT('Ctrl Pts',(14.7890097781812,-5.,76.3783306878053));
#39375=CARTESIAN_POINT('Ctrl Pts',(14.7890097781812,5.,76.3783306878053));
#39376=CARTESIAN_POINT('Ctrl Pts',(14.7583731025724,-5.,76.4072483152522));
#39377=CARTESIAN_POINT('Ctrl Pts',(14.7583731025724,5.,76.4072483152522));
#39378=CARTESIAN_POINT('Ctrl Pts',(14.7276607659748,-5.,76.4352830347113));
#39379=CARTESIAN_POINT('Ctrl Pts',(14.7276607659748,5.,76.4352830347113));
#39380=CARTESIAN_POINT('Ctrl Pts',(14.6969238755583,-5.,76.4624115358413));
#39381=CARTESIAN_POINT('Ctrl Pts',(14.6969238755583,5.,76.4624115358413));
#39382=CARTESIAN_POINT('Ctrl Pts',(14.6662264394396,-5.,76.4886045504555));
#39383=CARTESIAN_POINT('Ctrl Pts',(14.6662264394396,5.,76.4886045504555));
#39384=CARTESIAN_POINT('Ctrl Pts',(14.6356328340581,-5.,76.5138315797917));
#39385=CARTESIAN_POINT('Ctrl Pts',(14.6356328340581,5.,76.5138315797917));
#39386=CARTESIAN_POINT('Ctrl Pts',(14.6051972349025,-5.,76.5380650014057));
#39387=CARTESIAN_POINT('Ctrl Pts',(14.6051972349025,5.,76.5380650014057));
#39388=CARTESIAN_POINT('Ctrl Pts',(14.5749530575496,-5.,76.5612842962772));
#39389=CARTESIAN_POINT('Ctrl Pts',(14.5749530575496,5.,76.5612842962772));
#39390=CARTESIAN_POINT('Ctrl Pts',(14.5449001535355,-5.,76.583481316641));
#39391=CARTESIAN_POINT('Ctrl Pts',(14.5449001535355,5.,76.583481316641));
#39392=CARTESIAN_POINT('Ctrl Pts',(14.5149987482656,-5.,76.6046629918255));
#39393=CARTESIAN_POINT('Ctrl Pts',(14.5149987482656,5.,76.6046629918255));
#39394=CARTESIAN_POINT('Ctrl Pts',(14.4852084852497,-5.,76.6248360933492));
#39395=CARTESIAN_POINT('Ctrl Pts',(14.4852084852497,5.,76.6248360933492));
#39396=CARTESIAN_POINT('Ctrl Pts',(14.4555238389698,-5.,76.6439936173949));
#39397=CARTESIAN_POINT('Ctrl Pts',(14.4555238389698,5.,76.6439936173949));
#39398=CARTESIAN_POINT('Ctrl Pts',(14.4260085031102,-5.,76.6621016876444));
#39399=CARTESIAN_POINT('Ctrl Pts',(14.4260085031102,5.,76.6621016876444));
#39400=CARTESIAN_POINT('Ctrl Pts',(14.3968367013156,-5.,76.6790839349479));
#39401=CARTESIAN_POINT('Ctrl Pts',(14.3968367013156,5.,76.6790839349479));
#39402=CARTESIAN_POINT('Ctrl Pts',(14.3683140305578,-5.,76.6948139561085));
#39403=CARTESIAN_POINT('Ctrl Pts',(14.3683140305578,5.,76.6948139561085));
#39404=CARTESIAN_POINT('Ctrl Pts',(14.3408088953677,-5.,76.709142427651));
#39405=CARTESIAN_POINT('Ctrl Pts',(14.3408088953677,5.,76.709142427651));
#39406=CARTESIAN_POINT('Ctrl Pts',(14.3146943136958,-5.,76.7219204938828));
#39407=CARTESIAN_POINT('Ctrl Pts',(14.3146943136958,5.,76.7219204938828));
#39408=CARTESIAN_POINT('Ctrl Pts',(14.2902911577409,-5.,76.7330224855497));
#39409=CARTESIAN_POINT('Ctrl Pts',(14.2902911577409,5.,76.7330224855497));
#39410=CARTESIAN_POINT('Ctrl Pts',(14.2677963745262,-5.,76.7423753282655));
#39411=CARTESIAN_POINT('Ctrl Pts',(14.2677963745262,5.,76.7423753282655));
#39412=CARTESIAN_POINT('Ctrl Pts',(14.2513960065121,-5.,76.7484364250213));
#39413=CARTESIAN_POINT('Ctrl Pts',(14.2513960065121,5.,76.7484364250213));
#39414=CARTESIAN_POINT('Ctrl Pts',(14.2400033288828,-5.,76.7521814186714));
#39415=CARTESIAN_POINT('Ctrl Pts',(14.2400033288828,5.,76.7521814186714));
#39416=CARTESIAN_POINT('Ctrl Pts',(14.2328107850219,-5.,76.7543228322031));
#39417=CARTESIAN_POINT('Ctrl Pts',(14.2328107850219,5.,76.7543228322031));
#39418=CARTESIAN_POINT('Ctrl Pts',(14.2293151609602,-5.,76.7553047249138));
#39419=CARTESIAN_POINT('Ctrl Pts',(14.2293151609602,5.,76.7553047249138));
#39420=CARTESIAN_POINT('',(14.2293151609602,0.,76.7553047249138));
#39421=CARTESIAN_POINT('Ctrl Pts',(15.0130389285309,4.8,76.1357717468986));
#39422=CARTESIAN_POINT('Ctrl Pts',(15.0130389285309,3.13333333333333,76.1357717468986));
#39423=CARTESIAN_POINT('Ctrl Pts',(15.0130389285309,1.46666666666667,76.1357717468986));
#39424=CARTESIAN_POINT('Ctrl Pts',(15.0130389285309,-1.73333333333333,76.1357717468986));
#39425=CARTESIAN_POINT('Ctrl Pts',(15.0130389285309,-3.26666666666667,76.1357717468986));
#39426=CARTESIAN_POINT('Ctrl Pts',(15.0130389285309,-4.8,76.1357717468986));
#39427=CARTESIAN_POINT('Origin',(9.30999999999972,0.,78.0000000000001));
#39428=CARTESIAN_POINT('',(13.941494462579,0.,77.5855617740846));
#39429=CARTESIAN_POINT('',(13.8039273911235,0.,76.805380142761));
#39430=CARTESIAN_POINT('Origin',(14.2293151609602,0.,76.7553047249138));
#39431=CARTESIAN_POINT('Ctrl Pts',(14.3583550124563,-5.,77.4871260887099));
#39432=CARTESIAN_POINT('Ctrl Pts',(14.3583550124563,5.,77.4871260887099));
#39433=CARTESIAN_POINT('Ctrl Pts',(14.3619756516734,-5.,77.4868531921847));
#39434=CARTESIAN_POINT('Ctrl Pts',(14.3619756516734,5.,77.4868531921847));
#39435=CARTESIAN_POINT('Ctrl Pts',(14.3694668386202,-5.,77.4864054677684));
#39436=CARTESIAN_POINT('Ctrl Pts',(14.3694668386202,5.,77.4864054677684));
#39437=CARTESIAN_POINT('Ctrl Pts',(14.3814533169788,-5.,77.486028085408));
#39438=CARTESIAN_POINT('Ctrl Pts',(14.3814533169788,5.,77.486028085408));
#39439=CARTESIAN_POINT('Ctrl Pts',(14.3989376389619,-5.,77.4861143970885));
#39440=CARTESIAN_POINT('Ctrl Pts',(14.3989376389619,5.,77.4861143970885));
#39441=CARTESIAN_POINT('Ctrl Pts',(14.4232746813706,-5.,77.4872095254305));
#39442=CARTESIAN_POINT('Ctrl Pts',(14.4232746813706,5.,77.4872095254305));
#39443=CARTESIAN_POINT('Ctrl Pts',(14.4500032517364,-5.,77.4892956142184));
#39444=CARTESIAN_POINT('Ctrl Pts',(14.4500032517364,5.,77.4892956142184));
#39445=CARTESIAN_POINT('Ctrl Pts',(14.478913287478,-5.,77.4923713558196));
#39446=CARTESIAN_POINT('Ctrl Pts',(14.478913287478,5.,77.4923713558196));
#39447=CARTESIAN_POINT('Ctrl Pts',(14.5096602859406,-5.,77.4964284045148));
#39448=CARTESIAN_POINT('Ctrl Pts',(14.5096602859406,5.,77.4964284045148));
#39449=CARTESIAN_POINT('Ctrl Pts',(14.5418428132648,-5.,77.5014544613684));
#39450=CARTESIAN_POINT('Ctrl Pts',(14.5418428132648,5.,77.5014544613684));
#39451=CARTESIAN_POINT('Ctrl Pts',(14.575063610798,-5.,77.5074352099942));
#39452=CARTESIAN_POINT('Ctrl Pts',(14.575063610798,5.,77.5074352099942));
#39453=CARTESIAN_POINT('Ctrl Pts',(14.6089922788841,-5.,77.5143563905722));
#39454=CARTESIAN_POINT('Ctrl Pts',(14.6089922788841,5.,77.5143563905722));
#39455=CARTESIAN_POINT('Ctrl Pts',(14.6434389810628,-5.,77.5222058275741));
#39456=CARTESIAN_POINT('Ctrl Pts',(14.6434389810628,5.,77.5222058275741));
#39457=CARTESIAN_POINT('Ctrl Pts',(14.6783322784657,-5.,77.5309734721938));
#39458=CARTESIAN_POINT('Ctrl Pts',(14.6783322784657,5.,77.5309734721938));
#39459=CARTESIAN_POINT('Ctrl Pts',(14.7136749679333,-5.,77.5406508531512));
#39460=CARTESIAN_POINT('Ctrl Pts',(14.7136749679333,5.,77.5406508531512));
#39461=CARTESIAN_POINT('Ctrl Pts',(14.7495072881561,-5.,77.5512305308537));
#39462=CARTESIAN_POINT('Ctrl Pts',(14.7495072881561,5.,77.5512305308537));
#39463=CARTESIAN_POINT('Ctrl Pts',(14.7858689849959,-5.,77.5627054130239));
#39464=CARTESIAN_POINT('Ctrl Pts',(14.7858689849959,5.,77.5627054130239));
#39465=CARTESIAN_POINT('Ctrl Pts',(14.8227574112639,-5.,77.575067792493));
#39466=CARTESIAN_POINT('Ctrl Pts',(14.8227574112639,5.,77.575067792493));
#39467=CARTESIAN_POINT('Ctrl Pts',(14.8601341486718,-5.,77.5883098164962));
#39468=CARTESIAN_POINT('Ctrl Pts',(14.8601341486718,5.,77.5883098164962));
#39469=CARTESIAN_POINT('Ctrl Pts',(14.8979388414815,-5.,77.6024240575431));
#39470=CARTESIAN_POINT('Ctrl Pts',(14.8979388414815,5.,77.6024240575431));
#39471=CARTESIAN_POINT('Ctrl Pts',(14.936100564438,-5.,77.6174038742163));
#39472=CARTESIAN_POINT('Ctrl Pts',(14.936100564438,5.,77.6174038742163));
#39473=CARTESIAN_POINT('Ctrl Pts',(14.9745491592773,-5.,77.6332436554837));
#39474=CARTESIAN_POINT('Ctrl Pts',(14.9745491592773,5.,77.6332436554837));
#39475=CARTESIAN_POINT('Ctrl Pts',(15.0132286283616,-5.,77.6499389764632));
#39476=CARTESIAN_POINT('Ctrl Pts',(15.0132286283616,5.,77.6499389764632));
#39477=CARTESIAN_POINT('Ctrl Pts',(15.0521004985737,-5.,77.6674864154704));
#39478=CARTESIAN_POINT('Ctrl Pts',(15.0521004985737,5.,77.6674864154704));
#39479=CARTESIAN_POINT('Ctrl Pts',(15.0911389772507,-5.,77.685883061039));
#39480=CARTESIAN_POINT('Ctrl Pts',(15.0911389772507,5.,77.685883061039));
#39481=CARTESIAN_POINT('Ctrl Pts',(15.1303285446315,-5.,77.705125952756));
#39482=CARTESIAN_POINT('Ctrl Pts',(15.1303285446315,5.,77.705125952756));
#39483=CARTESIAN_POINT('Ctrl Pts',(15.1696605646238,-5.,77.7252113440577));
#39484=CARTESIAN_POINT('Ctrl Pts',(15.1696605646238,5.,77.7252113440577));
#39485=CARTESIAN_POINT('Ctrl Pts',(15.2091304011272,-5.,77.7461338990148));
#39486=CARTESIAN_POINT('Ctrl Pts',(15.2091304011272,5.,77.7461338990148));
#39487=CARTESIAN_POINT('Ctrl Pts',(15.2487341651656,-5.,77.7678855886962));
#39488=CARTESIAN_POINT('Ctrl Pts',(15.2487341651656,5.,77.7678855886962));
#39489=CARTESIAN_POINT('Ctrl Pts',(15.2884686193296,-5.,77.7904570486235));
#39490=CARTESIAN_POINT('Ctrl Pts',(15.2884686193296,5.,77.7904570486235));
#39491=CARTESIAN_POINT('Ctrl Pts',(15.3283312556985,-5.,77.8138389888447));
#39492=CARTESIAN_POINT('Ctrl Pts',(15.3283312556985,5.,77.8138389888447));
#39493=CARTESIAN_POINT('Ctrl Pts',(15.3603224837765,-5.,77.8331865255343));
#39494=CARTESIAN_POINT('Ctrl Pts',(15.3603224837765,5.,77.8331865255343));
#39495=CARTESIAN_POINT('Ctrl Pts',(15.3843723110553,-5.,77.8480557822982));
#39496=CARTESIAN_POINT('Ctrl Pts',(15.3843723110553,5.,77.8480557822982));
#39497=CARTESIAN_POINT('Ctrl Pts',(15.4004305532434,-5.,77.8581277114053));
#39498=CARTESIAN_POINT('Ctrl Pts',(15.4004305532434,5.,77.8581277114053));
#39499=CARTESIAN_POINT('Ctrl Pts',(15.408465930345,-5.,77.8632034487949));
#39500=CARTESIAN_POINT('Ctrl Pts',(15.408465930345,5.,77.8632034487949));
#39501=CARTESIAN_POINT('Ctrl Pts',(15.3067072115039,-4.8,77.8012473409061));
#39502=CARTESIAN_POINT('Ctrl Pts',(15.3067072115039,-3.13333333333333,77.8012473409061));
#39503=CARTESIAN_POINT('Ctrl Pts',(15.3067072115039,-1.46666666666667,77.8012473409061));
#39504=CARTESIAN_POINT('Ctrl Pts',(15.3067072115039,1.73333333333333,77.8012473409061));
#39505=CARTESIAN_POINT('Ctrl Pts',(15.3067072115039,3.26666666666667,77.8012473409061));
#39506=CARTESIAN_POINT('Ctrl Pts',(15.3067072115039,4.8,77.8012473409061));
#39507=CARTESIAN_POINT('',(14.3583550124563,0.,77.4871260887099));
#39508=CARTESIAN_POINT('Origin',(13.941494462579,0.,77.5855617740846));
#39509=CARTESIAN_POINT('Ctrl Pts',(15.408465930345,-5.,78.1367965512051));
#39510=CARTESIAN_POINT('Ctrl Pts',(15.408465930345,5.,78.1367965512051));
#39511=CARTESIAN_POINT('Ctrl Pts',(15.4004305532433,-5.,78.1418722885381));
#39512=CARTESIAN_POINT('Ctrl Pts',(15.4004305532433,5.,78.1418722885381));
#39513=CARTESIAN_POINT('Ctrl Pts',(15.3843723110551,-5.,78.1519442175461));
#39514=CARTESIAN_POINT('Ctrl Pts',(15.3843723110551,5.,78.1519442175461));
#39515=CARTESIAN_POINT('Ctrl Pts',(15.3603224837762,-5.,78.1668134742034));
#39516=CARTESIAN_POINT('Ctrl Pts',(15.3603224837762,5.,78.1668134742034));
#39517=CARTESIAN_POINT('Ctrl Pts',(15.3283312556981,-5.,78.1861610108314));
#39518=CARTESIAN_POINT('Ctrl Pts',(15.3283312556981,5.,78.1861610108314));
#39519=CARTESIAN_POINT('Ctrl Pts',(15.2884686193292,-5.,78.2095429510792));
#39520=CARTESIAN_POINT('Ctrl Pts',(15.2884686193292,5.,78.2095429510792));
#39521=CARTESIAN_POINT('Ctrl Pts',(15.2487341651653,-5.,78.2321144110984));
#39522=CARTESIAN_POINT('Ctrl Pts',(15.2487341651653,5.,78.2321144110984));
#39523=CARTESIAN_POINT('Ctrl Pts',(15.2091304011271,-5.,78.2538661008963));
#39524=CARTESIAN_POINT('Ctrl Pts',(15.2091304011271,5.,78.2538661008963));
#39525=CARTESIAN_POINT('Ctrl Pts',(15.1696605646239,-5.,78.2747886559577));
#39526=CARTESIAN_POINT('Ctrl Pts',(15.1696605646239,5.,78.2747886559577));
#39527=CARTESIAN_POINT('Ctrl Pts',(15.1303285446317,-5.,78.2948740473268));
#39528=CARTESIAN_POINT('Ctrl Pts',(15.1303285446317,5.,78.2948740473268));
#39529=CARTESIAN_POINT('Ctrl Pts',(15.0911389772509,-5.,78.3141169390679));
#39530=CARTESIAN_POINT('Ctrl Pts',(15.0911389772509,5.,78.3141169390679));
#39531=CARTESIAN_POINT('Ctrl Pts',(15.0521004985739,-5.,78.3325135846235));
#39532=CARTESIAN_POINT('Ctrl Pts',(15.0521004985739,5.,78.3325135846235));
#39533=CARTESIAN_POINT('Ctrl Pts',(15.0132286283617,-5.,78.3500610235947));
#39534=CARTESIAN_POINT('Ctrl Pts',(15.0132286283617,5.,78.3500610235947));
#39535=CARTESIAN_POINT('Ctrl Pts',(14.9745491592773,-5.,78.3667563445323));
#39536=CARTESIAN_POINT('Ctrl Pts',(14.9745491592773,5.,78.3667563445323));
#39537=CARTESIAN_POINT('Ctrl Pts',(14.936100564438,-5.,78.3825961257675));
#39538=CARTESIAN_POINT('Ctrl Pts',(14.936100564438,5.,78.3825961257675));
#39539=CARTESIAN_POINT('Ctrl Pts',(14.8979388414814,-5.,78.3975759424268));
#39540=CARTESIAN_POINT('Ctrl Pts',(14.8979388414814,5.,78.3975759424268));
#39541=CARTESIAN_POINT('Ctrl Pts',(14.8601341486718,-5.,78.4116901834755));
#39542=CARTESIAN_POINT('Ctrl Pts',(14.8601341486718,5.,78.4116901834755));
#39543=CARTESIAN_POINT('Ctrl Pts',(14.8227574112638,-5.,78.4249322074904));
#39544=CARTESIAN_POINT('Ctrl Pts',(14.8227574112638,5.,78.4249322074904));
#39545=CARTESIAN_POINT('Ctrl Pts',(14.7858689849959,-5.,78.4372945869721));
#39546=CARTESIAN_POINT('Ctrl Pts',(14.7858689849959,5.,78.4372945869721));
#39547=CARTESIAN_POINT('Ctrl Pts',(14.7495072881561,-5.,78.4487694691489));
#39548=CARTESIAN_POINT('Ctrl Pts',(14.7495072881561,5.,78.4487694691489));
#39549=CARTESIAN_POINT('Ctrl Pts',(14.7136749679335,-5.,78.4593491468485));
#39550=CARTESIAN_POINT('Ctrl Pts',(14.7136749679335,5.,78.4593491468485));
#39551=CARTESIAN_POINT('Ctrl Pts',(14.678332278466,-5.,78.4690265277979));
#39552=CARTESIAN_POINT('Ctrl Pts',(14.678332278466,5.,78.4690265277979));
#39553=CARTESIAN_POINT('Ctrl Pts',(14.6434389810631,-5.,78.4777941724113));
#39554=CARTESIAN_POINT('Ctrl Pts',(14.6434389810631,5.,78.4777941724113));
#39555=CARTESIAN_POINT('Ctrl Pts',(14.6089922788842,-5.,78.4856436094153));
#39556=CARTESIAN_POINT('Ctrl Pts',(14.6089922788842,5.,78.4856436094153));
#39557=CARTESIAN_POINT('Ctrl Pts',(14.575063610798,-5.,78.492564790007));
#39558=CARTESIAN_POINT('Ctrl Pts',(14.575063610798,5.,78.492564790007));
#39559=CARTESIAN_POINT('Ctrl Pts',(14.5418428132646,-5.,78.498545538655));
#39560=CARTESIAN_POINT('Ctrl Pts',(14.5418428132646,5.,78.498545538655));
#39561=CARTESIAN_POINT('Ctrl Pts',(14.5096602859403,-5.,78.5035715955264));
#39562=CARTESIAN_POINT('Ctrl Pts',(14.5096602859403,5.,78.5035715955264));
#39563=CARTESIAN_POINT('Ctrl Pts',(14.4789132874778,-5.,78.5076286442221));
#39564=CARTESIAN_POINT('Ctrl Pts',(14.4789132874778,5.,78.5076286442221));
#39565=CARTESIAN_POINT('Ctrl Pts',(14.4500032517364,-5.,78.5107043857979));
#39566=CARTESIAN_POINT('Ctrl Pts',(14.4500032517364,5.,78.5107043857979));
#39567=CARTESIAN_POINT('Ctrl Pts',(14.4232746813707,-5.,78.5127904745387));
#39568=CARTESIAN_POINT('Ctrl Pts',(14.4232746813707,5.,78.5127904745387));
#39569=CARTESIAN_POINT('Ctrl Pts',(14.3989376389621,-5.,78.513885602836));
#39570=CARTESIAN_POINT('Ctrl Pts',(14.3989376389621,5.,78.513885602836));
#39571=CARTESIAN_POINT('Ctrl Pts',(14.3814533169789,-5.,78.5139719145117));
#39572=CARTESIAN_POINT('Ctrl Pts',(14.3814533169789,5.,78.5139719145117));
#39573=CARTESIAN_POINT('Ctrl Pts',(14.3694668386203,-5.,78.5135945321781));
#39574=CARTESIAN_POINT('Ctrl Pts',(14.3694668386203,5.,78.5135945321781));
#39575=CARTESIAN_POINT('Ctrl Pts',(14.3619756516734,-5.,78.5131468077949));
#39576=CARTESIAN_POINT('Ctrl Pts',(14.3619756516734,5.,78.5131468077949));
#39577=CARTESIAN_POINT('Ctrl Pts',(14.3583550124563,-5.,78.5128739112901));
#39578=CARTESIAN_POINT('Ctrl Pts',(14.3583550124563,5.,78.5128739112901));
#39579=CARTESIAN_POINT('',(14.3583550124563,0.,78.5128739112901));
#39580=CARTESIAN_POINT('Ctrl Pts',(15.306707211514,4.8,78.1987526587886));
#39581=CARTESIAN_POINT('Ctrl Pts',(15.306707211514,3.13333333333333,78.1987526587886));
#39582=CARTESIAN_POINT('Ctrl Pts',(15.306707211514,1.46666666666667,78.1987526587886));
#39583=CARTESIAN_POINT('Ctrl Pts',(15.306707211514,-1.73333333333333,78.1987526587886));
#39584=CARTESIAN_POINT('Ctrl Pts',(15.306707211514,-3.26666666666667,78.1987526587886));
#39585=CARTESIAN_POINT('Ctrl Pts',(15.306707211514,-4.8,78.1987526587886));
#39586=CARTESIAN_POINT('Origin',(9.30999999999925,0.,77.9999999999999));
#39587=CARTESIAN_POINT('',(13.8039273911235,0.,79.194619857239));
#39588=CARTESIAN_POINT('',(13.941494462579,0.,78.4144382259154));
#39589=CARTESIAN_POINT('Origin',(14.3583550124563,0.,78.5128739112901));
#39590=CARTESIAN_POINT('Ctrl Pts',(14.2293151609602,-5.,79.2446952750862));
#39591=CARTESIAN_POINT('Ctrl Pts',(14.2293151609602,5.,79.2446952750862));
#39592=CARTESIAN_POINT('Ctrl Pts',(14.2328107850219,-5.,79.2456771677792));
#39593=CARTESIAN_POINT('Ctrl Pts',(14.2328107850219,5.,79.2456771677792));
#39594=CARTESIAN_POINT('Ctrl Pts',(14.2400033288829,-5.,79.247818581282));
#39595=CARTESIAN_POINT('Ctrl Pts',(14.2400033288829,5.,79.247818581282));
#39596=CARTESIAN_POINT('Ctrl Pts',(14.2513960065123,-5.,79.2515635749088));
#39597=CARTESIAN_POINT('Ctrl Pts',(14.2513960065123,5.,79.2515635749088));
#39598=CARTESIAN_POINT('Ctrl Pts',(14.2677963745263,-5.,79.2576246716687));
#39599=CARTESIAN_POINT('Ctrl Pts',(14.2677963745263,5.,79.2576246716687));
#39600=CARTESIAN_POINT('Ctrl Pts',(14.290291157741,-5.,79.2669775144234));
#39601=CARTESIAN_POINT('Ctrl Pts',(14.290291157741,5.,79.2669775144234));
#39602=CARTESIAN_POINT('Ctrl Pts',(14.3146943136958,-5.,79.2780795061314));
#39603=CARTESIAN_POINT('Ctrl Pts',(14.3146943136958,5.,79.2780795061314));
#39604=CARTESIAN_POINT('Ctrl Pts',(14.3408088953677,-5.,79.2908575723857));
#39605=CARTESIAN_POINT('Ctrl Pts',(14.3408088953677,5.,79.2908575723857));
#39606=CARTESIAN_POINT('Ctrl Pts',(14.3683140305578,-5.,79.305186043928));
#39607=CARTESIAN_POINT('Ctrl Pts',(14.3683140305578,5.,79.305186043928));
#39608=CARTESIAN_POINT('Ctrl Pts',(14.3968367013155,-5.,79.3209160650726));
#39609=CARTESIAN_POINT('Ctrl Pts',(14.3968367013155,5.,79.3209160650726));
#39610=CARTESIAN_POINT('Ctrl Pts',(14.4260085031102,-5.,79.3378983123566));
#39611=CARTESIAN_POINT('Ctrl Pts',(14.4260085031102,5.,79.3378983123566));
#39612=CARTESIAN_POINT('Ctrl Pts',(14.4555238389699,-5.,79.3560063825941));
#39613=CARTESIAN_POINT('Ctrl Pts',(14.4555238389699,5.,79.3560063825941));
#39614=CARTESIAN_POINT('Ctrl Pts',(14.4852084852499,-5.,79.3751639066383));
#39615=CARTESIAN_POINT('Ctrl Pts',(14.4852084852499,5.,79.3751639066383));
#39616=CARTESIAN_POINT('Ctrl Pts',(14.514998748266,-5.,79.395337008168));
#39617=CARTESIAN_POINT('Ctrl Pts',(14.514998748266,5.,79.395337008168));
#39618=CARTESIAN_POINT('Ctrl Pts',(14.5449001535359,-5.,79.4165186833593));
#39619=CARTESIAN_POINT('Ctrl Pts',(14.5449001535359,5.,79.4165186833593));
#39620=CARTESIAN_POINT('Ctrl Pts',(14.5749530575497,-5.,79.4387157037252));
#39621=CARTESIAN_POINT('Ctrl Pts',(14.5749530575497,5.,79.4387157037252));
#39622=CARTESIAN_POINT('Ctrl Pts',(14.6051972349022,-5.,79.4619349985905));
#39623=CARTESIAN_POINT('Ctrl Pts',(14.6051972349022,5.,79.4619349985905));
#39624=CARTESIAN_POINT('Ctrl Pts',(14.6356328340575,-5.,79.4861684201933));
#39625=CARTESIAN_POINT('Ctrl Pts',(14.6356328340575,5.,79.4861684201933));
#39626=CARTESIAN_POINT('Ctrl Pts',(14.6662264394389,-5.,79.5113954495195));
#39627=CARTESIAN_POINT('Ctrl Pts',(14.6662264394389,5.,79.5113954495195));
#39628=CARTESIAN_POINT('Ctrl Pts',(14.6969238755576,-5.,79.5375884641322));
#39629=CARTESIAN_POINT('Ctrl Pts',(14.6969238755576,5.,79.5375884641322));
#39630=CARTESIAN_POINT('Ctrl Pts',(14.7276607659746,-5.,79.5647169652746));
#39631=CARTESIAN_POINT('Ctrl Pts',(14.7276607659746,5.,79.5647169652746));
#39632=CARTESIAN_POINT('Ctrl Pts',(14.7583731025727,-5.,79.5927516847618));
#39633=CARTESIAN_POINT('Ctrl Pts',(14.7583731025727,5.,79.5927516847618));
#39634=CARTESIAN_POINT('Ctrl Pts',(14.789009778182,-5.,79.6216693122451));
#39635=CARTESIAN_POINT('Ctrl Pts',(14.789009778182,5.,79.6216693122451));
#39636=CARTESIAN_POINT('Ctrl Pts',(14.8195358101796,-5.,79.6514534738131));
#39637=CARTESIAN_POINT('Ctrl Pts',(14.8195358101796,5.,79.6514534738131));
#39638=CARTESIAN_POINT('Ctrl Pts',(14.8499279571675,-5.,79.6820926119728));
#39639=CARTESIAN_POINT('Ctrl Pts',(14.8499279571675,5.,79.6820926119728));
#39640=CARTESIAN_POINT('Ctrl Pts',(14.8801726478586,-5.,79.7135786367758));
#39641=CARTESIAN_POINT('Ctrl Pts',(14.8801726478586,5.,79.7135786367758));
#39642=CARTESIAN_POINT('Ctrl Pts',(14.91026304838,-5.,79.7459050738868));
#39643=CARTESIAN_POINT('Ctrl Pts',(14.91026304838,5.,79.7459050738868));
#39644=CARTESIAN_POINT('Ctrl Pts',(14.9401966272191,-5.,79.7790653235324));
#39645=CARTESIAN_POINT('Ctrl Pts',(14.9401966272191,5.,79.7790653235324));
#39646=CARTESIAN_POINT('Ctrl Pts',(14.969972475995,-5.,79.8130505108762));
#39647=CARTESIAN_POINT('Ctrl Pts',(14.969972475995,5.,79.8130505108762));
#39648=CARTESIAN_POINT('Ctrl Pts',(14.9995907553857,-5.,79.8478507289248));
#39649=CARTESIAN_POINT('Ctrl Pts',(14.9995907553857,5.,79.8478507289248));
#39650=CARTESIAN_POINT('Ctrl Pts',(15.0290522860757,-5.,79.8834563902168));
#39651=CARTESIAN_POINT('Ctrl Pts',(15.0290522860757,5.,79.8834563902168));
#39652=CARTESIAN_POINT('Ctrl Pts',(15.0524969597716,-5.,79.9125787720828));
#39653=CARTESIAN_POINT('Ctrl Pts',(15.0524969597716,5.,79.9125787720828));
#39654=CARTESIAN_POINT('Ctrl Pts',(15.0700108196889,-5.,79.934776828306));
#39655=CARTESIAN_POINT('Ctrl Pts',(15.0700108196889,5.,79.934776828306));
#39656=CARTESIAN_POINT('Ctrl Pts',(15.0816558287594,-5.,79.9497335880528));
#39657=CARTESIAN_POINT('Ctrl Pts',(15.0816558287594,5.,79.9497335880528));
#39658=CARTESIAN_POINT('Ctrl Pts',(15.0874706089091,-5.,79.9572514818469));
#39659=CARTESIAN_POINT('Ctrl Pts',(15.0874706089091,5.,79.9572514818469));
#39660=CARTESIAN_POINT('Ctrl Pts',(15.0130389285914,-4.8,79.8642282529162));
#39661=CARTESIAN_POINT('Ctrl Pts',(15.0130389285914,-3.13333333333333,79.8642282529162));
#39662=CARTESIAN_POINT('Ctrl Pts',(15.0130389285914,-1.46666666666667,79.8642282529162));
#39663=CARTESIAN_POINT('Ctrl Pts',(15.0130389285914,1.73333333333333,79.8642282529162));
#39664=CARTESIAN_POINT('Ctrl Pts',(15.0130389285914,3.26666666666667,79.8642282529162));
#39665=CARTESIAN_POINT('Ctrl Pts',(15.0130389285914,4.8,79.8642282529162));
#39666=CARTESIAN_POINT('',(14.2293151609602,0.,79.2446952750862));
#39667=CARTESIAN_POINT('Origin',(13.8039273911235,0.,79.194619857239));
#39668=CARTESIAN_POINT('Ctrl Pts',(13.8937648093287,-5.,82.0248105760097));
#39669=CARTESIAN_POINT('Ctrl Pts',(13.8937648093287,5.,82.0248105760097));
#39670=CARTESIAN_POINT('Ctrl Pts',(13.8843467322662,-5.,82.0235337755467));
#39671=CARTESIAN_POINT('Ctrl Pts',(13.8843467322662,5.,82.0235337755467));
#39672=CARTESIAN_POINT('Ctrl Pts',(13.8655712938686,-5.,82.02092728168));
#39673=CARTESIAN_POINT('Ctrl Pts',(13.8655712938686,5.,82.02092728168));
#39674=CARTESIAN_POINT('Ctrl Pts',(13.8375902833457,-5.,82.0168588621226));
#39675=CARTESIAN_POINT('Ctrl Pts',(13.8375902833457,5.,82.0168588621226));
#39676=CARTESIAN_POINT('Ctrl Pts',(13.8006472240062,-5.,82.0111163700153));
#39677=CARTESIAN_POINT('Ctrl Pts',(13.8006472240062,5.,82.0111163700153));
#39678=CARTESIAN_POINT('Ctrl Pts',(13.7550810514543,-5.,82.0034047666646));
#39679=CARTESIAN_POINT('Ctrl Pts',(13.7550810514543,5.,82.0034047666646));
#39680=CARTESIAN_POINT('Ctrl Pts',(13.7101340388377,-5.,81.9951546933737));
#39681=CARTESIAN_POINT('Ctrl Pts',(13.7101340388377,5.,81.9951546933737));
#39682=CARTESIAN_POINT('Ctrl Pts',(13.6658140788142,-5.,81.9863606456546));
#39683=CARTESIAN_POINT('Ctrl Pts',(13.6658140788142,5.,81.9863606456546));
#39684=CARTESIAN_POINT('Ctrl Pts',(13.6221296707664,-5.,81.9770175308379));
#39685=CARTESIAN_POINT('Ctrl Pts',(13.6221296707664,5.,81.9770175308379));
#39686=CARTESIAN_POINT('Ctrl Pts',(13.579088954728,-5.,81.9671216981718));
#39687=CARTESIAN_POINT('Ctrl Pts',(13.579088954728,5.,81.9671216981718));
#39688=CARTESIAN_POINT('Ctrl Pts',(13.5366989120296,-5.,81.9566720401197));
#39689=CARTESIAN_POINT('Ctrl Pts',(13.5366989120296,5.,81.9566720401197));
#39690=CARTESIAN_POINT('Ctrl Pts',(13.4949685665442,-5.,81.9456712378251));
#39691=CARTESIAN_POINT('Ctrl Pts',(13.4949685665442,5.,81.9456712378251));
#39692=CARTESIAN_POINT('Ctrl Pts',(13.4539117100108,-5.,81.9341269994011));
#39693=CARTESIAN_POINT('Ctrl Pts',(13.4539117100108,5.,81.9341269994011));
#39694=CARTESIAN_POINT('Ctrl Pts',(13.4135499722044,-5.,81.9220536737527));
#39695=CARTESIAN_POINT('Ctrl Pts',(13.4135499722044,5.,81.9220536737527));
#39696=CARTESIAN_POINT('Ctrl Pts',(13.3739150246538,-5.,81.9094733697732));
#39697=CARTESIAN_POINT('Ctrl Pts',(13.3739150246538,5.,81.9094733697732));
#39698=CARTESIAN_POINT('Ctrl Pts',(13.3350526082949,-5.,81.8964186924009));
#39699=CARTESIAN_POINT('Ctrl Pts',(13.3350526082949,5.,81.8964186924009));
#39700=CARTESIAN_POINT('Ctrl Pts',(13.2970200741786,-5.,81.8829304401978));
#39701=CARTESIAN_POINT('Ctrl Pts',(13.2970200741786,5.,81.8829304401978));
#39702=CARTESIAN_POINT('Ctrl Pts',(13.2598760232249,-5.,81.8690491154141));
#39703=CARTESIAN_POINT('Ctrl Pts',(13.2598760232249,5.,81.8690491154141));
#39704=CARTESIAN_POINT('Ctrl Pts',(13.2236714649137,-5.,81.8548078241759));
#39705=CARTESIAN_POINT('Ctrl Pts',(13.2236714649137,5.,81.8548078241759));
#39706=CARTESIAN_POINT('Ctrl Pts',(13.1884408770234,-5.,81.8402252457097));
#39707=CARTESIAN_POINT('Ctrl Pts',(13.1884408770234,5.,81.8402252457097));
#39708=CARTESIAN_POINT('Ctrl Pts',(13.1541912414923,-5.,81.8252971775583));
#39709=CARTESIAN_POINT('Ctrl Pts',(13.1541912414923,5.,81.8252971775583));
#39710=CARTESIAN_POINT('Ctrl Pts',(13.1208966700501,-5.,81.8099926385766));
#39711=CARTESIAN_POINT('Ctrl Pts',(13.1208966700501,5.,81.8099926385766));
#39712=CARTESIAN_POINT('Ctrl Pts',(13.0885311201469,-5.,81.7942800647796));
#39713=CARTESIAN_POINT('Ctrl Pts',(13.0885311201469,5.,81.7942800647796));
#39714=CARTESIAN_POINT('Ctrl Pts',(13.0570978945104,-5.,81.7781511690216));
#39715=CARTESIAN_POINT('Ctrl Pts',(13.0570978945104,5.,81.7781511690216));
#39716=CARTESIAN_POINT('Ctrl Pts',(13.0266581777357,-5.,81.7616441734931));
#39717=CARTESIAN_POINT('Ctrl Pts',(13.0266581777357,5.,81.7616441734931));
#39718=CARTESIAN_POINT('Ctrl Pts',(12.9973652192683,-5.,81.7448717757205));
#39719=CARTESIAN_POINT('Ctrl Pts',(12.9973652192683,5.,81.7448717757205));
#39720=CARTESIAN_POINT('Ctrl Pts',(12.9694812859689,-5.,81.7280354288443));
#39721=CARTESIAN_POINT('Ctrl Pts',(12.9694812859689,5.,81.7280354288443));
#39722=CARTESIAN_POINT('Ctrl Pts',(12.9433198980207,-5.,81.7113795188064));
#39723=CARTESIAN_POINT('Ctrl Pts',(12.9433198980207,5.,81.7113795188064));
#39724=CARTESIAN_POINT('Ctrl Pts',(12.9191964772076,-5.,81.6951526607806));
#39725=CARTESIAN_POINT('Ctrl Pts',(12.9191964772076,5.,81.6951526607806));
#39726=CARTESIAN_POINT('Ctrl Pts',(12.897380292397,-5.,81.6795699036158));
#39727=CARTESIAN_POINT('Ctrl Pts',(12.897380292397,5.,81.6795699036158));
#39728=CARTESIAN_POINT('Ctrl Pts',(12.8780331013841,-5.,81.6647652712487));
#39729=CARTESIAN_POINT('Ctrl Pts',(12.8780331013841,5.,81.6647652712487));
#39730=CARTESIAN_POINT('Ctrl Pts',(12.8645838536101,-5.,81.653592684294));
#39731=CARTESIAN_POINT('Ctrl Pts',(12.8645838536101,5.,81.653592684294));
#39732=CARTESIAN_POINT('Ctrl Pts',(12.8556442551671,-5.,81.6455988328799));
#39733=CARTESIAN_POINT('Ctrl Pts',(12.8556442551671,5.,81.6455988328799));
#39734=CARTESIAN_POINT('Ctrl Pts',(12.85019346473,-5.,81.6404406139507));
#39735=CARTESIAN_POINT('Ctrl Pts',(12.85019346473,5.,81.6404406139507));
#39736=CARTESIAN_POINT('Ctrl Pts',(12.8475953086752,-5.,81.6379042610703));
#39737=CARTESIAN_POINT('Ctrl Pts',(12.8475953086752,5.,81.6379042610703));
#39738=CARTESIAN_POINT('',(12.8475953086752,0.,81.6379042610703));
#39739=CARTESIAN_POINT('Ctrl Pts',(13.7759884899248,4.8,82.0068624643054));
#39740=CARTESIAN_POINT('Ctrl Pts',(13.7759884899248,3.13333333333333,82.0068624643054));
#39741=CARTESIAN_POINT('Ctrl Pts',(13.7759884899248,1.46666666666667,82.0068624643054));
#39742=CARTESIAN_POINT('Ctrl Pts',(13.7759884899248,-1.73333333333333,82.0068624643054));
#39743=CARTESIAN_POINT('Ctrl Pts',(13.7759884899248,-3.26666666666667,82.0068624643054));
#39744=CARTESIAN_POINT('Ctrl Pts',(13.7759884899248,-4.8,82.0068624643054));
#39745=CARTESIAN_POINT('Origin',(9.31000000000031,0.,78.0000000000004));
#39746=CARTESIAN_POINT('',(11.9846612632316,0.,81.8037727491227));
#39747=CARTESIAN_POINT('',(12.5915348397961,0.,81.2945453548562));
#39748=CARTESIAN_POINT('Origin',(12.8475953086752,0.,81.6379042610703));
#39749=CARTESIAN_POINT('Ctrl Pts',(12.2783393423437,-5.,82.1155667324646));
#39750=CARTESIAN_POINT('Ctrl Pts',(12.2783393423437,5.,82.1155667324646));
#39751=CARTESIAN_POINT('Ctrl Pts',(12.2803859972687,-5.,82.1185658497385));
#39752=CARTESIAN_POINT('Ctrl Pts',(12.2803859972687,5.,82.1185658497385));
#39753=CARTESIAN_POINT('Ctrl Pts',(12.2845193314492,-5.,82.124829545725));
#39754=CARTESIAN_POINT('Ctrl Pts',(12.2845193314492,5.,82.124829545725));
#39755=CARTESIAN_POINT('Ctrl Pts',(12.2908393933303,-5.,82.1350214493006));
#39756=CARTESIAN_POINT('Ctrl Pts',(12.2908393933303,5.,82.1350214493006));
#39757=CARTESIAN_POINT('Ctrl Pts',(12.2995068062155,-5.,82.1502064721471));
#39758=CARTESIAN_POINT('Ctrl Pts',(12.2995068062155,5.,82.1502064721471));
#39759=CARTESIAN_POINT('Ctrl Pts',(12.3107269184707,-5.,82.1718305333045));
#39760=CARTESIAN_POINT('Ctrl Pts',(12.3107269184707,5.,82.1718305333045));
#39761=CARTESIAN_POINT('Ctrl Pts',(12.3222845977848,-5.,82.1960211986505));
#39762=CARTESIAN_POINT('Ctrl Pts',(12.3222845977848,5.,82.1960211986505));
#39763=CARTESIAN_POINT('Ctrl Pts',(12.334075945302,-5.,82.2225958948322));
#39764=CARTESIAN_POINT('Ctrl Pts',(12.334075945302,5.,82.2225958948322));
#39765=CARTESIAN_POINT('Ctrl Pts',(12.3459359372985,-5.,82.2512521009388));
#39766=CARTESIAN_POINT('Ctrl Pts',(12.3459359372985,5.,82.2512521009388));
#39767=CARTESIAN_POINT('Ctrl Pts',(12.3576745080383,-5.,82.2816360155831));
#39768=CARTESIAN_POINT('Ctrl Pts',(12.3576745080383,5.,82.2816360155831));
#39769=CARTESIAN_POINT('Ctrl Pts',(12.369105426554,-5.,82.3133964444896));
#39770=CARTESIAN_POINT('Ctrl Pts',(12.369105426554,5.,82.3133964444896));
#39771=CARTESIAN_POINT('Ctrl Pts',(12.3800758423883,-5.,82.3462401232546));
#39772=CARTESIAN_POINT('Ctrl Pts',(12.3800758423883,5.,82.3462401232546));
#39773=CARTESIAN_POINT('Ctrl Pts',(12.3905013816289,-5.,82.3799965609175));
#39774=CARTESIAN_POINT('Ctrl Pts',(12.3905013816289,5.,82.3799965609175));
#39775=CARTESIAN_POINT('Ctrl Pts',(12.4003550273611,-5.,82.4145988652004));
#39776=CARTESIAN_POINT('Ctrl Pts',(12.4003550273611,5.,82.4145988652004));
#39777=CARTESIAN_POINT('Ctrl Pts',(12.4096455143463,-5.,82.4500452225975));
#39778=CARTESIAN_POINT('Ctrl Pts',(12.4096455143463,5.,82.4500452225975));
#39779=CARTESIAN_POINT('Ctrl Pts',(12.418399404803,-5.,82.4863667610403));
#39780=CARTESIAN_POINT('Ctrl Pts',(12.418399404803,5.,82.4863667610403));
#39781=CARTESIAN_POINT('Ctrl Pts',(12.4266427137534,-5.,82.5235943553157));
#39782=CARTESIAN_POINT('Ctrl Pts',(12.4266427137534,5.,82.5235943553157));
#39783=CARTESIAN_POINT('Ctrl Pts',(12.4343807922091,-5.,82.5617218593056));
#39784=CARTESIAN_POINT('Ctrl Pts',(12.4343807922091,5.,82.5617218593056));
#39785=CARTESIAN_POINT('Ctrl Pts',(12.4416012317233,-5.,82.6007120754133));
#39786=CARTESIAN_POINT('Ctrl Pts',(12.4416012317233,5.,82.6007120754133));
#39787=CARTESIAN_POINT('Ctrl Pts',(12.4482802868263,-5.,82.6405090202912));
#39788=CARTESIAN_POINT('Ctrl Pts',(12.4482802868263,5.,82.6405090202912));
#39789=CARTESIAN_POINT('Ctrl Pts',(12.4543882465293,-5.,82.6810479501583));
#39790=CARTESIAN_POINT('Ctrl Pts',(12.4543882465293,5.,82.6810479501583));
#39791=CARTESIAN_POINT('Ctrl Pts',(12.4598948909969,-5.,82.7222653006607));
#39792=CARTESIAN_POINT('Ctrl Pts',(12.4598948909969,5.,82.7222653006607));
#39793=CARTESIAN_POINT('Ctrl Pts',(12.4647760534665,-5.,82.7641103639807));
#39794=CARTESIAN_POINT('Ctrl Pts',(12.4647760534665,5.,82.7641103639807));
#39795=CARTESIAN_POINT('Ctrl Pts',(12.4690154606377,-5.,82.8065481105801));
#39796=CARTESIAN_POINT('Ctrl Pts',(12.4690154606377,5.,82.8065481105801));
#39797=CARTESIAN_POINT('Ctrl Pts',(12.4726027375752,-5.,82.8495547476242));
#39798=CARTESIAN_POINT('Ctrl Pts',(12.4726027375752,5.,82.8495547476242));
#39799=CARTESIAN_POINT('Ctrl Pts',(12.4755326881847,-5.,82.8931153543989));
#39800=CARTESIAN_POINT('Ctrl Pts',(12.4755326881847,5.,82.8931153543989));
#39801=CARTESIAN_POINT('Ctrl Pts',(12.4778042390369,-5.,82.9372205785469));
#39802=CARTESIAN_POINT('Ctrl Pts',(12.4778042390369,5.,82.9372205785469));
#39803=CARTESIAN_POINT('Ctrl Pts',(12.4794196931349,-5.,82.9818637371221));
#39804=CARTESIAN_POINT('Ctrl Pts',(12.4794196931349,5.,82.9818637371221));
#39805=CARTESIAN_POINT('Ctrl Pts',(12.4803840592604,-5.,83.0270374477065));
#39806=CARTESIAN_POINT('Ctrl Pts',(12.4803840592604,5.,83.0270374477065));
#39807=CARTESIAN_POINT('Ctrl Pts',(12.4807038286021,-5.,83.072734224382));
#39808=CARTESIAN_POINT('Ctrl Pts',(12.4807038286021,5.,83.072734224382));
#39809=CARTESIAN_POINT('Ctrl Pts',(12.480385792553,-5.,83.1189472502496));
#39810=CARTESIAN_POINT('Ctrl Pts',(12.480385792553,5.,83.1189472502496));
#39811=CARTESIAN_POINT('Ctrl Pts',(12.4796259483469,-5.,83.1563262348074));
#39812=CARTESIAN_POINT('Ctrl Pts',(12.4796259483469,5.,83.1563262348074));
#39813=CARTESIAN_POINT('Ctrl Pts',(12.478773707943,-5.,83.1845886245686));
#39814=CARTESIAN_POINT('Ctrl Pts',(12.478773707943,5.,83.1845886245686));
#39815=CARTESIAN_POINT('Ctrl Pts',(12.4780802826114,-5.,83.2035314347966));
#39816=CARTESIAN_POINT('Ctrl Pts',(12.4780802826114,5.,83.2035314347966));
#39817=CARTESIAN_POINT('Ctrl Pts',(12.4777022536662,-5.,83.2130281441901));
#39818=CARTESIAN_POINT('Ctrl Pts',(12.4777022536662,5.,83.2130281441901));
#39819=CARTESIAN_POINT('Ctrl Pts',(12.4804784574569,-4.8,83.0939244547599));
#39820=CARTESIAN_POINT('Ctrl Pts',(12.4804784574569,-3.13333333333333,83.0939244547599));
#39821=CARTESIAN_POINT('Ctrl Pts',(12.4804784574569,-1.46666666666667,83.0939244547599));
#39822=CARTESIAN_POINT('Ctrl Pts',(12.4804784574569,1.73333333333333,83.0939244547599));
#39823=CARTESIAN_POINT('Ctrl Pts',(12.4804784574569,3.26666666666667,83.09392445476));
#39824=CARTESIAN_POINT('Ctrl Pts',(12.4804784574569,4.8,83.09392445476));
#39825=CARTESIAN_POINT('',(12.2783393423437,0.,82.1155667324646));
#39826=CARTESIAN_POINT('Origin',(11.9846612632316,0.,81.8037727491227));
#39827=CARTESIAN_POINT('Ctrl Pts',(10.2342691911562,-5.,84.0295710015124));
#39828=CARTESIAN_POINT('Ctrl Pts',(10.2342691911562,5.,84.0295710015124));
#39829=CARTESIAN_POINT('Ctrl Pts',(10.2278752370576,-5.,84.0225390923711));
#39830=CARTESIAN_POINT('Ctrl Pts',(10.2278752370576,5.,84.0225390923711));
#39831=CARTESIAN_POINT('Ctrl Pts',(10.2151678387374,-5.,84.0084737830622));
#39832=CARTESIAN_POINT('Ctrl Pts',(10.2151678387374,5.,84.0084737830622));
#39833=CARTESIAN_POINT('Ctrl Pts',(10.1963482707627,-5.,83.9873713459997));
#39834=CARTESIAN_POINT('Ctrl Pts',(10.1963482707627,5.,83.9873713459997));
#39835=CARTESIAN_POINT('Ctrl Pts',(10.1717394481999,-5.,83.9592258010255));
#39836=CARTESIAN_POINT('Ctrl Pts',(10.1717394481999,5.,83.9592258010255));
#39837=CARTESIAN_POINT('Ctrl Pts',(10.1417906580151,-5.,83.9240289989938));
#39838=CARTESIAN_POINT('Ctrl Pts',(10.1417906580151,5.,83.9240289989938));
#39839=CARTESIAN_POINT('Ctrl Pts',(10.1126622936843,-5.,83.8888176933897));
#39840=CARTESIAN_POINT('Ctrl Pts',(10.1126622936843,5.,83.8888176933897));
#39841=CARTESIAN_POINT('Ctrl Pts',(10.0843639395383,-5.,83.8535927408343));
#39842=CARTESIAN_POINT('Ctrl Pts',(10.0843639395383,5.,83.8535927408343));
#39843=CARTESIAN_POINT('Ctrl Pts',(10.056905379975,-5.,83.8183557034152));
#39844=CARTESIAN_POINT('Ctrl Pts',(10.056905379975,5.,83.8183557034152));
#39845=CARTESIAN_POINT('Ctrl Pts',(10.0302951972726,-5.,83.7831090168075));
#39846=CARTESIAN_POINT('Ctrl Pts',(10.0302951972726,5.,83.7831090168075));
#39847=CARTESIAN_POINT('Ctrl Pts',(10.004539451349,-5.,83.7478563201022));
#39848=CARTESIAN_POINT('Ctrl Pts',(10.004539451349,5.,83.7478563201022));
#39849=CARTESIAN_POINT('Ctrl Pts',(9.97964333148819,-5.,83.7126054676082));
#39850=CARTESIAN_POINT('Ctrl Pts',(9.97964333148819,5.,83.7126054676082));
#39851=CARTESIAN_POINT('Ctrl Pts',(9.95561244809968,-5.,83.6773712292418));
#39852=CARTESIAN_POINT('Ctrl Pts',(9.95561244809968,5.,83.6773712292418));
#39853=CARTESIAN_POINT('Ctrl Pts',(9.93245414725961,-5.,83.6421785002535));
#39854=CARTESIAN_POINT('Ctrl Pts',(9.93245414725961,5.,83.6421785002535));
#39855=CARTESIAN_POINT('Ctrl Pts',(9.91017847944887,-5.,83.607064575104));
#39856=CARTESIAN_POINT('Ctrl Pts',(9.91017847944887,5.,83.607064575104));
#39857=CARTESIAN_POINT('Ctrl Pts',(9.88879952620944,-5.,83.5720838323314));
#39858=CARTESIAN_POINT('Ctrl Pts',(9.88879952620944,5.,83.5720838323314));
#39859=CARTESIAN_POINT('Ctrl Pts',(9.86833499618459,-5.,83.537304389991));
#39860=CARTESIAN_POINT('Ctrl Pts',(9.86833499618459,5.,83.537304389991));
#39861=CARTESIAN_POINT('Ctrl Pts',(9.84880374593727,-5.,83.5027949425508));
#39862=CARTESIAN_POINT('Ctrl Pts',(9.84880374593727,5.,83.5027949425508));
#39863=CARTESIAN_POINT('Ctrl Pts',(9.83022357078563,-5.,83.4686136390358));
#39864=CARTESIAN_POINT('Ctrl Pts',(9.83022357078563,5.,83.4686136390358));
#39865=CARTESIAN_POINT('Ctrl Pts',(9.81260887546256,-5.,83.4347969504531));
#39866=CARTESIAN_POINT('Ctrl Pts',(9.81260887546256,5.,83.4347969504531));
#39867=CARTESIAN_POINT('Ctrl Pts',(9.79596770972913,-5.,83.4013461454384));
#39868=CARTESIAN_POINT('Ctrl Pts',(9.79596770972913,5.,83.4013461454384));
#39869=CARTESIAN_POINT('Ctrl Pts',(9.78030015631686,-5.,83.3682208504004));
#39870=CARTESIAN_POINT('Ctrl Pts',(9.78030015631686,5.,83.3682208504004));
#39871=CARTESIAN_POINT('Ctrl Pts',(9.76560655441585,-5.,83.3353801460973));
#39872=CARTESIAN_POINT('Ctrl Pts',(9.76560655441585,5.,83.3353801460973));
#39873=CARTESIAN_POINT('Ctrl Pts',(9.75189476093909,-5.,83.30281980716));
#39874=CARTESIAN_POINT('Ctrl Pts',(9.75189476093909,5.,83.30281980716));
#39875=CARTESIAN_POINT('Ctrl Pts',(9.73918707725655,-5.,83.270608442185));
#39876=CARTESIAN_POINT('Ctrl Pts',(9.73918707725655,5.,83.270608442185));
#39877=CARTESIAN_POINT('Ctrl Pts',(9.72752845867955,-5.,83.2389308893288));
#39878=CARTESIAN_POINT('Ctrl Pts',(9.72752845867955,5.,83.2389308893288));
#39879=CARTESIAN_POINT('Ctrl Pts',(9.71699032169307,-5.,83.2081100525341));
#39880=CARTESIAN_POINT('Ctrl Pts',(9.71699032169307,5.,83.2081100525341));
#39881=CARTESIAN_POINT('Ctrl Pts',(9.70765574843163,-5.,83.1785346691788));
#39882=CARTESIAN_POINT('Ctrl Pts',(9.70765574843163,5.,83.1785346691788));
#39883=CARTESIAN_POINT('Ctrl Pts',(9.69960655924427,-5.,83.1505979387468));
#39884=CARTESIAN_POINT('Ctrl Pts',(9.69960655924427,5.,83.1505979387468));
#39885=CARTESIAN_POINT('Ctrl Pts',(9.69291079531643,-5.,83.1246376809074));
#39886=CARTESIAN_POINT('Ctrl Pts',(9.69291079531643,5.,83.1246376809074));
#39887=CARTESIAN_POINT('Ctrl Pts',(9.6876062213894,-5.,83.1008605398683));
#39888=CARTESIAN_POINT('Ctrl Pts',(9.6876062213894,5.,83.1008605398683));
#39889=CARTESIAN_POINT('Ctrl Pts',(9.68448510032915,-5.,83.0836568318856));
#39890=CARTESIAN_POINT('Ctrl Pts',(9.68448510032915,5.,83.0836568318856));
#39891=CARTESIAN_POINT('Ctrl Pts',(9.68277531926867,-5.,83.0717869233261));
#39892=CARTESIAN_POINT('Ctrl Pts',(9.68277531926867,5.,83.0717869233261));
#39893=CARTESIAN_POINT('Ctrl Pts',(9.68191541076936,-5.,83.0643317978355));
#39894=CARTESIAN_POINT('Ctrl Pts',(9.68191541076936,5.,83.0643317978355));
#39895=CARTESIAN_POINT('Ctrl Pts',(9.68155544397255,-5.,83.0607187762934));
#39896=CARTESIAN_POINT('Ctrl Pts',(9.68155544397255,5.,83.0607187762934));
#39897=CARTESIAN_POINT('',(9.68155544397255,0.,83.0607187762934));
#39898=CARTESIAN_POINT('Ctrl Pts',(10.1555841198781,4.8,83.9401167914621));
#39899=CARTESIAN_POINT('Ctrl Pts',(10.1555841198781,3.13333333333333,83.9401167914621));
#39900=CARTESIAN_POINT('Ctrl Pts',(10.1555841198781,1.46666666666667,83.9401167914621));
#39901=CARTESIAN_POINT('Ctrl Pts',(10.1555841198781,-1.73333333333333,83.9401167914621));
#39902=CARTESIAN_POINT('Ctrl Pts',(10.1555841198781,-3.26666666666667,83.9401167914621));
#39903=CARTESIAN_POINT('Ctrl Pts',(10.1555841198781,-4.8,83.9401167914621));
#39904=CARTESIAN_POINT('Origin',(9.31,0.,78.0000000000002));
#39905=CARTESIAN_POINT('',(8.91389140472481,0.,82.6330980974667));
#39906=CARTESIAN_POINT('',(9.70610859527519,0.,82.6330980974667));
#39907=CARTESIAN_POINT('Origin',(9.68155544397255,0.,83.0607187762934));
#39908=CARTESIAN_POINT('Ctrl Pts',(8.93844455602746,-5.,83.0607187762934));
#39909=CARTESIAN_POINT('Ctrl Pts',(8.93844455602746,5.,83.0607187762934));
#39910=CARTESIAN_POINT('Ctrl Pts',(8.93808458922896,-5.,83.0643317978355));
#39911=CARTESIAN_POINT('Ctrl Pts',(8.93808458922896,5.,83.0643317978355));
#39912=CARTESIAN_POINT('Ctrl Pts',(8.93722468072689,-5.,83.0717869233258));
#39913=CARTESIAN_POINT('Ctrl Pts',(8.93722468072689,5.,83.0717869233258));
#39914=CARTESIAN_POINT('Ctrl Pts',(8.93551489966416,-5.,83.0836568318852));
#39915=CARTESIAN_POINT('Ctrl Pts',(8.93551489966416,5.,83.0836568318852));
#39916=CARTESIAN_POINT('Ctrl Pts',(8.93239377860429,-5.,83.1008605398679));
#39917=CARTESIAN_POINT('Ctrl Pts',(8.93239377860429,5.,83.1008605398679));
#39918=CARTESIAN_POINT('Ctrl Pts',(8.92708920468098,-5.,83.1246376809072));
#39919=CARTESIAN_POINT('Ctrl Pts',(8.92708920468098,5.,83.1246376809072));
#39920=CARTESIAN_POINT('Ctrl Pts',(8.92039344075711,-5.,83.1505979387469));
#39921=CARTESIAN_POINT('Ctrl Pts',(8.92039344075711,5.,83.1505979387469));
#39922=CARTESIAN_POINT('Ctrl Pts',(8.91234425157185,-5.,83.178534669179));
#39923=CARTESIAN_POINT('Ctrl Pts',(8.91234425157185,5.,83.178534669179));
#39924=CARTESIAN_POINT('Ctrl Pts',(8.90300967831031,-5.,83.2081100525344));
#39925=CARTESIAN_POINT('Ctrl Pts',(8.90300967831031,5.,83.2081100525344));
#39926=CARTESIAN_POINT('Ctrl Pts',(8.89247154132227,-5.,83.2389308893288));
#39927=CARTESIAN_POINT('Ctrl Pts',(8.89247154132227,5.,83.2389308893288));
#39928=CARTESIAN_POINT('Ctrl Pts',(8.88081292274349,-5.,83.270608442185));
#39929=CARTESIAN_POINT('Ctrl Pts',(8.88081292274349,5.,83.270608442185));
#39930=CARTESIAN_POINT('Ctrl Pts',(8.86810523906001,-5.,83.30281980716));
#39931=CARTESIAN_POINT('Ctrl Pts',(8.86810523906001,5.,83.30281980716));
#39932=CARTESIAN_POINT('Ctrl Pts',(8.85439344558332,-5.,83.3353801460974));
#39933=CARTESIAN_POINT('Ctrl Pts',(8.85439344558332,5.,83.3353801460974));
#39934=CARTESIAN_POINT('Ctrl Pts',(8.839699843683,-5.,83.3682208504006));
#39935=CARTESIAN_POINT('Ctrl Pts',(8.839699843683,5.,83.3682208504006));
#39936=CARTESIAN_POINT('Ctrl Pts',(8.82403229027133,-5.,83.4013461454385));
#39937=CARTESIAN_POINT('Ctrl Pts',(8.82403229027133,5.,83.4013461454385));
#39938=CARTESIAN_POINT('Ctrl Pts',(8.80739112453778,-5.,83.4347969504531));
#39939=CARTESIAN_POINT('Ctrl Pts',(8.80739112453778,5.,83.4347969504531));
#39940=CARTESIAN_POINT('Ctrl Pts',(8.78977642921359,-5.,83.4686136390359));
#39941=CARTESIAN_POINT('Ctrl Pts',(8.78977642921359,5.,83.4686136390359));
#39942=CARTESIAN_POINT('Ctrl Pts',(8.77119625406031,-5.,83.5027949425511));
#39943=CARTESIAN_POINT('Ctrl Pts',(8.77119625406031,5.,83.5027949425511));
#39944=CARTESIAN_POINT('Ctrl Pts',(8.75166500381164,-5.,83.5373043899916));
#39945=CARTESIAN_POINT('Ctrl Pts',(8.75166500381164,5.,83.5373043899916));
#39946=CARTESIAN_POINT('Ctrl Pts',(8.7312004737867,-5.,83.5720838323321));
#39947=CARTESIAN_POINT('Ctrl Pts',(8.7312004737867,5.,83.5720838323321));
#39948=CARTESIAN_POINT('Ctrl Pts',(8.70982152054912,-5.,83.6070645751044));
#39949=CARTESIAN_POINT('Ctrl Pts',(8.70982152054912,5.,83.6070645751044));
#39950=CARTESIAN_POINT('Ctrl Pts',(8.68754585274241,-5.,83.6421785002532));
#39951=CARTESIAN_POINT('Ctrl Pts',(8.68754585274241,5.,83.6421785002532));
#39952=CARTESIAN_POINT('Ctrl Pts',(8.66438755190743,-5.,83.6773712292402));
#39953=CARTESIAN_POINT('Ctrl Pts',(8.66438755190743,5.,83.6773712292402));
#39954=CARTESIAN_POINT('Ctrl Pts',(8.64035666852326,-5.,83.7126054676056));
#39955=CARTESIAN_POINT('Ctrl Pts',(8.64035666852326,5.,83.7126054676056));
#39956=CARTESIAN_POINT('Ctrl Pts',(8.61546054866391,-5.,83.7478563200994));
#39957=CARTESIAN_POINT('Ctrl Pts',(8.61546054866391,5.,83.7478563200994));
#39958=CARTESIAN_POINT('Ctrl Pts',(8.58970480273733,-5.,83.7831090168055));
#39959=CARTESIAN_POINT('Ctrl Pts',(8.58970480273733,5.,83.7831090168055));
#39960=CARTESIAN_POINT('Ctrl Pts',(8.5630946200268,-5.,83.8183557034149));
#39961=CARTESIAN_POINT('Ctrl Pts',(8.5630946200268,5.,83.8183557034149));
#39962=CARTESIAN_POINT('Ctrl Pts',(8.53563606045106,-5.,83.8535927408361));
#39963=CARTESIAN_POINT('Ctrl Pts',(8.53563606045106,5.,83.8535927408361));
#39964=CARTESIAN_POINT('Ctrl Pts',(8.50733770629117,-5.,83.8888176933934));
#39965=CARTESIAN_POINT('Ctrl Pts',(8.50733770629117,5.,83.8888176933934));
#39966=CARTESIAN_POINT('Ctrl Pts',(8.47820934194942,-5.,83.9240289989987));
#39967=CARTESIAN_POINT('Ctrl Pts',(8.47820934194942,5.,83.9240289989987));
#39968=CARTESIAN_POINT('Ctrl Pts',(8.44826055176156,-5.,83.9592258010304));
#39969=CARTESIAN_POINT('Ctrl Pts',(8.44826055176156,5.,83.9592258010304));
#39970=CARTESIAN_POINT('Ctrl Pts',(8.42365172920609,-5.,83.9873713460034));
#39971=CARTESIAN_POINT('Ctrl Pts',(8.42365172920609,5.,83.9873713460034));
#39972=CARTESIAN_POINT('Ctrl Pts',(8.40483216124414,-5.,84.0084737830643));
#39973=CARTESIAN_POINT('Ctrl Pts',(8.40483216124414,5.,84.0084737830643));
#39974=CARTESIAN_POINT('Ctrl Pts',(8.3921247629357,-5.,84.0225390923718));
#39975=CARTESIAN_POINT('Ctrl Pts',(8.3921247629357,5.,84.0225390923718));
#39976=CARTESIAN_POINT('Ctrl Pts',(8.38573080884383,-5.,84.0295710015124));
#39977=CARTESIAN_POINT('Ctrl Pts',(8.38573080884383,5.,84.0295710015124));
#39978=CARTESIAN_POINT('Ctrl Pts',(8.46441588009367,-4.8,83.9401167914581));
#39979=CARTESIAN_POINT('Ctrl Pts',(8.46441588009367,-3.13333333333333,83.9401167914581));
#39980=CARTESIAN_POINT('Ctrl Pts',(8.46441588009367,-1.46666666666667,83.9401167914581));
#39981=CARTESIAN_POINT('Ctrl Pts',(8.46441588009367,1.73333333333333,83.9401167914581));
#39982=CARTESIAN_POINT('Ctrl Pts',(8.46441588009368,3.26666666666667,83.9401167914581));
#39983=CARTESIAN_POINT('Ctrl Pts',(8.46441588009368,4.8,83.9401167914581));
#39984=CARTESIAN_POINT('',(8.93844455602746,0.,83.0607187762934));
#39985=CARTESIAN_POINT('Origin',(8.91389140472481,0.,82.6330980974667));
#39986=CARTESIAN_POINT('Ctrl Pts',(6.14229774633382,-5.,83.2130281441901));
#39987=CARTESIAN_POINT('Ctrl Pts',(6.14229774633382,5.,83.2130281441901));
#39988=CARTESIAN_POINT('Ctrl Pts',(6.14191971738338,-5.,83.2035314347958));
#39989=CARTESIAN_POINT('Ctrl Pts',(6.14191971738338,5.,83.2035314347958));
#39990=CARTESIAN_POINT('Ctrl Pts',(6.14122629204258,-5.,83.1845886245663));
#39991=CARTESIAN_POINT('Ctrl Pts',(6.14122629204258,5.,83.1845886245663));
#39992=CARTESIAN_POINT('Ctrl Pts',(6.14037405162884,-5.,83.1563262348033));
#39993=CARTESIAN_POINT('Ctrl Pts',(6.14037405162884,5.,83.1563262348033));
#39994=CARTESIAN_POINT('Ctrl Pts',(6.13961420741709,-5.,83.1189472502444));
#39995=CARTESIAN_POINT('Ctrl Pts',(6.13961420741709,5.,83.1189472502444));
#39996=CARTESIAN_POINT('Ctrl Pts',(6.13929617137036,-5.,83.072734224377));
#39997=CARTESIAN_POINT('Ctrl Pts',(6.13929617137036,5.,83.072734224377));
#39998=CARTESIAN_POINT('Ctrl Pts',(6.13961594072051,-5.,83.0270374477027));
#39999=CARTESIAN_POINT('Ctrl Pts',(6.13961594072051,5.,83.0270374477027));
#40000=CARTESIAN_POINT('Ctrl Pts',(6.14058030685684,-5.,82.9818637371201));
#40001=CARTESIAN_POINT('Ctrl Pts',(6.14058030685684,5.,82.9818637371201));
#40002=CARTESIAN_POINT('Ctrl Pts',(6.14219576096457,-5.,82.9372205785471));
#40003=CARTESIAN_POINT('Ctrl Pts',(6.14219576096457,5.,82.9372205785471));
#40004=CARTESIAN_POINT('Ctrl Pts',(6.14446731182308,-5.,82.893115354401));
#40005=CARTESIAN_POINT('Ctrl Pts',(6.14446731182308,5.,82.893115354401));
#40006=CARTESIAN_POINT('Ctrl Pts',(6.14739726243497,-5.,82.8495547476274));
#40007=CARTESIAN_POINT('Ctrl Pts',(6.14739726243497,5.,82.8495547476274));
#40008=CARTESIAN_POINT('Ctrl Pts',(6.15098453937128,-5.,82.8065481105834));
#40009=CARTESIAN_POINT('Ctrl Pts',(6.15098453937128,5.,82.8065481105834));
#40010=CARTESIAN_POINT('Ctrl Pts',(6.15522394653913,-5.,82.7641103639832));
#40011=CARTESIAN_POINT('Ctrl Pts',(6.15522394653913,5.,82.7641103639832));
#40012=CARTESIAN_POINT('Ctrl Pts',(6.16010510900473,-5.,82.7222653006616));
#40013=CARTESIAN_POINT('Ctrl Pts',(6.16010510900473,5.,82.7222653006616));
#40014=CARTESIAN_POINT('Ctrl Pts',(6.16561175346913,-5.,82.6810479501576));
#40015=CARTESIAN_POINT('Ctrl Pts',(6.16561175346913,5.,82.6810479501576));
#40016=CARTESIAN_POINT('Ctrl Pts',(6.17171971317045,-5.,82.6405090202891));
#40017=CARTESIAN_POINT('Ctrl Pts',(6.17171971317045,5.,82.6405090202891));
#40018=CARTESIAN_POINT('Ctrl Pts',(6.17839876827339,-5.,82.6007120754106));
#40019=CARTESIAN_POINT('Ctrl Pts',(6.17839876827339,5.,82.6007120754106));
#40020=CARTESIAN_POINT('Ctrl Pts',(6.18561920778864,-5.,82.5617218593032));
#40021=CARTESIAN_POINT('Ctrl Pts',(6.18561920778864,5.,82.5617218593032));
#40022=CARTESIAN_POINT('Ctrl Pts',(6.19335728624576,-5.,82.5235943553145));
#40023=CARTESIAN_POINT('Ctrl Pts',(6.19335728624576,5.,82.5235943553145));
#40024=CARTESIAN_POINT('Ctrl Pts',(6.20160059519734,-5.,82.4863667610406));
#40025=CARTESIAN_POINT('Ctrl Pts',(6.20160059519734,5.,82.4863667610406));
#40026=CARTESIAN_POINT('Ctrl Pts',(6.21035448565451,-5.,82.4500452225988));
#40027=CARTESIAN_POINT('Ctrl Pts',(6.21035448565451,5.,82.4500452225988));
#40028=CARTESIAN_POINT('Ctrl Pts',(6.21964497263948,-5.,82.4145988652022));
#40029=CARTESIAN_POINT('Ctrl Pts',(6.21964497263948,5.,82.4145988652022));
#40030=CARTESIAN_POINT('Ctrl Pts',(6.22949861837122,-5.,82.3799965609194));
#40031=CARTESIAN_POINT('Ctrl Pts',(6.22949861837122,5.,82.3799965609194));
#40032=CARTESIAN_POINT('Ctrl Pts',(6.23992415761144,-5.,82.3462401232558));
#40033=CARTESIAN_POINT('Ctrl Pts',(6.23992415761144,5.,82.3462401232558));
#40034=CARTESIAN_POINT('Ctrl Pts',(6.25089457344595,-5.,82.3133964444894));
#40035=CARTESIAN_POINT('Ctrl Pts',(6.25089457344595,5.,82.3133964444894));
#40036=CARTESIAN_POINT('Ctrl Pts',(6.26232549196237,-5.,82.2816360155812));
#40037=CARTESIAN_POINT('Ctrl Pts',(6.26232549196237,5.,82.2816360155812));
#40038=CARTESIAN_POINT('Ctrl Pts',(6.27406406270293,-5.,82.2512521009353));
#40039=CARTESIAN_POINT('Ctrl Pts',(6.27406406270293,5.,82.2512521009353));
#40040=CARTESIAN_POINT('Ctrl Pts',(6.28592405469946,-5.,82.2225958948289));
#40041=CARTESIAN_POINT('Ctrl Pts',(6.28592405469946,5.,82.2225958948289));
#40042=CARTESIAN_POINT('Ctrl Pts',(6.29771540221578,-5.,82.1960211986491));
#40043=CARTESIAN_POINT('Ctrl Pts',(6.29771540221578,5.,82.1960211986491));
#40044=CARTESIAN_POINT('Ctrl Pts',(6.30927308152824,-5.,82.1718305333071));
#40045=CARTESIAN_POINT('Ctrl Pts',(6.30927308152824,5.,82.1718305333071));
#40046=CARTESIAN_POINT('Ctrl Pts',(6.32049319378186,-5.,82.1502064721534));
#40047=CARTESIAN_POINT('Ctrl Pts',(6.32049319378186,5.,82.1502064721534));
#40048=CARTESIAN_POINT('Ctrl Pts',(6.32916060666696,-5.,82.1350214493075));
#40049=CARTESIAN_POINT('Ctrl Pts',(6.32916060666696,5.,82.1350214493075));
#40050=CARTESIAN_POINT('Ctrl Pts',(6.33548066854901,-5.,82.1248295457296));
#40051=CARTESIAN_POINT('Ctrl Pts',(6.33548066854901,5.,82.1248295457296));
#40052=CARTESIAN_POINT('Ctrl Pts',(6.33961400273064,-5.,82.1185658497402));
#40053=CARTESIAN_POINT('Ctrl Pts',(6.33961400273064,5.,82.1185658497402));
#40054=CARTESIAN_POINT('Ctrl Pts',(6.34166065765632,-5.,82.1155667324646));
#40055=CARTESIAN_POINT('Ctrl Pts',(6.34166065765632,5.,82.1155667324646));
#40056=CARTESIAN_POINT('',(6.34166065765632,0.,82.1155667324646));
#40057=CARTESIAN_POINT('Ctrl Pts',(6.13952154251532,4.8,83.0939244547427));
#40058=CARTESIAN_POINT('Ctrl Pts',(6.13952154251532,3.13333333333333,83.0939244547427));
#40059=CARTESIAN_POINT('Ctrl Pts',(6.13952154251532,1.46666666666667,83.0939244547427));
#40060=CARTESIAN_POINT('Ctrl Pts',(6.13952154251532,-1.73333333333333,83.0939244547427));
#40061=CARTESIAN_POINT('Ctrl Pts',(6.13952154251532,-3.26666666666667,83.0939244547427));
#40062=CARTESIAN_POINT('Ctrl Pts',(6.13952154251532,-4.8,83.0939244547427));
#40063=CARTESIAN_POINT('Origin',(9.3100000000004,0.,77.9999999999995));
#40064=CARTESIAN_POINT('',(6.02846516020393,0.,81.2945453548562));
#40065=CARTESIAN_POINT('',(6.63533873676839,0.,81.8037727491227));
#40066=CARTESIAN_POINT('Origin',(6.34166065765632,0.,82.1155667324646));
#40067=CARTESIAN_POINT('Ctrl Pts',(5.77240469132478,-5.,81.6379042610703));
#40068=CARTESIAN_POINT('Ctrl Pts',(5.77240469132478,5.,81.6379042610703));
#40069=CARTESIAN_POINT('Ctrl Pts',(5.76980653526848,-5.,81.640440613956));
#40070=CARTESIAN_POINT('Ctrl Pts',(5.76980653526848,5.,81.640440613956));
#40071=CARTESIAN_POINT('Ctrl Pts',(5.76435574482894,-5.,81.6455988328939));
#40072=CARTESIAN_POINT('Ctrl Pts',(5.76435574482894,5.,81.6455988328939));
#40073=CARTESIAN_POINT('Ctrl Pts',(5.75541614638387,-5.,81.6535926843148));
#40074=CARTESIAN_POINT('Ctrl Pts',(5.75541614638387,5.,81.6535926843148));
#40075=CARTESIAN_POINT('Ctrl Pts',(5.74196689861022,-5.,81.664765271268));
#40076=CARTESIAN_POINT('Ctrl Pts',(5.74196689861022,5.,81.664765271268));
#40077=CARTESIAN_POINT('Ctrl Pts',(5.7226197076007,-5.,81.6795699036238));
#40078=CARTESIAN_POINT('Ctrl Pts',(5.7226197076007,5.,81.6795699036238));
#40079=CARTESIAN_POINT('Ctrl Pts',(5.70080352279367,-5.,81.6951526607764));
#40080=CARTESIAN_POINT('Ctrl Pts',(5.70080352279367,5.,81.6951526607764));
#40081=CARTESIAN_POINT('Ctrl Pts',(5.67668010198233,-5.,81.7113795187953));
#40082=CARTESIAN_POINT('Ctrl Pts',(5.67668010198233,5.,81.7113795187953));
#40083=CARTESIAN_POINT('Ctrl Pts',(5.65051871403411,-5.,81.7280354288328));
#40084=CARTESIAN_POINT('Ctrl Pts',(5.65051871403411,5.,81.7280354288328));
#40085=CARTESIAN_POINT('Ctrl Pts',(5.6226347807333,-5.,81.7448717757137));
#40086=CARTESIAN_POINT('Ctrl Pts',(5.6226347807333,5.,81.7448717757137));
#40087=CARTESIAN_POINT('Ctrl Pts',(5.59334182226431,-5.,81.7616441734925));
#40088=CARTESIAN_POINT('Ctrl Pts',(5.59334182226431,5.,81.7616441734925));
#40089=CARTESIAN_POINT('Ctrl Pts',(5.56290210548887,-5.,81.7781511690255));
#40090=CARTESIAN_POINT('Ctrl Pts',(5.56290210548887,5.,81.7781511690255));
#40091=CARTESIAN_POINT('Ctrl Pts',(5.53146887985245,-5.,81.7942800647846));
#40092=CARTESIAN_POINT('Ctrl Pts',(5.53146887985245,5.,81.7942800647846));
#40093=CARTESIAN_POINT('Ctrl Pts',(5.49910332995,-5.,81.8099926385801));
#40094=CARTESIAN_POINT('Ctrl Pts',(5.49910332995,5.,81.8099926385801));
#40095=CARTESIAN_POINT('Ctrl Pts',(5.46580875850822,-5.,81.8252971775594));
#40096=CARTESIAN_POINT('Ctrl Pts',(5.46580875850822,5.,81.8252971775594));
#40097=CARTESIAN_POINT('Ctrl Pts',(5.43155912297688,-5.,81.8402252457094));
#40098=CARTESIAN_POINT('Ctrl Pts',(5.43155912297688,5.,81.8402252457094));
#40099=CARTESIAN_POINT('Ctrl Pts',(5.39632853508549,-5.,81.8548078241758));
#40100=CARTESIAN_POINT('Ctrl Pts',(5.39632853508549,5.,81.8548078241758));
#40101=CARTESIAN_POINT('Ctrl Pts',(5.36012397677274,-5.,81.8690491154153));
#40102=CARTESIAN_POINT('Ctrl Pts',(5.36012397677274,5.,81.8690491154153));
#40103=CARTESIAN_POINT('Ctrl Pts',(5.32297992581797,-5.,81.8829304401999));
#40104=CARTESIAN_POINT('Ctrl Pts',(5.32297992581797,5.,81.8829304401999));
#40105=CARTESIAN_POINT('Ctrl Pts',(5.28494739170169,-5.,81.896418692403));
#40106=CARTESIAN_POINT('Ctrl Pts',(5.28494739170169,5.,81.896418692403));
#40107=CARTESIAN_POINT('Ctrl Pts',(5.24608497534447,-5.,81.9094733697741));
#40108=CARTESIAN_POINT('Ctrl Pts',(5.24608497534447,5.,81.9094733697741));
#40109=CARTESIAN_POINT('Ctrl Pts',(5.20645002779738,-5.,81.9220536737517));
#40110=CARTESIAN_POINT('Ctrl Pts',(5.20645002779738,5.,81.9220536737517));
#40111=CARTESIAN_POINT('Ctrl Pts',(5.16608828999526,-5.,81.934126999398));
#40112=CARTESIAN_POINT('Ctrl Pts',(5.16608828999526,5.,81.934126999398));
#40113=CARTESIAN_POINT('Ctrl Pts',(5.12503143346544,-5.,81.9456712378206));
#40114=CARTESIAN_POINT('Ctrl Pts',(5.12503143346544,5.,81.9456712378206));
#40115=CARTESIAN_POINT('Ctrl Pts',(5.08330108798129,-5.,81.956672040115));
#40116=CARTESIAN_POINT('Ctrl Pts',(5.08330108798129,5.,81.956672040115));
#40117=CARTESIAN_POINT('Ctrl Pts',(5.04091104528035,-5.,81.9671216981684));
#40118=CARTESIAN_POINT('Ctrl Pts',(5.04091104528035,5.,81.9671216981684));
#40119=CARTESIAN_POINT('Ctrl Pts',(4.99787032923518,-5.,81.9770175308375));
#40120=CARTESIAN_POINT('Ctrl Pts',(4.99787032923518,5.,81.9770175308375));
#40121=CARTESIAN_POINT('Ctrl Pts',(4.9541859211769,-5.,81.986360645658));
#40122=CARTESIAN_POINT('Ctrl Pts',(4.9541859211769,5.,81.986360645658));
#40123=CARTESIAN_POINT('Ctrl Pts',(4.90986596114179,-5.,81.9951546933809));
#40124=CARTESIAN_POINT('Ctrl Pts',(4.90986596114179,5.,81.9951546933809));
#40125=CARTESIAN_POINT('Ctrl Pts',(4.86491894851597,-5.,82.0034047666743));
#40126=CARTESIAN_POINT('Ctrl Pts',(4.86491894851597,5.,82.0034047666743));
#40127=CARTESIAN_POINT('Ctrl Pts',(4.81935277596149,-5.,82.0111163700251));
#40128=CARTESIAN_POINT('Ctrl Pts',(4.81935277596149,5.,82.0111163700251));
#40129=CARTESIAN_POINT('Ctrl Pts',(4.78240971662817,-5.,82.01685886213));
#40130=CARTESIAN_POINT('Ctrl Pts',(4.78240971662817,5.,82.01685886213));
#40131=CARTESIAN_POINT('Ctrl Pts',(4.75442870611591,-5.,82.0209272816843));
#40132=CARTESIAN_POINT('Ctrl Pts',(4.75442870611591,5.,82.0209272816843));
#40133=CARTESIAN_POINT('Ctrl Pts',(4.7356532677282,-5.,82.0235337755483));
#40134=CARTESIAN_POINT('Ctrl Pts',(4.7356532677282,5.,82.0235337755483));
#40135=CARTESIAN_POINT('Ctrl Pts',(4.72623519067131,-5.,82.0248105760097));
#40136=CARTESIAN_POINT('Ctrl Pts',(4.72623519067131,5.,82.0248105760097));
#40137=CARTESIAN_POINT('Ctrl Pts',(4.84401151007851,-4.8,82.006862464309));
#40138=CARTESIAN_POINT('Ctrl Pts',(4.84401151007851,-3.13333333333333,82.006862464309));
#40139=CARTESIAN_POINT('Ctrl Pts',(4.84401151007851,-1.46666666666667,82.006862464309));
#40140=CARTESIAN_POINT('Ctrl Pts',(4.84401151007851,1.73333333333333,82.006862464309));
#40141=CARTESIAN_POINT('Ctrl Pts',(4.84401151007851,3.26666666666667,82.0068624643091));
#40142=CARTESIAN_POINT('Ctrl Pts',(4.84401151007851,4.8,82.0068624643091));
#40143=CARTESIAN_POINT('',(5.77240469132478,0.,81.6379042610703));
#40144=CARTESIAN_POINT('Origin',(6.02846516020393,0.,81.2945453548562));
#40145=CARTESIAN_POINT('Ctrl Pts',(3.53252939109094,-5.,79.9572514818469));
#40146=CARTESIAN_POINT('Ctrl Pts',(3.53252939109094,5.,79.9572514818469));
#40147=CARTESIAN_POINT('Ctrl Pts',(3.53834417123336,-5.,79.9497335880616));
#40148=CARTESIAN_POINT('Ctrl Pts',(3.53834417123336,5.,79.9497335880616));
#40149=CARTESIAN_POINT('Ctrl Pts',(3.54998918029107,-5.,79.9347768283301));
#40150=CARTESIAN_POINT('Ctrl Pts',(3.54998918029107,5.,79.9347768283301));
#40151=CARTESIAN_POINT('Ctrl Pts',(3.56750304019465,-5.,79.9125787721238));
#40152=CARTESIAN_POINT('Ctrl Pts',(3.56750304019465,5.,79.9125787721238));
#40153=CARTESIAN_POINT('Ctrl Pts',(3.59094771388259,-5.,79.8834563902682));
#40154=CARTESIAN_POINT('Ctrl Pts',(3.59094771388259,5.,79.8834563902682));
#40155=CARTESIAN_POINT('Ctrl Pts',(3.62040924457587,-5.,79.8478507289727));
#40156=CARTESIAN_POINT('Ctrl Pts',(3.62040924457587,5.,79.8478507289727));
#40157=CARTESIAN_POINT('Ctrl Pts',(3.65002752397834,-5.,79.8130505109097));
#40158=CARTESIAN_POINT('Ctrl Pts',(3.65002752397834,5.,79.8130505109097));
#40159=CARTESIAN_POINT('Ctrl Pts',(3.67980337276931,-5.,79.7790653235472));
#40160=CARTESIAN_POINT('Ctrl Pts',(3.67980337276931,5.,79.7790653235472));
#40161=CARTESIAN_POINT('Ctrl Pts',(3.70973695162199,-5.,79.7459050738843));
#40162=CARTESIAN_POINT('Ctrl Pts',(3.70973695162199,5.,79.7459050738843));
#40163=CARTESIAN_POINT('Ctrl Pts',(3.73982735215234,-5.,79.7135786367618));
#40164=CARTESIAN_POINT('Ctrl Pts',(3.73982735215234,5.,79.7135786367618));
#40165=CARTESIAN_POINT('Ctrl Pts',(3.77007204284678,-5.,79.6820926119545));
#40166=CARTESIAN_POINT('Ctrl Pts',(3.77007204284678,5.,79.6820926119545));
#40167=CARTESIAN_POINT('Ctrl Pts',(3.80046418983303,-5.,79.6514534737968));
#40168=CARTESIAN_POINT('Ctrl Pts',(3.80046418983303,5.,79.6514534737968));
#40169=CARTESIAN_POINT('Ctrl Pts',(3.83099022182597,-5.,79.6216693122348));
#40170=CARTESIAN_POINT('Ctrl Pts',(3.83099022182597,5.,79.6216693122348));
#40171=CARTESIAN_POINT('Ctrl Pts',(3.86162689742956,-5.,79.5927516847587));
#40172=CARTESIAN_POINT('Ctrl Pts',(3.86162689742956,5.,79.5927516847587));
#40173=CARTESIAN_POINT('Ctrl Pts',(3.89233923402316,-5.,79.5647169652776));
#40174=CARTESIAN_POINT('Ctrl Pts',(3.89233923402316,5.,79.5647169652776));
#40175=CARTESIAN_POINT('Ctrl Pts',(3.92307612443792,-5.,79.5375884641383));
#40176=CARTESIAN_POINT('Ctrl Pts',(3.92307612443792,5.,79.5375884641383));
#40177=CARTESIAN_POINT('Ctrl Pts',(3.95377356055667,-5.,79.5113954495259));
#40178=CARTESIAN_POINT('Ctrl Pts',(3.95377356055667,5.,79.5113954495259));
#40179=CARTESIAN_POINT('Ctrl Pts',(3.9843671659396,-5.,79.4861684201978));
#40180=CARTESIAN_POINT('Ctrl Pts',(3.9843671659396,5.,79.4861684201978));
#40181=CARTESIAN_POINT('Ctrl Pts',(4.01480276509681,-5.,79.4619349985923));
#40182=CARTESIAN_POINT('Ctrl Pts',(4.01480276509681,5.,79.4619349985923));
#40183=CARTESIAN_POINT('Ctrl Pts',(4.04504694245072,-5.,79.4387157037247));
#40184=CARTESIAN_POINT('Ctrl Pts',(4.04504694245072,5.,79.4387157037247));
#40185=CARTESIAN_POINT('Ctrl Pts',(4.07509984646481,-5.,79.4165186833579));
#40186=CARTESIAN_POINT('Ctrl Pts',(4.07509984646481,5.,79.4165186833579));
#40187=CARTESIAN_POINT('Ctrl Pts',(4.10500125173415,-5.,79.3953370081669));
#40188=CARTESIAN_POINT('Ctrl Pts',(4.10500125173415,5.,79.3953370081669));
#40189=CARTESIAN_POINT('Ctrl Pts',(4.13479151474939,-5.,79.3751639066383));
#40190=CARTESIAN_POINT('Ctrl Pts',(4.13479151474939,5.,79.3751639066383));
#40191=CARTESIAN_POINT('Ctrl Pts',(4.16447616102922,-5.,79.3560063825947));
#40192=CARTESIAN_POINT('Ctrl Pts',(4.16447616102922,5.,79.3560063825947));
#40193=CARTESIAN_POINT('Ctrl Pts',(4.19399149688981,-5.,79.3378983123566));
#40194=CARTESIAN_POINT('Ctrl Pts',(4.19399149688981,5.,79.3378983123566));
#40195=CARTESIAN_POINT('Ctrl Pts',(4.22316329868624,-5.,79.3209160650712));
#40196=CARTESIAN_POINT('Ctrl Pts',(4.22316329868624,5.,79.3209160650712));
#40197=CARTESIAN_POINT('Ctrl Pts',(4.25168596944548,-5.,79.3051860439254));
#40198=CARTESIAN_POINT('Ctrl Pts',(4.25168596944548,5.,79.3051860439254));
#40199=CARTESIAN_POINT('Ctrl Pts',(4.27919110463568,-5.,79.290857572383));
#40200=CARTESIAN_POINT('Ctrl Pts',(4.27919110463568,5.,79.290857572383));
#40201=CARTESIAN_POINT('Ctrl Pts',(4.30530568630548,-5.,79.2780795061304));
#40202=CARTESIAN_POINT('Ctrl Pts',(4.30530568630548,5.,79.2780795061304));
#40203=CARTESIAN_POINT('Ctrl Pts',(4.32970884225655,-5.,79.2669775144253));
#40204=CARTESIAN_POINT('Ctrl Pts',(4.32970884225655,5.,79.2669775144253));
#40205=CARTESIAN_POINT('Ctrl Pts',(4.35220362546771,-5.,79.2576246716733));
#40206=CARTESIAN_POINT('Ctrl Pts',(4.35220362546771,5.,79.2576246716733));
#40207=CARTESIAN_POINT('Ctrl Pts',(4.36860399348142,-5.,79.2515635749137));
#40208=CARTESIAN_POINT('Ctrl Pts',(4.36860399348142,5.,79.2515635749137));
#40209=CARTESIAN_POINT('Ctrl Pts',(4.37999667111292,-5.,79.2478185812853));
#40210=CARTESIAN_POINT('Ctrl Pts',(4.37999667111292,5.,79.2478185812853));
#40211=CARTESIAN_POINT('Ctrl Pts',(4.3871892149765,-5.,79.2456771677804));
#40212=CARTESIAN_POINT('Ctrl Pts',(4.3871892149765,5.,79.2456771677804));
#40213=CARTESIAN_POINT('Ctrl Pts',(4.39068483903982,-5.,79.2446952750862));
#40214=CARTESIAN_POINT('Ctrl Pts',(4.39068483903982,5.,79.2446952750862));
#40215=CARTESIAN_POINT('',(4.39068483903982,0.,79.2446952750862));
#40216=CARTESIAN_POINT('Ctrl Pts',(3.60696107140889,4.8,79.864228252917));
#40217=CARTESIAN_POINT('Ctrl Pts',(3.60696107140889,3.13333333333333,79.864228252917));
#40218=CARTESIAN_POINT('Ctrl Pts',(3.60696107140889,1.46666666666667,79.864228252917));
#40219=CARTESIAN_POINT('Ctrl Pts',(3.60696107140889,-1.73333333333333,79.864228252917));
#40220=CARTESIAN_POINT('Ctrl Pts',(3.60696107140887,-3.26666666666667,79.8642282529171));
#40221=CARTESIAN_POINT('Ctrl Pts',(3.60696107140887,-4.8,79.8642282529171));
#40222=CARTESIAN_POINT('Origin',(9.31000000000016,0.,78.));
#40223=CARTESIAN_POINT('',(4.67850553742098,0.,78.4144382259154));
#40224=CARTESIAN_POINT('',(4.81607260887647,0.,79.194619857239));
#40225=CARTESIAN_POINT('Origin',(4.39068483903982,0.,79.2446952750862));
#40226=CARTESIAN_POINT('Ctrl Pts',(4.2616449875437,-5.,78.5128739112901));
#40227=CARTESIAN_POINT('Ctrl Pts',(4.2616449875437,5.,78.5128739112901));
#40228=CARTESIAN_POINT('Ctrl Pts',(4.25802434832344,-5.,78.5131468077951));
#40229=CARTESIAN_POINT('Ctrl Pts',(4.25802434832344,5.,78.5131468077951));
#40230=CARTESIAN_POINT('Ctrl Pts',(4.25053316137154,-5.,78.5135945321785));
#40231=CARTESIAN_POINT('Ctrl Pts',(4.25053316137154,5.,78.5135945321785));
#40232=CARTESIAN_POINT('Ctrl Pts',(4.23854668300885,-5.,78.5139719145122));
#40233=CARTESIAN_POINT('Ctrl Pts',(4.23854668300885,5.,78.5139719145122));
#40234=CARTESIAN_POINT('Ctrl Pts',(4.22106236102646,-5.,78.5138856028362));
#40235=CARTESIAN_POINT('Ctrl Pts',(4.22106236102646,5.,78.5138856028362));
#40236=CARTESIAN_POINT('Ctrl Pts',(4.19672531862463,-5.,78.5127904745385));
#40237=CARTESIAN_POINT('Ctrl Pts',(4.19672531862463,5.,78.5127904745385));
#40238=CARTESIAN_POINT('Ctrl Pts',(4.16999674826607,-5.,78.510704385798));
#40239=CARTESIAN_POINT('Ctrl Pts',(4.16999674826607,5.,78.510704385798));
#40240=CARTESIAN_POINT('Ctrl Pts',(4.14108671252852,-5.,78.5076286442226));
#40241=CARTESIAN_POINT('Ctrl Pts',(4.14108671252852,5.,78.5076286442226));
#40242=CARTESIAN_POINT('Ctrl Pts',(4.110339714066,-5.,78.5035715955273));
#40243=CARTESIAN_POINT('Ctrl Pts',(4.110339714066,5.,78.5035715955273));
#40244=CARTESIAN_POINT('Ctrl Pts',(4.07815718673905,-5.,78.4985455386556));
#40245=CARTESIAN_POINT('Ctrl Pts',(4.07815718673905,5.,78.4985455386556));
#40246=CARTESIAN_POINT('Ctrl Pts',(4.04493638920224,-5.,78.4925647900071));
#40247=CARTESIAN_POINT('Ctrl Pts',(4.04493638920224,5.,78.4925647900071));
#40248=CARTESIAN_POINT('Ctrl Pts',(4.01100772111375,-5.,78.4856436094149));
#40249=CARTESIAN_POINT('Ctrl Pts',(4.01100772111375,5.,78.4856436094149));
#40250=CARTESIAN_POINT('Ctrl Pts',(3.97656101893434,-5.,78.477794172411));
#40251=CARTESIAN_POINT('Ctrl Pts',(3.97656101893434,5.,78.477794172411));
#40252=CARTESIAN_POINT('Ctrl Pts',(3.94166772153227,-5.,78.4690265277979));
#40253=CARTESIAN_POINT('Ctrl Pts',(3.94166772153227,5.,78.4690265277979));
#40254=CARTESIAN_POINT('Ctrl Pts',(3.906325032066,-5.,78.4593491468487));
#40255=CARTESIAN_POINT('Ctrl Pts',(3.906325032066,5.,78.4593491468487));
#40256=CARTESIAN_POINT('Ctrl Pts',(3.87049271184418,-5.,78.448769469149));
#40257=CARTESIAN_POINT('Ctrl Pts',(3.87049271184418,5.,78.448769469149));
#40258=CARTESIAN_POINT('Ctrl Pts',(3.83413101500406,-5.,78.4372945869717));
#40259=CARTESIAN_POINT('Ctrl Pts',(3.83413101500406,5.,78.4372945869717));
#40260=CARTESIAN_POINT('Ctrl Pts',(3.79724258873491,-5.,78.4249322074894));
#40261=CARTESIAN_POINT('Ctrl Pts',(3.79724258873491,5.,78.4249322074894));
#40262=CARTESIAN_POINT('Ctrl Pts',(3.75986585132571,-5.,78.4116901834742));
#40263=CARTESIAN_POINT('Ctrl Pts',(3.75986585132571,5.,78.4116901834742));
#40264=CARTESIAN_POINT('Ctrl Pts',(3.72206115851568,-5.,78.3975759424256));
#40265=CARTESIAN_POINT('Ctrl Pts',(3.72206115851568,5.,78.3975759424256));
#40266=CARTESIAN_POINT('Ctrl Pts',(3.68389943556036,-5.,78.3825961257671));
#40267=CARTESIAN_POINT('Ctrl Pts',(3.68389943556036,5.,78.3825961257671));
#40268=CARTESIAN_POINT('Ctrl Pts',(3.64545084072423,-5.,78.3667563445328));
#40269=CARTESIAN_POINT('Ctrl Pts',(3.64545084072423,5.,78.3667563445328));
#40270=CARTESIAN_POINT('Ctrl Pts',(3.60677137164415,-5.,78.3500610235961));
#40271=CARTESIAN_POINT('Ctrl Pts',(3.60677137164415,5.,78.3500610235961));
#40272=CARTESIAN_POINT('Ctrl Pts',(3.56789950143576,-5.,78.3325135846256));
#40273=CARTESIAN_POINT('Ctrl Pts',(3.56789950143576,5.,78.3325135846256));
#40274=CARTESIAN_POINT('Ctrl Pts',(3.52886102276017,-5.,78.31411693907));
#40275=CARTESIAN_POINT('Ctrl Pts',(3.52886102276017,5.,78.31411693907));
#40276=CARTESIAN_POINT('Ctrl Pts',(3.48967145537698,-5.,78.2948740473282));
#40277=CARTESIAN_POINT('Ctrl Pts',(3.48967145537698,5.,78.2948740473282));
#40278=CARTESIAN_POINT('Ctrl Pts',(3.45033943537775,-5.,78.2747886559578));
#40279=CARTESIAN_POINT('Ctrl Pts',(3.45033943537775,5.,78.2747886559578));
#40280=CARTESIAN_POINT('Ctrl Pts',(3.41086959886365,-5.,78.2538661008949));
#40281=CARTESIAN_POINT('Ctrl Pts',(3.41086959886365,5.,78.2538661008949));
#40282=CARTESIAN_POINT('Ctrl Pts',(3.37126583481318,-5.,78.2321144110957));
#40283=CARTESIAN_POINT('Ctrl Pts',(3.37126583481318,5.,78.2321144110957));
#40284=CARTESIAN_POINT('Ctrl Pts',(3.33153138063971,-5.,78.2095429510755));
#40285=CARTESIAN_POINT('Ctrl Pts',(3.33153138063971,5.,78.2095429510755));
#40286=CARTESIAN_POINT('Ctrl Pts',(3.29166874426803,-5.,78.1861610108276));
#40287=CARTESIAN_POINT('Ctrl Pts',(3.29166874426803,5.,78.1861610108276));
#40288=CARTESIAN_POINT('Ctrl Pts',(3.25967751619637,-5.,78.1668134742004));
#40289=CARTESIAN_POINT('Ctrl Pts',(3.25967751619637,5.,78.1668134742004));
#40290=CARTESIAN_POINT('Ctrl Pts',(3.23562768892866,-5.,78.1519442175444));
#40291=CARTESIAN_POINT('Ctrl Pts',(3.23562768892866,5.,78.1519442175444));
#40292=CARTESIAN_POINT('Ctrl Pts',(3.21956944675078,-5.,78.1418722885375));
#40293=CARTESIAN_POINT('Ctrl Pts',(3.21956944675078,5.,78.1418722885375));
#40294=CARTESIAN_POINT('Ctrl Pts',(3.21153406965502,-5.,78.1367965512051));
#40295=CARTESIAN_POINT('Ctrl Pts',(3.21153406965502,5.,78.1367965512051));
#40296=CARTESIAN_POINT('Ctrl Pts',(3.31329278848646,-4.8,78.1987526588035));
#40297=CARTESIAN_POINT('Ctrl Pts',(3.31329278848646,-3.13333333333333,78.1987526588035));
#40298=CARTESIAN_POINT('Ctrl Pts',(3.31329278848646,-1.46666666666667,78.1987526588035));
#40299=CARTESIAN_POINT('Ctrl Pts',(3.31329278848646,1.73333333333333,78.1987526588035));
#40300=CARTESIAN_POINT('Ctrl Pts',(3.31329278848646,3.26666666666667,78.1987526588035));
#40301=CARTESIAN_POINT('Ctrl Pts',(3.31329278848646,4.8,78.1987526588035));
#40302=CARTESIAN_POINT('',(4.2616449875437,0.,78.5128739112901));
#40303=CARTESIAN_POINT('Origin',(4.67850553742098,0.,78.4144382259154));
#40304=CARTESIAN_POINT('Origin',(9.31,0.,78.));
#40305=CARTESIAN_POINT('Origin',(9.31,0.,78.));
#40306=CARTESIAN_POINT('Origin',(9.31,0.,78.));
#40307=CARTESIAN_POINT('Origin',(9.31,0.,78.));
#40308=CARTESIAN_POINT('Origin',(9.31,0.,78.));
#40309=CARTESIAN_POINT('Origin',(9.31,0.,78.));
#40310=CARTESIAN_POINT('Origin',(9.31,0.,78.));
#40311=CARTESIAN_POINT('Origin',(9.31,0.,78.));
#40312=CARTESIAN_POINT('Origin',(9.31,0.,78.));
#40313=CARTESIAN_POINT('Origin',(9.31,0.,78.));
#40314=CARTESIAN_POINT('Origin',(9.31,0.,78.));
#40315=CARTESIAN_POINT('Origin',(9.31,0.,78.));
#40316=CARTESIAN_POINT('Origin',(9.31,0.,78.));
#40317=CARTESIAN_POINT('Origin',(9.31,0.,78.));
#40318=CARTESIAN_POINT('Origin',(9.31,0.,78.));
#40319=CARTESIAN_POINT('Origin',(9.31,0.,78.));
#40320=CARTESIAN_POINT('Origin',(9.31,0.,78.));
#40321=CARTESIAN_POINT('Origin',(9.31,0.,78.));
#70725=UNCERTAINTY_MEASURE_WITH_UNIT(LENGTH_MEASURE(0.001),#70758,
'DISTANCE_ACCURACY_VALUE',
'Maximum model space distance between geometric entities at asserted c
onnectivities');
#70740=UNCERTAINTY_MEASURE_WITH_UNIT(LENGTH_MEASURE(0.001),#70758,
'DISTANCE_ACCURACY_VALUE',
'Maximum model space distance between geometric entities at asserted c
onnectivities');
#70742=(
GEOMETRIC_REPRESENTATION_CONTEXT(3)
GLOBAL_UNCERTAINTY_ASSIGNED_CONTEXT((#70725))
GLOBAL_UNIT_ASSIGNED_CONTEXT((#70758,#70760,#70761))
REPRESENTATION_CONTEXT('','3D')
);
#70757=(
GEOMETRIC_REPRESENTATION_CONTEXT(3)
GLOBAL_UNCERTAINTY_ASSIGNED_CONTEXT((#70740))
GLOBAL_UNIT_ASSIGNED_CONTEXT((#70758,#70760,#70761))
REPRESENTATION_CONTEXT('','3D')
);
#70758=(
LENGTH_UNIT()
NAMED_UNIT(*)
SI_UNIT(.CENTI.,.METRE.)
);
#70760=(
NAMED_UNIT(*)
PLANE_ANGLE_UNIT()
SI_UNIT($,.RADIAN.)
);
#70761=(
NAMED_UNIT(*)
SI_UNIT($,.STERADIAN.)
SOLID_ANGLE_UNIT()
);
#70763=SHAPE_DEFINITION_REPRESENTATION(#70779,#70818);
#70779=PRODUCT_DEFINITION_SHAPE('',$,#70835);
#70818=SHAPE_REPRESENTATION('',(#27054),#70742);
#70833=PRODUCT_DEFINITION_CONTEXT('part definition',#70883,'design');
#70835=PRODUCT_DEFINITION('2026-10-19-02-54-55-610',
'03_Pinion_Shaft_m6_z18_D125_Journals',#70851,#70833);
#70851=PRODUCT_DEFINITION_FORMATION('',$,#70886);
#70883=APPLICATION_CONTEXT(
'Core Data for Automotive Mechanical Design Process');
#70884=PRODUCT_CONTEXT('part definition',#70883,'mechanical');
#70886=PRODUCT('2026-10-19-02-54-55-610',
'03_Pinion_Shaft_m6_z18_D125_Journals',$,(#70884));
#71041=COLOUR_RGB('Grey',0.48,0.52,0.57);
#71042=FILL_AREA_STYLE_COLOUR('',#71041);
#71043=FILL_AREA_STYLE('',(#71042));
#71044=SURFACE_STYLE_FILL_AREA(#71043);
#71045=SURFACE_SIDE_STYLE('',(#71044));
#71046=SURFACE_STYLE_USAGE(.BOTH.,#71045);
#71047=PRESENTATION_STYLE_ASSIGNMENT((#71046));
ENDSEC;
END-ISO-10303-21;
